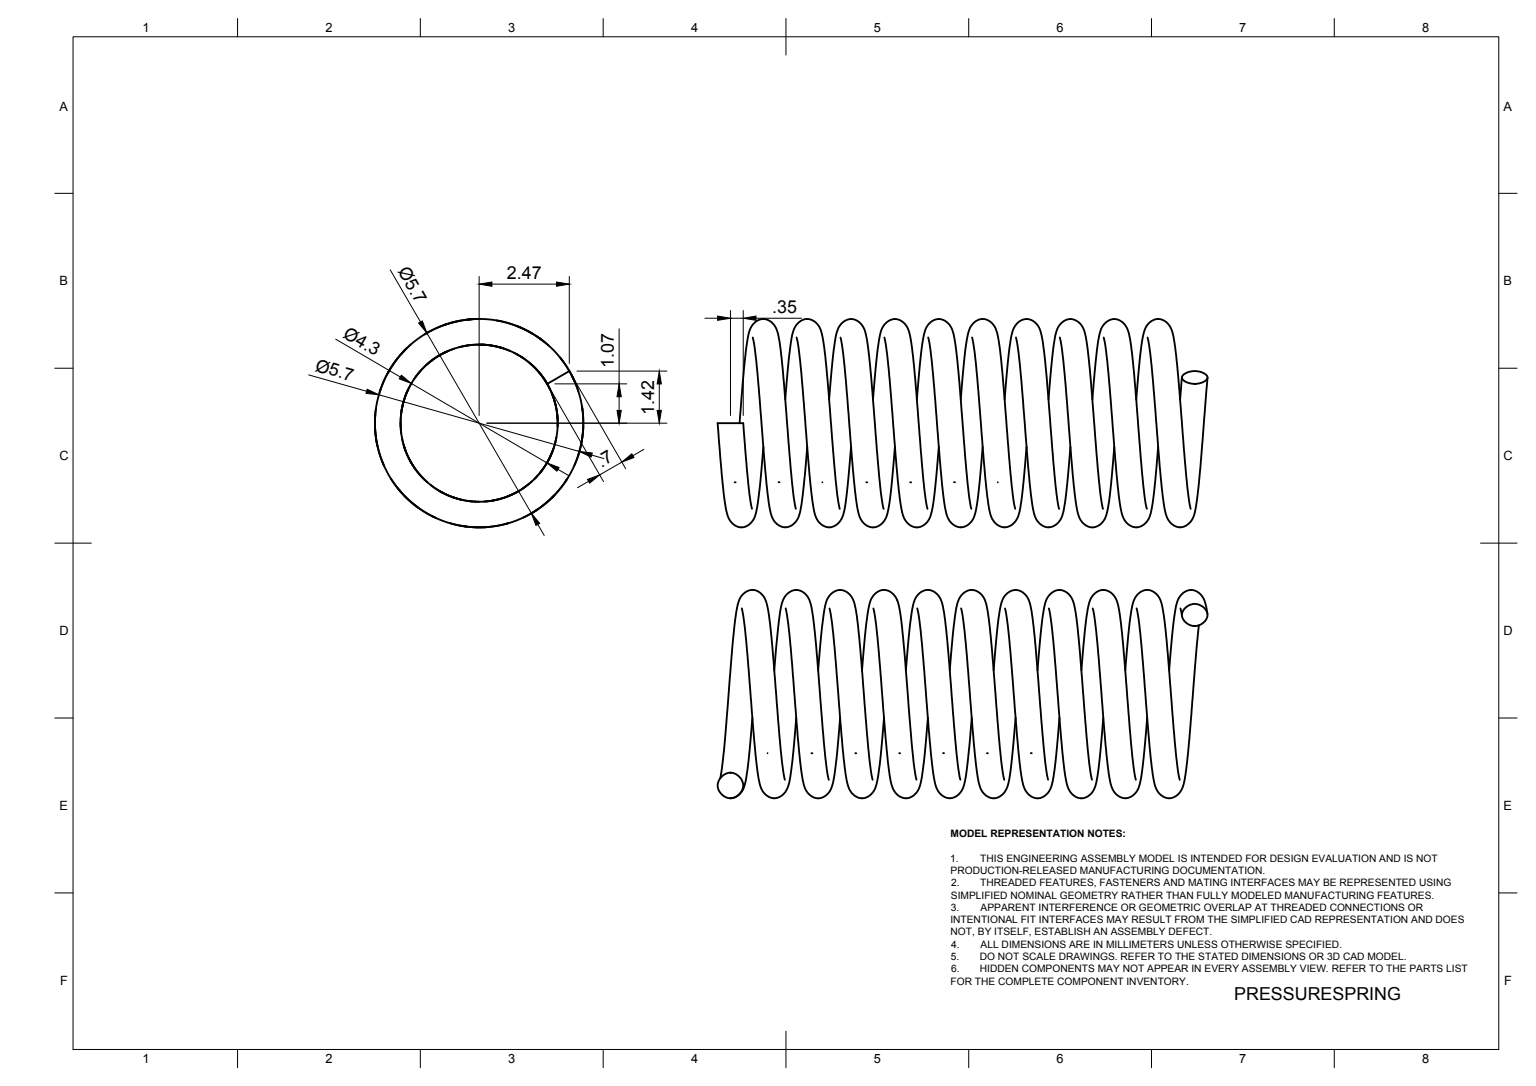
ISO-10303-21;
HEADER;
/* Generated by software containing ST-Developer
 * from STEP Tools, Inc. (www.steptools.com) 
 */

FILE_DESCRIPTION(
/* description */ (''),
/* implementation_level */ '2;1');

FILE_NAME(
/* name */ 'PRESSURESPRING.step',
/* time_stamp */ '2026-10-06T01:16:10-07:00',
/* author */ (''),
/* organization */ (''),
/* preprocessor_version */ 'ST-DEVELOPER v20.2',
/* originating_system */ 'Autodesk Translation Framework v15.15.0.0',
/* authorisation */ '');

FILE_SCHEMA (('AUTOMOTIVE_DESIGN { 1 0 10303 214 3 1 1 }'));
ENDSEC;

DATA;
#10=MECHANICAL_DESIGN_GEOMETRIC_PRESENTATION_REPRESENTATION('',(#319),#17113);
#11=B_SPLINE_SURFACE_WITH_KNOTS('',3,3,((#11570,#11571,#11572,#11573,#11574,
#11575,#11576,#11577,#11578,#11579,#11580,#11581,#11582,#11583,#11584,#11585,
#11586,#11587,#11588,#11589,#11590,#11591,#11592,#11593,#11594,#11595,#11596,
#11597,#11598,#11599,#11600,#11601,#11602,#11603,#11604),(#11605,#11606,
#11607,#11608,#11609,#11610,#11611,#11612,#11613,#11614,#11615,#11616,#11617,
#11618,#11619,#11620,#11621,#11622,#11623,#11624,#11625,#11626,#11627,#11628,
#11629,#11630,#11631,#11632,#11633,#11634,#11635,#11636,#11637,#11638,#11639),
(#11640,#11641,#11642,#11643,#11644,#11645,#11646,#11647,#11648,#11649,
#11650,#11651,#11652,#11653,#11654,#11655,#11656,#11657,#11658,#11659,#11660,
#11661,#11662,#11663,#11664,#11665,#11666,#11667,#11668,#11669,#11670,#11671,
#11672,#11673,#11674),(#11675,#11676,#11677,#11678,#11679,#11680,#11681,
#11682,#11683,#11684,#11685,#11686,#11687,#11688,#11689,#11690,#11691,#11692,
#11693,#11694,#11695,#11696,#11697,#11698,#11699,#11700,#11701,#11702,#11703,
#11704,#11705,#11706,#11707,#11708,#11709),(#11710,#11711,#11712,#11713,
#11714,#11715,#11716,#11717,#11718,#11719,#11720,#11721,#11722,#11723,#11724,
#11725,#11726,#11727,#11728,#11729,#11730,#11731,#11732,#11733,#11734,#11735,
#11736,#11737,#11738,#11739,#11740,#11741,#11742,#11743,#11744),(#11745,
#11746,#11747,#11748,#11749,#11750,#11751,#11752,#11753,#11754,#11755,#11756,
#11757,#11758,#11759,#11760,#11761,#11762,#11763,#11764,#11765,#11766,#11767,
#11768,#11769,#11770,#11771,#11772,#11773,#11774,#11775,#11776,#11777,#11778,
#11779),(#11780,#11781,#11782,#11783,#11784,#11785,#11786,#11787,#11788,
#11789,#11790,#11791,#11792,#11793,#11794,#11795,#11796,#11797,#11798,#11799,
#11800,#11801,#11802,#11803,#11804,#11805,#11806,#11807,#11808,#11809,#11810,
#11811,#11812,#11813,#11814),(#11815,#11816,#11817,#11818,#11819,#11820,
#11821,#11822,#11823,#11824,#11825,#11826,#11827,#11828,#11829,#11830,#11831,
#11832,#11833,#11834,#11835,#11836,#11837,#11838,#11839,#11840,#11841,#11842,
#11843,#11844,#11845,#11846,#11847,#11848,#11849),(#11850,#11851,#11852,
#11853,#11854,#11855,#11856,#11857,#11858,#11859,#11860,#11861,#11862,#11863,
#11864,#11865,#11866,#11867,#11868,#11869,#11870,#11871,#11872,#11873,#11874,
#11875,#11876,#11877,#11878,#11879,#11880,#11881,#11882,#11883,#11884),
(#11885,#11886,#11887,#11888,#11889,#11890,#11891,#11892,#11893,#11894,
#11895,#11896,#11897,#11898,#11899,#11900,#11901,#11902,#11903,#11904,#11905,
#11906,#11907,#11908,#11909,#11910,#11911,#11912,#11913,#11914,#11915,#11916,
#11917,#11918,#11919)),.UNSPECIFIED.,.F.,.F.,.F.,(4,1,1,1,1,1,1,4),(4,1,
1,1,1,1,1,1,1,1,1,1,1,1,1,1,1,1,1,1,1,1,1,1,1,1,1,1,1,1,1,1,4),(-0.05714514294858,
0.,0.125,0.25,0.3267862857371,0.4035725714743,0.4803588572114,0.5571451429486),
(-0.02,0.0125,0.045,0.0775,0.11,0.1425,0.175,0.2075,0.24,0.2725,0.305,0.3375,
0.37,0.4025,0.435,0.4675,0.5,0.5325,0.565,0.5975,0.63,0.6625,0.695,0.7275,
0.76,0.7925,0.825,0.8575,0.89,0.9225,0.955,0.9875,1.02),.UNSPECIFIED.);
#12=B_SPLINE_SURFACE_WITH_KNOTS('',3,3,((#13047,#13048,#13049,#13050,#13051,
#13052,#13053,#13054,#13055,#13056,#13057,#13058,#13059,#13060,#13061,#13062,
#13063,#13064,#13065,#13066,#13067,#13068,#13069,#13070,#13071,#13072,#13073,
#13074,#13075,#13076,#13077,#13078,#13079,#13080,#13081),(#13082,#13083,
#13084,#13085,#13086,#13087,#13088,#13089,#13090,#13091,#13092,#13093,#13094,
#13095,#13096,#13097,#13098,#13099,#13100,#13101,#13102,#13103,#13104,#13105,
#13106,#13107,#13108,#13109,#13110,#13111,#13112,#13113,#13114,#13115,#13116),
(#13117,#13118,#13119,#13120,#13121,#13122,#13123,#13124,#13125,#13126,
#13127,#13128,#13129,#13130,#13131,#13132,#13133,#13134,#13135,#13136,#13137,
#13138,#13139,#13140,#13141,#13142,#13143,#13144,#13145,#13146,#13147,#13148,
#13149,#13150,#13151),(#13152,#13153,#13154,#13155,#13156,#13157,#13158,
#13159,#13160,#13161,#13162,#13163,#13164,#13165,#13166,#13167,#13168,#13169,
#13170,#13171,#13172,#13173,#13174,#13175,#13176,#13177,#13178,#13179,#13180,
#13181,#13182,#13183,#13184,#13185,#13186),(#13187,#13188,#13189,#13190,
#13191,#13192,#13193,#13194,#13195,#13196,#13197,#13198,#13199,#13200,#13201,
#13202,#13203,#13204,#13205,#13206,#13207,#13208,#13209,#13210,#13211,#13212,
#13213,#13214,#13215,#13216,#13217,#13218,#13219,#13220,#13221),(#13222,
#13223,#13224,#13225,#13226,#13227,#13228,#13229,#13230,#13231,#13232,#13233,
#13234,#13235,#13236,#13237,#13238,#13239,#13240,#13241,#13242,#13243,#13244,
#13245,#13246,#13247,#13248,#13249,#13250,#13251,#13252,#13253,#13254,#13255,
#13256),(#13257,#13258,#13259,#13260,#13261,#13262,#13263,#13264,#13265,
#13266,#13267,#13268,#13269,#13270,#13271,#13272,#13273,#13274,#13275,#13276,
#13277,#13278,#13279,#13280,#13281,#13282,#13283,#13284,#13285,#13286,#13287,
#13288,#13289,#13290,#13291)),.UNSPECIFIED.,.F.,.F.,.F.,(4,1,1,1,4),(4,
1,1,1,1,1,1,1,1,1,1,1,1,1,1,1,1,1,1,1,1,1,1,1,1,1,1,1,1,1,1,1,4),(0.4428548570514,
0.5,0.75,1.,1.057145142949),(-0.02,0.0125,0.045,0.0775,0.11,0.1425,0.175,
0.2075,0.24,0.2725,0.305,0.3375,0.37,0.4025,0.435,0.4675,0.5,0.5325,0.565,
0.5975,0.63,0.6625,0.695,0.7275,0.76,0.7925,0.825,0.8575,0.89,0.9225,0.955,
0.9875,1.02),.UNSPECIFIED.);
#13=B_SPLINE_SURFACE_WITH_KNOTS('',3,3,((#13335,#13336,#13337,#13338,#13339,
#13340,#13341,#13342,#13343,#13344,#13345,#13346,#13347,#13348,#13349,#13350,
#13351,#13352,#13353,#13354,#13355,#13356,#13357,#13358,#13359,#13360,#13361,
#13362,#13363,#13364,#13365,#13366,#13367,#13368,#13369),(#13370,#13371,
#13372,#13373,#13374,#13375,#13376,#13377,#13378,#13379,#13380,#13381,#13382,
#13383,#13384,#13385,#13386,#13387,#13388,#13389,#13390,#13391,#13392,#13393,
#13394,#13395,#13396,#13397,#13398,#13399,#13400,#13401,#13402,#13403,#13404),
(#13405,#13406,#13407,#13408,#13409,#13410,#13411,#13412,#13413,#13414,
#13415,#13416,#13417,#13418,#13419,#13420,#13421,#13422,#13423,#13424,#13425,
#13426,#13427,#13428,#13429,#13430,#13431,#13432,#13433,#13434,#13435,#13436,
#13437,#13438,#13439),(#13440,#13441,#13442,#13443,#13444,#13445,#13446,
#13447,#13448,#13449,#13450,#13451,#13452,#13453,#13454,#13455,#13456,#13457,
#13458,#13459,#13460,#13461,#13462,#13463,#13464,#13465,#13466,#13467,#13468,
#13469,#13470,#13471,#13472,#13473,#13474),(#13475,#13476,#13477,#13478,
#13479,#13480,#13481,#13482,#13483,#13484,#13485,#13486,#13487,#13488,#13489,
#13490,#13491,#13492,#13493,#13494,#13495,#13496,#13497,#13498,#13499,#13500,
#13501,#13502,#13503,#13504,#13505,#13506,#13507,#13508,#13509),(#13510,
#13511,#13512,#13513,#13514,#13515,#13516,#13517,#13518,#13519,#13520,#13521,
#13522,#13523,#13524,#13525,#13526,#13527,#13528,#13529,#13530,#13531,#13532,
#13533,#13534,#13535,#13536,#13537,#13538,#13539,#13540,#13541,#13542,#13543,
#13544),(#13545,#13546,#13547,#13548,#13549,#13550,#13551,#13552,#13553,
#13554,#13555,#13556,#13557,#13558,#13559,#13560,#13561,#13562,#13563,#13564,
#13565,#13566,#13567,#13568,#13569,#13570,#13571,#13572,#13573,#13574,#13575,
#13576,#13577,#13578,#13579)),.UNSPECIFIED.,.F.,.F.,.F.,(4,1,1,1,4),(4,
1,1,1,1,1,1,1,1,1,1,1,1,1,1,1,1,1,1,1,1,1,1,1,1,1,1,1,1,1,1,1,4),(0.4428548570514,
0.5,0.75,1.,1.057145142949),(-0.02,0.0125,0.045,0.0775,0.11,0.1425,0.175,
0.2075,0.24,0.2725,0.305,0.3375,0.37,0.4025,0.435,0.4675,0.5,0.5325,0.565,
0.5975,0.63,0.6625,0.695,0.7275,0.76,0.7925,0.825,0.8575,0.89,0.9225,0.955,
0.9875,1.02),.UNSPECIFIED.);
#14=B_SPLINE_SURFACE_WITH_KNOTS('',3,3,((#14695,#14696,#14697,#14698,#14699,
#14700,#14701,#14702,#14703,#14704,#14705,#14706,#14707,#14708,#14709,#14710,
#14711,#14712,#14713,#14714,#14715,#14716,#14717,#14718,#14719,#14720,#14721,
#14722,#14723,#14724,#14725,#14726,#14727,#14728,#14729),(#14730,#14731,
#14732,#14733,#14734,#14735,#14736,#14737,#14738,#14739,#14740,#14741,#14742,
#14743,#14744,#14745,#14746,#14747,#14748,#14749,#14750,#14751,#14752,#14753,
#14754,#14755,#14756,#14757,#14758,#14759,#14760,#14761,#14762,#14763,#14764),
(#14765,#14766,#14767,#14768,#14769,#14770,#14771,#14772,#14773,#14774,
#14775,#14776,#14777,#14778,#14779,#14780,#14781,#14782,#14783,#14784,#14785,
#14786,#14787,#14788,#14789,#14790,#14791,#14792,#14793,#14794,#14795,#14796,
#14797,#14798,#14799),(#14800,#14801,#14802,#14803,#14804,#14805,#14806,
#14807,#14808,#14809,#14810,#14811,#14812,#14813,#14814,#14815,#14816,#14817,
#14818,#14819,#14820,#14821,#14822,#14823,#14824,#14825,#14826,#14827,#14828,
#14829,#14830,#14831,#14832,#14833,#14834),(#14835,#14836,#14837,#14838,
#14839,#14840,#14841,#14842,#14843,#14844,#14845,#14846,#14847,#14848,#14849,
#14850,#14851,#14852,#14853,#14854,#14855,#14856,#14857,#14858,#14859,#14860,
#14861,#14862,#14863,#14864,#14865,#14866,#14867,#14868,#14869),(#14870,
#14871,#14872,#14873,#14874,#14875,#14876,#14877,#14878,#14879,#14880,#14881,
#14882,#14883,#14884,#14885,#14886,#14887,#14888,#14889,#14890,#14891,#14892,
#14893,#14894,#14895,#14896,#14897,#14898,#14899,#14900,#14901,#14902,#14903,
#14904),(#14905,#14906,#14907,#14908,#14909,#14910,#14911,#14912,#14913,
#14914,#14915,#14916,#14917,#14918,#14919,#14920,#14921,#14922,#14923,#14924,
#14925,#14926,#14927,#14928,#14929,#14930,#14931,#14932,#14933,#14934,#14935,
#14936,#14937,#14938,#14939),(#14940,#14941,#14942,#14943,#14944,#14945,
#14946,#14947,#14948,#14949,#14950,#14951,#14952,#14953,#14954,#14955,#14956,
#14957,#14958,#14959,#14960,#14961,#14962,#14963,#14964,#14965,#14966,#14967,
#14968,#14969,#14970,#14971,#14972,#14973,#14974),(#14975,#14976,#14977,
#14978,#14979,#14980,#14981,#14982,#14983,#14984,#14985,#14986,#14987,#14988,
#14989,#14990,#14991,#14992,#14993,#14994,#14995,#14996,#14997,#14998,#14999,
#15000,#15001,#15002,#15003,#15004,#15005,#15006,#15007,#15008,#15009),
(#15010,#15011,#15012,#15013,#15014,#15015,#15016,#15017,#15018,#15019,
#15020,#15021,#15022,#15023,#15024,#15025,#15026,#15027,#15028,#15029,#15030,
#15031,#15032,#15033,#15034,#15035,#15036,#15037,#15038,#15039,#15040,#15041,
#15042,#15043,#15044)),.UNSPECIFIED.,.F.,.F.,.F.,(4,1,1,1,1,1,1,4),(4,1,
1,1,1,1,1,1,1,1,1,1,1,1,1,1,1,1,1,1,1,1,1,1,1,1,1,1,1,1,1,1,4),(-0.05714514294857,
0.,0.125,0.25,0.3267862857371,0.4035725714743,0.4803588572114,0.5571451429486),
(-0.02,0.0125,0.045,0.0775,0.11,0.1425,0.175,0.2075,0.24,0.2725,0.305,0.3375,
0.37,0.4025,0.435,0.4675,0.5,0.5325,0.565,0.5975,0.63,0.6625,0.695,0.7275,
0.76,0.7925,0.825,0.8575,0.89,0.9225,0.955,0.9875,1.02),.UNSPECIFIED.);
#15=B_SPLINE_SURFACE_WITH_KNOTS('',3,3,((#15100,#15101,#15102,#15103,#15104,
#15105,#15106,#15107,#15108,#15109,#15110,#15111,#15112,#15113,#15114,#15115,
#15116,#15117,#15118,#15119,#15120,#15121,#15122,#15123,#15124,#15125,#15126,
#15127,#15128,#15129,#15130,#15131,#15132,#15133,#15134),(#15135,#15136,
#15137,#15138,#15139,#15140,#15141,#15142,#15143,#15144,#15145,#15146,#15147,
#15148,#15149,#15150,#15151,#15152,#15153,#15154,#15155,#15156,#15157,#15158,
#15159,#15160,#15161,#15162,#15163,#15164,#15165,#15166,#15167,#15168,#15169),
(#15170,#15171,#15172,#15173,#15174,#15175,#15176,#15177,#15178,#15179,
#15180,#15181,#15182,#15183,#15184,#15185,#15186,#15187,#15188,#15189,#15190,
#15191,#15192,#15193,#15194,#15195,#15196,#15197,#15198,#15199,#15200,#15201,
#15202,#15203,#15204),(#15205,#15206,#15207,#15208,#15209,#15210,#15211,
#15212,#15213,#15214,#15215,#15216,#15217,#15218,#15219,#15220,#15221,#15222,
#15223,#15224,#15225,#15226,#15227,#15228,#15229,#15230,#15231,#15232,#15233,
#15234,#15235,#15236,#15237,#15238,#15239),(#15240,#15241,#15242,#15243,
#15244,#15245,#15246,#15247,#15248,#15249,#15250,#15251,#15252,#15253,#15254,
#15255,#15256,#15257,#15258,#15259,#15260,#15261,#15262,#15263,#15264,#15265,
#15266,#15267,#15268,#15269,#15270,#15271,#15272,#15273,#15274),(#15275,
#15276,#15277,#15278,#15279,#15280,#15281,#15282,#15283,#15284,#15285,#15286,
#15287,#15288,#15289,#15290,#15291,#15292,#15293,#15294,#15295,#15296,#15297,
#15298,#15299,#15300,#15301,#15302,#15303,#15304,#15305,#15306,#15307,#15308,
#15309),(#15310,#15311,#15312,#15313,#15314,#15315,#15316,#15317,#15318,
#15319,#15320,#15321,#15322,#15323,#15324,#15325,#15326,#15327,#15328,#15329,
#15330,#15331,#15332,#15333,#15334,#15335,#15336,#15337,#15338,#15339,#15340,
#15341,#15342,#15343,#15344)),.UNSPECIFIED.,.F.,.F.,.F.,(4,1,1,1,4),(4,
1,1,1,1,1,1,1,1,1,1,1,1,1,1,1,1,1,1,1,1,1,1,1,1,1,1,1,1,1,1,1,4),(-0.05714514294858,
0.,0.25,0.5,0.5571451429486),(-0.02,0.0125,0.045,0.0775,0.11,0.1425,0.175,
0.2075,0.24,0.2725,0.305,0.3375,0.37,0.4025,0.435,0.4675,0.5,0.5325,0.565,
0.5975,0.63,0.6625,0.695,0.7275,0.76,0.7925,0.825,0.8575,0.89,0.9225,0.955,
0.9875,1.02),.UNSPECIFIED.);
#16=B_SPLINE_SURFACE_WITH_KNOTS('',3,3,((#16439,#16440,#16441,#16442,#16443,
#16444,#16445,#16446,#16447,#16448,#16449,#16450,#16451,#16452,#16453,#16454,
#16455,#16456,#16457,#16458,#16459,#16460,#16461,#16462,#16463,#16464,#16465,
#16466,#16467,#16468,#16469,#16470,#16471,#16472,#16473),(#16474,#16475,
#16476,#16477,#16478,#16479,#16480,#16481,#16482,#16483,#16484,#16485,#16486,
#16487,#16488,#16489,#16490,#16491,#16492,#16493,#16494,#16495,#16496,#16497,
#16498,#16499,#16500,#16501,#16502,#16503,#16504,#16505,#16506,#16507,#16508),
(#16509,#16510,#16511,#16512,#16513,#16514,#16515,#16516,#16517,#16518,
#16519,#16520,#16521,#16522,#16523,#16524,#16525,#16526,#16527,#16528,#16529,
#16530,#16531,#16532,#16533,#16534,#16535,#16536,#16537,#16538,#16539,#16540,
#16541,#16542,#16543),(#16544,#16545,#16546,#16547,#16548,#16549,#16550,
#16551,#16552,#16553,#16554,#16555,#16556,#16557,#16558,#16559,#16560,#16561,
#16562,#16563,#16564,#16565,#16566,#16567,#16568,#16569,#16570,#16571,#16572,
#16573,#16574,#16575,#16576,#16577,#16578),(#16579,#16580,#16581,#16582,
#16583,#16584,#16585,#16586,#16587,#16588,#16589,#16590,#16591,#16592,#16593,
#16594,#16595,#16596,#16597,#16598,#16599,#16600,#16601,#16602,#16603,#16604,
#16605,#16606,#16607,#16608,#16609,#16610,#16611,#16612,#16613),(#16614,
#16615,#16616,#16617,#16618,#16619,#16620,#16621,#16622,#16623,#16624,#16625,
#16626,#16627,#16628,#16629,#16630,#16631,#16632,#16633,#16634,#16635,#16636,
#16637,#16638,#16639,#16640,#16641,#16642,#16643,#16644,#16645,#16646,#16647,
#16648),(#16649,#16650,#16651,#16652,#16653,#16654,#16655,#16656,#16657,
#16658,#16659,#16660,#16661,#16662,#16663,#16664,#16665,#16666,#16667,#16668,
#16669,#16670,#16671,#16672,#16673,#16674,#16675,#16676,#16677,#16678,#16679,
#16680,#16681,#16682,#16683)),.UNSPECIFIED.,.F.,.F.,.F.,(4,1,1,1,4),(4,
1,1,1,1,1,1,1,1,1,1,1,1,1,1,1,1,1,1,1,1,1,1,1,1,1,1,1,1,1,1,1,4),(0.4428548570514,
0.5,0.75,1.,1.057145142949),(-0.02,0.0125,0.045,0.0775,0.11,0.1425,0.175,
0.2075,0.24,0.2725,0.305,0.3375,0.37,0.4025,0.435,0.4675,0.5,0.5325,0.565,
0.5975,0.63,0.6625,0.695,0.7275,0.76,0.7925,0.825,0.8575,0.89,0.9225,0.955,
0.9875,1.02),.UNSPECIFIED.);
#203=B_SPLINE_CURVE_WITH_KNOTS('',3,(#11526,#11527,#11528,#11529,#11530,
#11531,#11532,#11533,#11534,#11535,#11536,#11537,#11538,#11539,#11540,#11541,
#11542,#11543,#11544,#11545,#11546,#11547),.UNSPECIFIED.,.F.,.F.,(4,2,2,
2,2,2,2,2,2,2,4),(-0.102916914552731,-0.0960165368188152,-0.0889835057043814,
-0.0739989051443188,-0.0615887125232106,-0.0518493032905911,-0.0421259736973909,
-0.0296860378067567,-0.0142968246061035,-0.00712380381615376,-1.60735926204118E-5),
 .UNSPECIFIED.);
#204=B_SPLINE_CURVE_WITH_KNOTS('',3,(#11548,#11549,#11550,#11551,#11552,
#11553,#11554,#11555,#11556,#11557,#11558,#11559,#11560,#11561,#11562,#11563,
#11564,#11565,#11566,#11567,#11568,#11569),.UNSPECIFIED.,.F.,.F.,(4,2,2,
2,2,2,2,2,2,2,4),(-0.10788302753294,-0.100819295498672,-0.0936081097542318,
-0.077747080264816,-0.0645335298256269,-0.0542154745376808,-0.0438805066497465,
-0.0307065427009455,-0.0148008794241195,-0.00733029393624065,-1.25860813603491E-6),
 .UNSPECIFIED.);
#205=B_SPLINE_CURVE_WITH_KNOTS('',3,(#11921,#11922,#11923,#11924,#11925,
#11926,#11927,#11928,#11929,#11930,#11931,#11932,#11933,#11934,#11935,#11936,
#11937,#11938,#11939,#11940,#11941,#11942,#11943,#11944,#11945,#11946,#11947,
#11948,#11949,#11950,#11951,#11952,#11953,#11954,#11955,#11956,#11957,#11958,
#11959,#11960,#11961,#11962,#11963,#11964,#11965,#11966,#11967,#11968,#11969,
#11970,#11971,#11972,#11973,#11974,#11975,#11976,#11977,#11978,#11979,#11980,
#11981,#11982,#11983,#11984,#11985,#11986,#11987,#11988,#11989,#11990,#11991,
#11992,#11993,#11994,#11995,#11996,#11997,#11998,#11999,#12000,#12001,#12002,
#12003,#12004,#12005,#12006,#12007,#12008,#12009,#12010,#12011,#12012,#12013,
#12014,#12015,#12016,#12017,#12018,#12019,#12020,#12021,#12022,#12023,#12024,
#12025,#12026,#12027,#12028,#12029,#12030,#12031,#12032,#12033,#12034,#12035,
#12036,#12037,#12038,#12039,#12040,#12041,#12042,#12043,#12044,#12045,#12046,
#12047,#12048,#12049,#12050,#12051,#12052,#12053,#12054,#12055,#12056,#12057,
#12058,#12059,#12060,#12061,#12062,#12063,#12064,#12065,#12066,#12067,#12068,
#12069,#12070,#12071,#12072,#12073,#12074,#12075,#12076,#12077,#12078,#12079,
#12080,#12081,#12082,#12083,#12084,#12085,#12086,#12087,#12088,#12089,#12090,
#12091,#12092,#12093,#12094,#12095,#12096,#12097,#12098,#12099,#12100,#12101,
#12102,#12103,#12104,#12105,#12106,#12107,#12108,#12109,#12110,#12111,#12112,
#12113,#12114,#12115,#12116,#12117,#12118,#12119,#12120,#12121,#12122,#12123,
#12124,#12125,#12126,#12127,#12128,#12129,#12130,#12131,#12132,#12133,#12134,
#12135,#12136,#12137,#12138,#12139,#12140,#12141,#12142,#12143,#12144,#12145,
#12146,#12147,#12148,#12149,#12150,#12151,#12152,#12153,#12154,#12155,#12156,
#12157,#12158,#12159,#12160,#12161,#12162,#12163,#12164,#12165,#12166,#12167,
#12168,#12169,#12170,#12171,#12172,#12173,#12174,#12175,#12176,#12177,#12178,
#12179,#12180,#12181,#12182,#12183,#12184,#12185,#12186,#12187,#12188,#12189,
#12190,#12191,#12192,#12193,#12194,#12195,#12196,#12197,#12198,#12199,#12200,
#12201,#12202,#12203,#12204,#12205,#12206,#12207,#12208,#12209,#12210,#12211,
#12212,#12213,#12214,#12215,#12216,#12217,#12218,#12219,#12220,#12221,#12222,
#12223,#12224,#12225,#12226,#12227,#12228,#12229,#12230,#12231,#12232,#12233,
#12234,#12235,#12236,#12237,#12238,#12239,#12240,#12241,#12242,#12243,#12244,
#12245,#12246,#12247,#12248,#12249,#12250,#12251,#12252,#12253,#12254,#12255,
#12256,#12257,#12258,#12259,#12260,#12261,#12262,#12263,#12264,#12265,#12266,
#12267,#12268,#12269,#12270,#12271,#12272,#12273,#12274,#12275,#12276,#12277,
#12278,#12279,#12280,#12281,#12282,#12283,#12284,#12285,#12286,#12287,#12288,
#12289,#12290,#12291,#12292,#12293,#12294,#12295,#12296,#12297,#12298,#12299,
#12300,#12301,#12302,#12303,#12304,#12305,#12306,#12307,#12308,#12309,#12310,
#12311,#12312,#12313,#12314,#12315,#12316,#12317,#12318,#12319,#12320,#12321,
#12322,#12323,#12324,#12325,#12326,#12327,#12328,#12329,#12330,#12331,#12332,
#12333,#12334,#12335,#12336,#12337,#12338,#12339,#12340,#12341,#12342,#12343,
#12344,#12345,#12346,#12347,#12348,#12349,#12350,#12351,#12352,#12353,#12354,
#12355,#12356,#12357,#12358,#12359,#12360,#12361,#12362,#12363,#12364,#12365,
#12366,#12367,#12368,#12369,#12370,#12371,#12372,#12373,#12374,#12375,#12376,
#12377,#12378,#12379,#12380,#12381,#12382,#12383,#12384,#12385,#12386,#12387,
#12388,#12389,#12390,#12391,#12392,#12393,#12394,#12395,#12396,#12397,#12398,
#12399,#12400,#12401,#12402,#12403,#12404,#12405,#12406,#12407,#12408,#12409,
#12410,#12411,#12412,#12413,#12414,#12415,#12416,#12417,#12418,#12419,#12420,
#12421,#12422,#12423,#12424,#12425,#12426,#12427,#12428,#12429,#12430,#12431,
#12432,#12433,#12434,#12435,#12436,#12437,#12438,#12439,#12440,#12441,#12442,
#12443,#12444,#12445,#12446,#12447,#12448,#12449,#12450,#12451,#12452,#12453,
#12454,#12455,#12456,#12457,#12458,#12459,#12460,#12461,#12462,#12463,#12464,
#12465,#12466,#12467,#12468,#12469,#12470,#12471,#12472,#12473),
 .UNSPECIFIED.,.F.,.F.,(4,3,3,3,3,3,3,3,3,3,3,3,3,3,3,3,3,3,3,3,3,3,3,3,
3,3,3,3,3,3,3,3,3,3,3,3,3,3,3,3,3,3,3,3,3,3,3,3,3,3,3,3,3,3,3,3,3,3,3,3,
3,3,3,3,3,3,3,3,3,3,3,3,3,3,3,3,3,3,3,3,3,3,3,3,3,3,3,3,3,3,3,3,3,3,3,3,
3,3,3,3,3,3,3,3,3,3,3,3,3,3,3,3,3,3,3,3,3,3,3,3,3,3,3,3,3,3,3,3,3,3,3,3,
3,3,3,3,3,3,3,3,3,3,3,3,3,3,3,3,3,3,3,3,3,3,3,3,3,3,3,3,3,3,3,3,3,3,3,3,
3,3,3,3,3,3,3,3,3,3,3,3,3,3,3,3,4),(0.,0.00625925877618659,0.012498777633829,
0.01694915254237,0.0234628389430874,0.0301365197565823,0.03389830508475,
0.0399395455000561,0.0449988746104484,0.05084745762712,0.0573237266639631,
0.0638987543535039,0.06779661016949,0.0736716349306864,0.0774993881424463,
0.0833663385077181,0.08474576271186,0.091167331299509,0.097628739000386,
0.1016949152542,0.107513390502625,0.110000096381761,0.115819871711873,0.1186440677966,
0.12510195465327,0.131545205429102,0.135593220339,0.141479707111754,0.142500758971052,
0.148398207638992,0.1525423728814,0.159137176794001,0.165656536879295,0.1694915254237,
0.175001153770124,0.181104985312333,0.1864406779661,0.193291692194109,0.199994170967044,
0.2033898305085,0.207501144893393,0.213996704784992,0.2203389830508,0.227648989561867,
0.234707372019173,0.2372881355932,0.240000783824304,0.247222805643196,0.2542372881356,
0.2627118644068,0.270472303966788,0.271186440678,0.272500297957407,0.281244760606251,
0.2881355932203,0.297798413321956,0.304999991245754,0.3050847457627,0.314508174872632,
0.3220338983051,0.330512021731323,0.337499649903537,0.3389830508475,0.346615949971345,
0.354646702577775,0.3559322033898,0.363033438865616,0.369999163432914,0.3728813559322,
0.37985332543126,0.387078943207013,0.3898305084746,0.396262716777247,0.402498837141279,
0.4067796610169,0.413421019419821,0.420230556868151,0.4237288135593,0.429797841794845,
0.434998879663644,0.4406779661017,0.447154148986824,0.453734297968348,0.4576271186441,
0.46350827908289,0.467499317471382,0.47337093009509,0.4745762711864,0.48099518354306,
0.487461530539164,0.4915254237288,0.497345526991414,0.500000003734255,0.505820187494862,
0.5084745762712,0.514924727843856,0.521366864166133,0.5254237288136,0.531295850595029,
0.532500689595544,0.538382527082556,0.5423728813559,0.54894525402918,0.555450031435636,
0.5593220338983,0.565001126342026,0.571071570720213,0.5762711864407,0.583082695457437,
0.589755631698227,0.5932203389831,0.597501167527674,0.603935922491351,0.6101694915254,
0.617407999264796,0.624410071113853,0.6271186440678,0.630000840110392,0.637106843597801,
0.6440677966102,0.65254237288135,0.660180609988071,0.6610169491525,0.662500353088126,
0.670988906543055,0.6779661016949,0.687400217121739,0.6949152542373,0.695000011705008,
0.704653651272696,0.7118644067797,0.720597517779026,0.727499705010129,0.728813559322,
0.736568079962082,0.744745446872398,0.7457627118644,0.752979538682311,0.759999219617496,
0.7627118644068,0.769740858446909,0.777036628437343,0.7796610169492,0.786153842810917,
0.792498859618453,0.7966101694915,0.803280942492757,0.810128713700182,0.8135593220339,
0.81966162847591,0.824998852078597,0.8305084745763,0.836998731347478,0.843600194647583,
0.8474576271186,0.853354320256163,0.85749924799678,0.863385148965961,0.864406779661,
0.870826069225487,0.877299244450954,0.8813559322034,0.887175557231592,0.889999911082328,
0.895818397253527,0.8983050847458,0.904749271770384,0.911193161122928,0.9152542372881,
0.921121621454876,0.922500619004354,0.928376243104498,0.9322033898305,0.938769848536967,
0.945274226985483,0.9491525423729,0.955001131578282,0.961043720040324,0.9661016949153,
0.972776378140019,0.979322863868025,0.9830508474576,0.987501227214033,0.993762571705349,
1.),.UNSPECIFIED.);
#206=B_SPLINE_CURVE_WITH_KNOTS('',3,(#12475,#12476,#12477,#12478,#12479,
#12480,#12481,#12482,#12483,#12484,#12485,#12486,#12487,#12488,#12489,#12490,
#12491,#12492,#12493,#12494,#12495,#12496,#12497,#12498,#12499,#12500,#12501,
#12502,#12503,#12504,#12505,#12506,#12507,#12508,#12509,#12510,#12511,#12512,
#12513,#12514,#12515,#12516,#12517,#12518,#12519,#12520,#12521,#12522,#12523,
#12524,#12525,#12526,#12527,#12528,#12529),.UNSPECIFIED.,.F.,.F.,(4,3,3,
3,3,3,3,3,3,3,3,3,3,3,3,3,3,3,4),(2.3090748468048E-7,4.45838606717901E-5,
0.103040149515435,0.193721878728962,0.25,0.251116964176227,0.330254232791472,
0.414362786406979,0.487704402387173,0.498471340022485,0.5,0.590018211493824,
0.65062380043533,0.733876213547321,0.75,0.804169141594039,0.887250644440787,
0.959806362373788,1.),.UNSPECIFIED.);
#207=B_SPLINE_CURVE_WITH_KNOTS('',3,(#12530,#12531,#12532,#12533,#12534,
#12535,#12536,#12537,#12538,#12539,#12540,#12541,#12542,#12543,#12544,#12545,
#12546,#12547,#12548,#12549,#12550,#12551,#12552,#12553,#12554,#12555,#12556,
#12557,#12558,#12559,#12560,#12561,#12562,#12563,#12564,#12565,#12566,#12567,
#12568,#12569,#12570,#12571,#12572,#12573,#12574,#12575,#12576,#12577,#12578,
#12579,#12580,#12581,#12582,#12583,#12584,#12585,#12586,#12587,#12588,#12589,
#12590,#12591,#12592,#12593,#12594,#12595,#12596,#12597,#12598,#12599,#12600,
#12601,#12602,#12603,#12604,#12605,#12606,#12607,#12608,#12609,#12610,#12611,
#12612,#12613,#12614,#12615,#12616,#12617,#12618,#12619,#12620,#12621,#12622,
#12623,#12624,#12625,#12626,#12627,#12628,#12629,#12630,#12631,#12632,#12633,
#12634,#12635,#12636,#12637,#12638,#12639,#12640,#12641,#12642,#12643,#12644,
#12645,#12646,#12647,#12648,#12649,#12650,#12651,#12652,#12653,#12654,#12655,
#12656,#12657,#12658,#12659,#12660,#12661,#12662,#12663,#12664,#12665,#12666,
#12667,#12668,#12669,#12670,#12671,#12672,#12673,#12674,#12675,#12676,#12677,
#12678,#12679,#12680,#12681,#12682,#12683,#12684,#12685,#12686,#12687,#12688,
#12689,#12690,#12691,#12692,#12693,#12694,#12695,#12696,#12697,#12698,#12699,
#12700,#12701,#12702,#12703,#12704,#12705,#12706,#12707,#12708,#12709,#12710,
#12711,#12712,#12713,#12714,#12715,#12716,#12717,#12718,#12719,#12720,#12721,
#12722,#12723,#12724,#12725,#12726,#12727,#12728,#12729,#12730,#12731,#12732,
#12733,#12734,#12735,#12736,#12737,#12738,#12739,#12740,#12741,#12742,#12743,
#12744,#12745,#12746,#12747,#12748,#12749,#12750,#12751,#12752,#12753,#12754,
#12755,#12756,#12757,#12758,#12759,#12760,#12761,#12762,#12763,#12764,#12765,
#12766,#12767,#12768,#12769,#12770,#12771,#12772,#12773,#12774,#12775,#12776,
#12777,#12778,#12779,#12780,#12781,#12782,#12783,#12784,#12785,#12786,#12787,
#12788,#12789,#12790,#12791,#12792,#12793,#12794,#12795,#12796,#12797,#12798,
#12799,#12800,#12801,#12802,#12803,#12804,#12805,#12806,#12807,#12808,#12809,
#12810,#12811,#12812,#12813,#12814,#12815,#12816,#12817,#12818,#12819,#12820,
#12821,#12822,#12823,#12824,#12825,#12826,#12827,#12828,#12829,#12830,#12831,
#12832,#12833,#12834,#12835,#12836,#12837,#12838,#12839,#12840,#12841,#12842,
#12843,#12844,#12845,#12846,#12847,#12848,#12849,#12850,#12851,#12852,#12853,
#12854,#12855,#12856,#12857,#12858,#12859,#12860,#12861,#12862,#12863,#12864,
#12865,#12866,#12867,#12868,#12869,#12870,#12871,#12872,#12873,#12874,#12875,
#12876,#12877,#12878,#12879,#12880,#12881,#12882,#12883,#12884,#12885,#12886,
#12887,#12888,#12889,#12890,#12891,#12892,#12893,#12894,#12895,#12896,#12897,
#12898,#12899,#12900,#12901,#12902,#12903,#12904,#12905,#12906,#12907,#12908,
#12909,#12910,#12911,#12912,#12913,#12914,#12915,#12916,#12917,#12918,#12919,
#12920,#12921,#12922,#12923,#12924,#12925,#12926,#12927,#12928,#12929,#12930,
#12931,#12932,#12933,#12934,#12935,#12936,#12937,#12938,#12939,#12940,#12941,
#12942,#12943,#12944,#12945,#12946,#12947,#12948,#12949,#12950,#12951,#12952,
#12953,#12954,#12955,#12956,#12957,#12958,#12959,#12960,#12961,#12962,#12963,
#12964,#12965,#12966,#12967,#12968,#12969,#12970,#12971,#12972,#12973,#12974,
#12975,#12976,#12977,#12978,#12979,#12980,#12981,#12982,#12983,#12984,#12985,
#12986,#12987,#12988,#12989,#12990,#12991,#12992,#12993,#12994,#12995,#12996,
#12997,#12998,#12999,#13000,#13001,#13002,#13003,#13004,#13005,#13006,#13007,
#13008,#13009,#13010,#13011,#13012,#13013,#13014,#13015,#13016,#13017,#13018,
#13019,#13020,#13021,#13022,#13023,#13024,#13025,#13026,#13027,#13028,#13029,
#13030,#13031,#13032,#13033,#13034,#13035,#13036,#13037,#13038,#13039,#13040,
#13041,#13042,#13043,#13044,#13045,#13046),.UNSPECIFIED.,.F.,.F.,(4,3,3,
3,3,3,3,3,3,3,3,3,3,3,3,3,3,3,3,3,3,3,3,3,3,3,3,3,3,3,3,3,3,3,3,3,3,3,3,
3,3,3,3,3,3,3,3,3,3,3,3,3,3,3,3,3,3,3,3,3,3,3,3,3,3,3,3,3,3,3,3,3,3,3,3,
3,3,3,3,3,3,3,3,3,3,3,3,3,3,3,3,3,3,3,3,3,3,3,3,3,3,3,3,3,3,3,3,3,3,3,3,
3,3,3,3,3,3,3,3,3,3,3,3,3,3,3,3,3,3,3,3,3,3,3,3,3,3,3,3,3,3,3,3,3,3,3,3,
3,3,3,3,3,3,3,3,3,3,3,3,3,3,3,3,3,3,3,3,3,3,3,3,3,4),(0.,0.00661684428018137,
0.0124983817048157,0.01818181818182,0.0250973632804601,0.0321069440395133,
0.03636363636364,0.0426727072895669,0.0450002377175405,0.0513095386321912,
0.05454545454545,0.0617456270204197,0.0688539157013956,0.07272727272727,
0.0775015374916661,0.0844748541646262,0.09090909090909,0.099999999999995,
0.108428998891845,0.1090909090909,0.110000217048989,0.12078325484281,0.1272727272727,
0.135245023027212,0.142498954904298,0.1454545454545,0.152858323610583,0.160506895105771,
0.1636363636364,0.170111029696646,0.174998755495631,0.181458997908831,0.1818181818182,
0.188790646856768,0.195802632099578,0.2,0.206382022349692,0.207500940523936,
0.213892441612431,0.2181818181818,0.225620518782517,0.232894897619836,0.2363636363636,
0.240001295617423,0.24749297412486,0.2545454545455,0.264726456123787,0.272499960749247,
0.2727272727273,0.282186815835694,0.2909090909091,0.298158858068406,0.30499857495095,
0.3090909090909,0.316250190246083,0.323581911184479,0.3272727272727,0.33362603963409,
0.337499304115395,0.343846043279279,0.3454545454545,0.352469372648584,0.359471200512104,
0.3636363636364,0.370001396088217,0.376550684913404,0.3818181818182,0.389651332870855,
0.397226018556947,0.4,0.402500854077189,0.410898586807204,0.4181818181818,
0.428299197899163,0.434999622589465,0.4363636363636,0.444446016034832,0.452935768204114,
0.4545454545455,0.461363105296409,0.467498436350891,0.4727272727273,0.479753855421816,
0.486893984305155,0.4909090909091,0.497221599841649,0.500000000005468,0.506312508953864,
0.5090909090909,0.51621847416553,0.523276761335571,0.5272727272727,0.532501563654628,
0.539319218740823,0.5454545454545,0.553958909635691,0.562058015370272,0.5636363636364,
0.565000377410551,0.575117784621314,0.5818181818182,0.590215898849764,0.597499145923507,
0.6,0.607544531271774,0.615369919544731,0.6181818181818,0.624731104355087,
0.629998603919711,0.6363636363636,0.643337807116345,0.65037226491035,0.6545454545455,
0.660892194670005,0.662500695894973,0.6688540092563,0.6727272727273,0.680054450651049,
0.687247439083709,0.6909090909091,0.695001425052158,0.702251199224186,0.7090909090909,
0.718550473994048,0.7272727272727,0.727500039250745,0.737681014960217,0.7454545454545,
0.75294621533796,0.759998704384844,0.7636363636364,0.770877063207263,0.778316868345802,
0.7818181818182,0.78820968148288,0.792499059485903,0.798881080459228,0.8,
0.806989821379187,0.813987898953542,0.8181818181818,0.8246420626511,0.825001244513147,
0.831475912696751,0.8363636363636,0.844016416669735,0.851452485846813,0.8545454545455,
0.857501045096921,0.865473353019941,0.8727272727273,0.883510301615267,0.889999782950977,
0.8909090909091,0.899338076324425,0.908253206519462,0.9090909090909,0.916064220506329,
0.922498462512828,0.9272727272727,0.934348434679549,0.941558334052561,0.9454545454545,
0.951763846001661,0.954999762293423,0.961308832885248,0.9636363636364,0.970630377326059,
0.977577339610233,0.9818181818182,0.987501618301725,0.994118465771046,1.),
 .UNSPECIFIED.);
#208=B_SPLINE_CURVE_WITH_KNOTS('',3,(#13292,#13293,#13294,#13295,#13296,
#13297,#13298,#13299,#13300,#13301,#13302,#13303,#13304,#13305,#13306,#13307,
#13308,#13309,#13310,#13311,#13312,#13313,#13314,#13315,#13316,#13317,#13318,
#13319,#13320,#13321,#13322,#13323,#13324,#13325,#13326,#13327,#13328,#13329,
#13330,#13331,#13332,#13333,#13334),.UNSPECIFIED.,.F.,.F.,(4,3,3,3,3,3,
3,3,3,3,3,3,3,3,4),(0.,0.0875545420214221,0.172845777591114,0.25,0.335847439737665,
0.429706536547853,0.5,0.501528659336918,0.577112096273498,0.657242820384804,
0.735419949981763,0.75,0.839853036636981,0.941009610342587,1.),
 .UNSPECIFIED.);
#209=B_SPLINE_CURVE_WITH_KNOTS('',3,(#13581,#13582,#13583,#13584,#13585,
#13586,#13587,#13588,#13589,#13590,#13591,#13592,#13593,#13594,#13595,#13596,
#13597,#13598,#13599,#13600,#13601,#13602,#13603,#13604,#13605,#13606,#13607,
#13608,#13609,#13610,#13611,#13612,#13613,#13614,#13615,#13616,#13617,#13618,
#13619,#13620,#13621,#13622,#13623,#13624,#13625,#13626,#13627,#13628,#13629,
#13630,#13631,#13632,#13633,#13634,#13635,#13636,#13637,#13638,#13639,#13640,
#13641,#13642,#13643,#13644,#13645,#13646,#13647,#13648,#13649,#13650,#13651,
#13652,#13653,#13654,#13655,#13656,#13657,#13658,#13659,#13660,#13661,#13662,
#13663,#13664,#13665,#13666,#13667,#13668,#13669,#13670,#13671,#13672,#13673,
#13674,#13675,#13676,#13677,#13678,#13679,#13680,#13681,#13682,#13683,#13684,
#13685,#13686,#13687,#13688,#13689,#13690,#13691,#13692,#13693,#13694,#13695,
#13696,#13697,#13698,#13699,#13700,#13701,#13702,#13703,#13704,#13705,#13706,
#13707,#13708,#13709,#13710,#13711,#13712,#13713,#13714,#13715,#13716,#13717,
#13718,#13719,#13720,#13721,#13722,#13723,#13724,#13725,#13726,#13727,#13728,
#13729,#13730,#13731,#13732,#13733,#13734,#13735,#13736,#13737,#13738,#13739,
#13740,#13741,#13742,#13743,#13744,#13745,#13746,#13747,#13748,#13749,#13750,
#13751,#13752,#13753,#13754,#13755,#13756,#13757,#13758,#13759,#13760,#13761,
#13762,#13763,#13764,#13765,#13766,#13767,#13768,#13769,#13770,#13771,#13772,
#13773,#13774,#13775,#13776,#13777,#13778,#13779,#13780,#13781,#13782,#13783,
#13784,#13785,#13786,#13787,#13788,#13789,#13790,#13791,#13792,#13793,#13794,
#13795,#13796,#13797,#13798,#13799,#13800,#13801,#13802,#13803,#13804,#13805,
#13806,#13807,#13808,#13809,#13810,#13811,#13812,#13813,#13814,#13815,#13816,
#13817,#13818,#13819,#13820,#13821,#13822,#13823,#13824,#13825,#13826,#13827,
#13828,#13829,#13830,#13831,#13832,#13833,#13834,#13835,#13836,#13837,#13838,
#13839,#13840,#13841,#13842,#13843,#13844,#13845,#13846,#13847,#13848,#13849,
#13850,#13851,#13852,#13853,#13854,#13855,#13856,#13857,#13858,#13859,#13860,
#13861,#13862,#13863,#13864,#13865,#13866,#13867,#13868,#13869,#13870,#13871,
#13872,#13873,#13874,#13875,#13876,#13877,#13878,#13879,#13880,#13881,#13882,
#13883,#13884,#13885,#13886,#13887,#13888,#13889,#13890,#13891,#13892,#13893,
#13894,#13895,#13896,#13897,#13898,#13899,#13900,#13901,#13902,#13903,#13904,
#13905,#13906,#13907,#13908,#13909,#13910,#13911,#13912,#13913,#13914,#13915,
#13916,#13917,#13918,#13919,#13920,#13921,#13922,#13923,#13924,#13925,#13926,
#13927,#13928,#13929,#13930,#13931,#13932,#13933,#13934,#13935,#13936,#13937,
#13938,#13939,#13940,#13941,#13942,#13943,#13944,#13945,#13946,#13947,#13948,
#13949,#13950,#13951,#13952,#13953,#13954,#13955,#13956,#13957,#13958,#13959,
#13960,#13961,#13962,#13963,#13964,#13965,#13966,#13967,#13968,#13969,#13970,
#13971,#13972,#13973,#13974,#13975,#13976,#13977,#13978,#13979,#13980,#13981,
#13982,#13983,#13984,#13985,#13986,#13987,#13988,#13989,#13990,#13991,#13992,
#13993,#13994,#13995,#13996,#13997,#13998,#13999,#14000,#14001,#14002,#14003,
#14004,#14005,#14006,#14007,#14008,#14009,#14010,#14011,#14012,#14013,#14014,
#14015,#14016,#14017,#14018,#14019,#14020,#14021,#14022,#14023,#14024,#14025,
#14026,#14027,#14028,#14029,#14030,#14031,#14032,#14033,#14034,#14035,#14036,
#14037,#14038,#14039,#14040,#14041,#14042,#14043,#14044,#14045,#14046,#14047,
#14048,#14049,#14050,#14051,#14052,#14053,#14054,#14055,#14056,#14057,#14058,
#14059,#14060,#14061,#14062,#14063,#14064,#14065,#14066,#14067,#14068,#14069,
#14070,#14071,#14072,#14073,#14074,#14075,#14076,#14077,#14078,#14079,#14080,
#14081,#14082,#14083,#14084,#14085,#14086,#14087,#14088,#14089,#14090,#14091,
#14092,#14093,#14094,#14095,#14096,#14097),.UNSPECIFIED.,.F.,.F.,(4,3,3,
3,3,3,3,3,3,3,3,3,3,3,3,3,3,3,3,3,3,3,3,3,3,3,3,3,3,3,3,3,3,3,3,3,3,3,3,
3,3,3,3,3,3,3,3,3,3,3,3,3,3,3,3,3,3,3,3,3,3,3,3,3,3,3,3,3,3,3,3,3,3,3,3,
3,3,3,3,3,3,3,3,3,3,3,3,3,3,3,3,3,3,3,3,3,3,3,3,3,3,3,3,3,3,3,3,3,3,3,3,
3,3,3,3,3,3,3,3,3,3,3,3,3,3,3,3,3,3,3,3,3,3,3,3,3,3,3,3,3,3,3,3,3,3,3,3,
3,3,3,3,3,3,3,3,3,3,3,3,3,3,3,3,3,3,3,3,3,3,3,3,3,4),(0.,0.00661684587302782,
0.0124983817015463,0.01818181818182,0.0250973637783485,0.0321069452291795,
0.03636363636364,0.0426727071234974,0.0450002377120509,0.0513095384439047,
0.05454545454545,0.0617456257734155,0.0688539134555847,0.07272727272727,
0.0775015374894108,0.084474851540618,0.09090909090909,0.099999999999995,
0.108428992128763,0.1090909090909,0.110000217049007,0.120783250406177,0.1272727272727,
0.135245029127456,0.14249895490368,0.1454545454545,0.152858325981983,0.160506900311987,
0.1636363636364,0.170111030760943,0.174998755491235,0.181458998931494,0.1818181818182,
0.188790646918572,0.195802632397153,0.2,0.20638202166108,0.207500940519021,
0.213892440897584,0.2181818181818,0.225620516663454,0.232894893756121,0.2363636363636,
0.240001295616291,0.247492969823263,0.2545454545455,0.264726443160001,0.272499960749249,
0.2727272727273,0.282186826709124,0.2909090909091,0.298158861584354,0.304998574949388,
0.3090909090909,0.316250191676838,0.323581914343074,0.3272727272727,0.333626040135667,
0.337499304110203,0.343846043754309,0.3454545454545,0.352469372214191,0.359471199824338,
0.3636363636364,0.37000139608426,0.376550683586942,0.3818181818182,0.389651329369765,
0.397226012189459,0.4,0.402500854076844,0.41089857897861,0.4181818181818,
0.428299211683496,0.434999622589454,0.4363636363636,0.444446021132103,0.452935779498683,
0.4545454545455,0.461363107469399,0.467498436348121,0.4727272727273,0.479753856203367,
0.486893986084007,0.4909090909091,0.497221599849583,0.50000000008049,0.506312509021862,
0.5090909090909,0.516218473166445,0.523276759559391,0.5272727272727,0.532501563651875,
0.539319216575929,0.5454545454545,0.553958903433111,0.562058004188518,0.5636363636364,
0.565000377410543,0.575117770912628,0.5818181818182,0.590215906719939,0.597499145923154,
0.6,0.607544534174367,0.615369925924941,0.6181818181818,0.624731105684524,
0.62999860391574,0.6363636363636,0.643337807374441,0.650372265605971,0.6545454545455,
0.66089219418957,0.662500695889797,0.668854008752732,0.6727272727273,0.680054448914732,
0.687247435925352,0.6909090909091,0.695001425050611,0.702251195725602,0.7090909090909,
0.7185504630727,0.7272727272727,0.72750003925074,0.737681027864929,0.7454545454545,
0.752946219661666,0.759998704383705,0.7636363636364,0.770877064964224,0.778316872209192,
0.7818181818182,0.788209682197035,0.792499059480986,0.798881081142189,0.8,
0.806989821147635,0.813987898664929,0.8181818181818,0.824642061622228,0.825001244508765,
0.831475911633545,0.8363636363636,0.844016413814636,0.85145248064292,0.8545454545455,
0.857501045096319,0.865473346951777,0.8727272727273,0.883510306083592,0.889999782950987,
0.8909090909091,0.899338083037124,0.908253221411253,0.9090909090909,0.916064223141442,
0.922498462510562,0.9272727272727,0.934348435683629,0.941558336299738,0.9454545454545,
0.951763846186177,0.954999762287945,0.961308833047529,0.9636363636364,0.970630376636409,
0.977577338426202,0.9818181818182,0.987501618298469,0.994118464170932,1.),
 .UNSPECIFIED.);
#210=B_SPLINE_CURVE_WITH_KNOTS('',3,(#14099,#14100,#14101,#14102,#14103,
#14104,#14105,#14106,#14107,#14108,#14109,#14110,#14111,#14112,#14113,#14114,
#14115,#14116,#14117,#14118,#14119,#14120,#14121,#14122,#14123,#14124,#14125,
#14126,#14127,#14128,#14129,#14130,#14131,#14132,#14133,#14134,#14135,#14136,
#14137,#14138,#14139,#14140,#14141),.UNSPECIFIED.,.F.,.F.,(4,3,3,3,3,3,
3,3,3,3,3,3,3,3,4),(0.,0.0875545420481924,0.172845777629218,0.25,0.335847439744804,
0.429706536572654,0.5,0.501528659337301,0.577112096262907,0.657242820363663,
0.735419949953638,0.75,0.839853036634623,0.941009610341032,1.),
 .UNSPECIFIED.);
#211=B_SPLINE_CURVE_WITH_KNOTS('',3,(#14142,#14143,#14144,#14145,#14146,
#14147,#14148,#14149,#14150,#14151,#14152,#14153,#14154,#14155,#14156,#14157,
#14158,#14159,#14160,#14161,#14162,#14163,#14164,#14165,#14166,#14167,#14168,
#14169,#14170,#14171,#14172,#14173,#14174,#14175,#14176,#14177,#14178,#14179,
#14180,#14181,#14182,#14183,#14184,#14185,#14186,#14187,#14188,#14189,#14190,
#14191,#14192,#14193,#14194,#14195,#14196,#14197,#14198,#14199,#14200,#14201,
#14202,#14203,#14204,#14205,#14206,#14207,#14208,#14209,#14210,#14211,#14212,
#14213,#14214,#14215,#14216,#14217,#14218,#14219,#14220,#14221,#14222,#14223,
#14224,#14225,#14226,#14227,#14228,#14229,#14230,#14231,#14232,#14233,#14234,
#14235,#14236,#14237,#14238,#14239,#14240,#14241,#14242,#14243,#14244,#14245,
#14246,#14247,#14248,#14249,#14250,#14251,#14252,#14253,#14254,#14255,#14256,
#14257,#14258,#14259,#14260,#14261,#14262,#14263,#14264,#14265,#14266,#14267,
#14268,#14269,#14270,#14271,#14272,#14273,#14274,#14275,#14276,#14277,#14278,
#14279,#14280,#14281,#14282,#14283,#14284,#14285,#14286,#14287,#14288,#14289,
#14290,#14291,#14292,#14293,#14294,#14295,#14296,#14297,#14298,#14299,#14300,
#14301,#14302,#14303,#14304,#14305,#14306,#14307,#14308,#14309,#14310,#14311,
#14312,#14313,#14314,#14315,#14316,#14317,#14318,#14319,#14320,#14321,#14322,
#14323,#14324,#14325,#14326,#14327,#14328,#14329,#14330,#14331,#14332,#14333,
#14334,#14335,#14336,#14337,#14338,#14339,#14340,#14341,#14342,#14343,#14344,
#14345,#14346,#14347,#14348,#14349,#14350,#14351,#14352,#14353,#14354,#14355,
#14356,#14357,#14358,#14359,#14360,#14361,#14362,#14363,#14364,#14365,#14366,
#14367,#14368,#14369,#14370,#14371,#14372,#14373,#14374,#14375,#14376,#14377,
#14378,#14379,#14380,#14381,#14382,#14383,#14384,#14385,#14386,#14387,#14388,
#14389,#14390,#14391,#14392,#14393,#14394,#14395,#14396,#14397,#14398,#14399,
#14400,#14401,#14402,#14403,#14404,#14405,#14406,#14407,#14408,#14409,#14410,
#14411,#14412,#14413,#14414,#14415,#14416,#14417,#14418,#14419,#14420,#14421,
#14422,#14423,#14424,#14425,#14426,#14427,#14428,#14429,#14430,#14431,#14432,
#14433,#14434,#14435,#14436,#14437,#14438,#14439,#14440,#14441,#14442,#14443,
#14444,#14445,#14446,#14447,#14448,#14449,#14450,#14451,#14452,#14453,#14454,
#14455,#14456,#14457,#14458,#14459,#14460,#14461,#14462,#14463,#14464,#14465,
#14466,#14467,#14468,#14469,#14470,#14471,#14472,#14473,#14474,#14475,#14476,
#14477,#14478,#14479,#14480,#14481,#14482,#14483,#14484,#14485,#14486,#14487,
#14488,#14489,#14490,#14491,#14492,#14493,#14494,#14495,#14496,#14497,#14498,
#14499,#14500,#14501,#14502,#14503,#14504,#14505,#14506,#14507,#14508,#14509,
#14510,#14511,#14512,#14513,#14514,#14515,#14516,#14517,#14518,#14519,#14520,
#14521,#14522,#14523,#14524,#14525,#14526,#14527,#14528,#14529,#14530,#14531,
#14532,#14533,#14534,#14535,#14536,#14537,#14538,#14539,#14540,#14541,#14542,
#14543,#14544,#14545,#14546,#14547,#14548,#14549,#14550,#14551,#14552,#14553,
#14554,#14555,#14556,#14557,#14558,#14559,#14560,#14561,#14562,#14563,#14564,
#14565,#14566,#14567,#14568,#14569,#14570,#14571,#14572,#14573,#14574,#14575,
#14576,#14577,#14578,#14579,#14580,#14581,#14582,#14583,#14584,#14585,#14586,
#14587,#14588,#14589,#14590,#14591,#14592,#14593,#14594,#14595,#14596,#14597,
#14598,#14599,#14600,#14601,#14602,#14603,#14604,#14605,#14606,#14607,#14608,
#14609,#14610,#14611,#14612,#14613,#14614,#14615,#14616,#14617,#14618,#14619,
#14620,#14621,#14622,#14623,#14624,#14625,#14626,#14627,#14628,#14629,#14630,
#14631,#14632,#14633,#14634,#14635,#14636,#14637,#14638,#14639,#14640,#14641,
#14642,#14643,#14644,#14645,#14646,#14647,#14648,#14649,#14650,#14651,#14652,
#14653,#14654,#14655,#14656,#14657,#14658,#14659,#14660,#14661,#14662,#14663,
#14664,#14665,#14666,#14667,#14668,#14669,#14670,#14671,#14672,#14673,#14674,
#14675,#14676,#14677,#14678,#14679,#14680,#14681,#14682,#14683,#14684,#14685,
#14686,#14687,#14688,#14689,#14690,#14691,#14692,#14693,#14694),
 .UNSPECIFIED.,.F.,.F.,(4,3,3,3,3,3,3,3,3,3,3,3,3,3,3,3,3,3,3,3,3,3,3,3,
3,3,3,3,3,3,3,3,3,3,3,3,3,3,3,3,3,3,3,3,3,3,3,3,3,3,3,3,3,3,3,3,3,3,3,3,
3,3,3,3,3,3,3,3,3,3,3,3,3,3,3,3,3,3,3,3,3,3,3,3,3,3,3,3,3,3,3,3,3,3,3,3,
3,3,3,3,3,3,3,3,3,3,3,3,3,3,3,3,3,3,3,3,3,3,3,3,3,3,3,3,3,3,3,3,3,3,3,3,
3,3,3,3,3,3,3,3,3,3,3,3,3,3,3,3,3,3,3,3,3,3,3,3,3,3,3,3,3,3,3,3,3,3,3,3,
3,3,3,3,3,3,3,3,3,3,3,3,3,3,3,3,4),(0.,0.00625925877606793,0.0124987776338276,
0.01694915254237,0.0234628389429566,0.0301365197563092,0.03389830508475,
0.039939545499986,0.0449988746104479,0.05084745762712,0.0573237266639023,
0.0638987543533824,0.06779661016949,0.0736716349306714,0.0774993881424457,
0.0833663385077112,0.08474576271186,0.0911673312994687,0.097628739000311,
0.1016949152542,0.107513390502593,0.110000096381758,0.115819871711832,0.1186440677966,
0.125101954653236,0.131545205429034,0.135593220339,0.141479707111713,0.142500758971051,
0.148398207639012,0.1525423728814,0.159137176793838,0.165656536878994,0.1694915254237,
0.175001153770122,0.181104985312047,0.1864406779661,0.193291692193679,0.199994170966203,
0.2033898305085,0.207501144893392,0.213996704784881,0.2203389830508,0.227648989561818,
0.2347073720192,0.2372881355932,0.240000783824308,0.247222805643388,0.2542372881356,
0.2627118644068,0.270472303966989,0.271186440678,0.272500297957408,0.28124476060672,
0.2881355932203,0.297798413322731,0.304999991245749,0.3050847457627,0.314508174872286,
0.3220338983051,0.330512021731217,0.337499649903534,0.3389830508475,0.346615949971126,
0.354646702577011,0.3559322033898,0.363033438864976,0.36999916343291,0.3728813559322,
0.379853325430446,0.387078943205471,0.3898305084746,0.396262716777213,0.402498837141285,
0.4067796610169,0.413421019420046,0.42023055686854,0.4237288135593,0.429797841794883,
0.434998879663639,0.4406779661017,0.447154148986795,0.453734297968399,0.4576271186441,
0.463508279082776,0.46749931747137,0.473370930095005,0.4745762711864,0.480995183542743,
0.487461530538509,0.4915254237288,0.497345526991346,0.500000003734252,0.505820187494761,
0.5084745762712,0.514924727844113,0.521366864166466,0.5254237288136,0.531295850594903,
0.532500689595533,0.538382527082556,0.5423728813559,0.548945254028873,0.555450031435156,
0.5593220338983,0.565001126342024,0.571071570720126,0.5762711864407,0.583082695457072,
0.589755631697393,0.5932203389831,0.597501167527672,0.60393592249075,0.6101694915254,
0.617407999264105,0.624410071112492,0.6271186440678,0.630000840110391,0.637106843597752,
0.6440677966102,0.65254237288135,0.66018060998796,0.6610169491525,0.662500353088121,
0.67098890654174,0.6779661016949,0.687400217120541,0.6949152542373,0.695000011705004,
0.704653651273056,0.7118644067797,0.720597517778143,0.727499705010129,0.728813559322,
0.736568079961608,0.744745446870372,0.7457627118644,0.752979538681499,0.759999219617496,
0.7627118644068,0.769740858446694,0.777036628436699,0.7796610169492,0.786153842811008,
0.79249885961846,0.7966101694915,0.803280942492585,0.810128713699996,0.8135593220339,
0.819661628475613,0.824998852078598,0.8305084745763,0.836998731347269,0.843600194647035,
0.8474576271186,0.853354320256033,0.857499247996783,0.863385148965559,0.864406779661,
0.870826069224946,0.877299244449807,0.8813559322034,0.887175557231284,0.88999991108234,
0.895818397253246,0.8983050847458,0.90474927177023,0.911193161122714,0.9152542372881,
0.921121621454917,0.922500619004355,0.928376243104466,0.9322033898305,0.938769848537038,
0.945274226985684,0.9491525423729,0.95500113157828,0.961043720040502,0.9661016949153,
0.972776378140131,0.97932286386849,0.9830508474576,0.987501227214035,0.993762571705703,
1.),.UNSPECIFIED.);
#212=B_SPLINE_CURVE_WITH_KNOTS('',3,(#15045,#15046,#15047,#15048,#15049,
#15050,#15051,#15052,#15053,#15054,#15055,#15056,#15057,#15058,#15059,#15060,
#15061,#15062,#15063,#15064,#15065,#15066,#15067,#15068,#15069,#15070,#15071,
#15072,#15073,#15074,#15075,#15076,#15077,#15078,#15079,#15080,#15081,#15082,
#15083,#15084,#15085,#15086,#15087,#15088,#15089,#15090,#15091,#15092,#15093,
#15094,#15095,#15096,#15097,#15098,#15099),.UNSPECIFIED.,.F.,.F.,(4,3,3,
3,3,3,3,3,3,3,3,3,3,3,3,3,3,3,4),(2.28557416296169E-7,4.45838597195228E-5,
0.103040149522257,0.1937218787354,0.25,0.251116964175455,0.330254232785831,
0.414362786403821,0.487704402379652,0.49847134002181,0.5,0.590018211501603,
0.650623800434858,0.733876213552138,0.75,0.804169141593649,0.887250644428625,
0.959806362374165,1.),.UNSPECIFIED.);
#213=B_SPLINE_CURVE_WITH_KNOTS('',3,(#15346,#15347,#15348,#15349,#15350,
#15351,#15352,#15353,#15354,#15355,#15356,#15357,#15358,#15359,#15360,#15361,
#15362,#15363,#15364,#15365,#15366,#15367,#15368,#15369,#15370,#15371,#15372,
#15373,#15374,#15375,#15376,#15377,#15378,#15379,#15380,#15381,#15382,#15383,
#15384,#15385,#15386,#15387,#15388,#15389,#15390,#15391,#15392,#15393,#15394,
#15395,#15396,#15397,#15398,#15399,#15400,#15401,#15402,#15403,#15404,#15405,
#15406,#15407,#15408,#15409,#15410,#15411,#15412,#15413,#15414,#15415,#15416,
#15417,#15418,#15419,#15420,#15421,#15422,#15423,#15424,#15425,#15426,#15427,
#15428,#15429,#15430,#15431,#15432,#15433,#15434,#15435,#15436,#15437,#15438,
#15439,#15440,#15441,#15442,#15443,#15444,#15445,#15446,#15447,#15448,#15449,
#15450,#15451,#15452,#15453,#15454,#15455,#15456,#15457,#15458,#15459,#15460,
#15461,#15462,#15463,#15464,#15465,#15466,#15467,#15468,#15469,#15470,#15471,
#15472,#15473,#15474,#15475,#15476,#15477,#15478,#15479,#15480,#15481,#15482,
#15483,#15484,#15485,#15486,#15487,#15488,#15489,#15490,#15491,#15492,#15493,
#15494,#15495,#15496,#15497,#15498,#15499,#15500,#15501,#15502,#15503,#15504,
#15505,#15506,#15507,#15508,#15509,#15510,#15511,#15512,#15513,#15514,#15515,
#15516,#15517,#15518,#15519,#15520,#15521,#15522,#15523,#15524,#15525,#15526,
#15527,#15528,#15529,#15530,#15531,#15532,#15533,#15534,#15535,#15536,#15537,
#15538,#15539,#15540,#15541,#15542,#15543,#15544,#15545,#15546,#15547,#15548,
#15549,#15550,#15551,#15552,#15553,#15554,#15555,#15556,#15557,#15558,#15559,
#15560,#15561,#15562,#15563,#15564,#15565,#15566,#15567,#15568,#15569,#15570,
#15571,#15572,#15573,#15574,#15575,#15576,#15577,#15578,#15579,#15580,#15581,
#15582,#15583,#15584,#15585,#15586,#15587,#15588,#15589,#15590,#15591,#15592,
#15593,#15594,#15595,#15596,#15597,#15598,#15599,#15600,#15601,#15602,#15603,
#15604,#15605,#15606,#15607,#15608,#15609,#15610,#15611,#15612,#15613,#15614,
#15615,#15616,#15617,#15618,#15619,#15620,#15621,#15622,#15623,#15624,#15625,
#15626,#15627,#15628,#15629,#15630,#15631,#15632,#15633,#15634,#15635,#15636,
#15637,#15638,#15639,#15640,#15641,#15642,#15643,#15644,#15645,#15646,#15647,
#15648,#15649,#15650,#15651,#15652,#15653,#15654,#15655,#15656,#15657,#15658,
#15659,#15660,#15661,#15662,#15663,#15664,#15665,#15666,#15667,#15668,#15669,
#15670,#15671,#15672,#15673,#15674,#15675,#15676,#15677,#15678,#15679,#15680,
#15681,#15682,#15683,#15684,#15685,#15686,#15687,#15688,#15689,#15690,#15691,
#15692,#15693,#15694,#15695,#15696,#15697,#15698,#15699,#15700,#15701,#15702,
#15703,#15704,#15705,#15706,#15707,#15708,#15709,#15710,#15711,#15712,#15713,
#15714,#15715,#15716,#15717,#15718,#15719,#15720,#15721,#15722,#15723,#15724,
#15725,#15726,#15727,#15728,#15729,#15730,#15731,#15732,#15733,#15734,#15735,
#15736,#15737,#15738,#15739,#15740,#15741,#15742,#15743,#15744,#15745,#15746,
#15747,#15748,#15749,#15750,#15751,#15752,#15753,#15754,#15755,#15756,#15757,
#15758,#15759,#15760,#15761,#15762,#15763,#15764,#15765,#15766,#15767,#15768,
#15769,#15770,#15771,#15772,#15773,#15774,#15775,#15776,#15777,#15778,#15779,
#15780,#15781,#15782,#15783,#15784,#15785,#15786,#15787,#15788,#15789,#15790,
#15791,#15792,#15793,#15794,#15795,#15796,#15797,#15798,#15799,#15800,#15801,
#15802,#15803,#15804,#15805,#15806,#15807,#15808,#15809,#15810,#15811,#15812,
#15813,#15814,#15815,#15816,#15817,#15818,#15819,#15820,#15821,#15822,#15823,
#15824,#15825,#15826,#15827,#15828,#15829,#15830,#15831,#15832,#15833,#15834,
#15835,#15836,#15837,#15838,#15839,#15840,#15841,#15842,#15843,#15844,#15845,
#15846,#15847,#15848,#15849,#15850,#15851,#15852,#15853,#15854,#15855,#15856,
#15857,#15858,#15859,#15860,#15861,#15862,#15863,#15864,#15865,#15866,#15867,
#15868,#15869,#15870,#15871,#15872,#15873,#15874,#15875,#15876,#15877,#15878,
#15879,#15880,#15881,#15882,#15883,#15884,#15885,#15886,#15887,#15888,#15889,
#15890,#15891,#15892,#15893,#15894,#15895,#15896,#15897,#15898),
 .UNSPECIFIED.,.F.,.F.,(4,3,3,3,3,3,3,3,3,3,3,3,3,3,3,3,3,3,3,3,3,3,3,3,
3,3,3,3,3,3,3,3,3,3,3,3,3,3,3,3,3,3,3,3,3,3,3,3,3,3,3,3,3,3,3,3,3,3,3,3,
3,3,3,3,3,3,3,3,3,3,3,3,3,3,3,3,3,3,3,3,3,3,3,3,3,3,3,3,3,3,3,3,3,3,3,3,
3,3,3,3,3,3,3,3,3,3,3,3,3,3,3,3,3,3,3,3,3,3,3,3,3,3,3,3,3,3,3,3,3,3,3,3,
3,3,3,3,3,3,3,3,3,3,3,3,3,3,3,3,3,3,3,3,3,3,3,3,3,3,3,3,3,3,3,3,3,3,3,3,
3,3,3,3,3,3,3,3,3,3,3,3,3,3,3,3,4),(0.,0.00625707247057022,0.0124987693041953,
0.01694915254237,0.0234597676321377,0.030130415664672,0.03389830508475,
0.0399367007525247,0.0449988678636083,0.05084745762712,0.0573205787421996,
0.0638925612737411,0.06779661016949,0.0736684880648363,0.0774993821578474,
0.0833631085591902,0.08474576271186,0.0911641141481979,0.097622449623175,
0.1016949152542,0.107509985014228,0.11000009299126,0.115816381204191,0.1186440677966,
0.125098471554685,0.131538419892334,0.135593220339,0.141475976279384,0.142500758333531,
0.148394384381762,0.1525423728814,0.159133140168786,0.165648703850875,0.1694915254237,
0.175001155269066,0.181100725849585,0.1864406779661,0.193286624103164,0.199984396474713,
0.2033898305085,0.207501147182458,0.213991841709094,0.2203389830508,0.227641776056833,
0.234693622399377,0.2372881355932,0.240000785292989,0.247217140945622,0.2542372881356,
0.2627118644068,0.27046083374304,0.271186440678,0.272500297585015,0.281238797730683,
0.2881355932203,0.297779235715604,0.304999989764099,0.3050847457627,0.314497758523359,
0.3220338983051,0.330516391338742,0.337499647052717,0.3389830508475,0.346610725412041,
0.354635740839695,0.3559322033898,0.363032643660964,0.369999158245744,0.3728813559322,
0.379849543493191,0.387071287109133,0.3898305084746,0.39626048216284,0.402498830192386,
0.4067796610169,0.41341773856689,0.420224034400144,0.4237288135593,0.429795057904492,
0.434998872355421,0.4406779661017,0.447151018279596,0.453728136179621,0.4576271186441,
0.463505178577456,0.467499311365647,0.473367745831533,0.4745762711864,0.480991993708343,
0.48745528955393,0.4915254237288,0.49734215213837,0.500000000044217,0.50581672845434,
0.5084745762712,0.514921286064733,0.521360156754795,0.5254237288136,0.531292163279376,
0.532500688634353,0.538378748567485,0.5423728813559,0.548941304568806,0.555442363344076,
0.5593220338983,0.565001127644577,0.571067371989645,0.5762711864407,0.583077792237934,
0.58974616604175,0.5932203389831,0.597501169807617,0.603931143495856,0.6101694915254,
0.617401150396015,0.624396992337254,0.6271186440678,0.630000841754257,0.637101282025258,
0.6440677966102,0.652108496201867,0.659748125429028,0.6610169491525,0.662500352947285,
0.670982845980953,0.6779661016949,0.687379114455814,0.6949152542373,0.695000010235901,
0.704643652731264,0.7118644067797,0.720602906926292,0.727499702414991,0.728813559322,
0.736562528658307,0.744733729676818,0.7457627118644,0.752979067516863,0.75999921470701,
0.7627118644068,0.769736974051562,0.777028740384925,0.7796610169492,0.786151711475952,
0.792498852817539,0.7966101694915,0.803277624820126,0.810122107164893,0.8135593220339,
0.819658892614575,0.824998844730939,0.8305084745763,0.836995593846511,0.843594013502594,
0.8474576271186,0.853351253166922,0.857499241666464,0.863381997606931,0.864406779661,
0.870822899633561,0.8772930400371,0.8813559322034,0.887172220416142,0.889999907008734,
0.895814976768646,0.8983050847458,0.904745868788263,0.911186525219332,0.9152542372881,
0.92111796368911,0.922500617842136,0.928372495737183,0.9322033898305,0.93876593182826,
0.945266618311092,0.9491525423729,0.955001132136413,0.961039527803894,0.9661016949153,
0.972771935762613,0.979314297120634,0.9830508474576,0.987501230695801,0.993758303164287,
1.),.UNSPECIFIED.);
#214=B_SPLINE_CURVE_WITH_KNOTS('',3,(#15900,#15901,#15902,#15903,#15904,
#15905,#15906,#15907,#15908,#15909,#15910,#15911,#15912,#15913,#15914,#15915,
#15916,#15917,#15918,#15919,#15920,#15921),.UNSPECIFIED.,.F.,.F.,(4,2,2,
2,2,2,2,2,2,2,4),(-0.108366379525748,-0.101004560326757,-0.0935005570164099,
-0.0775237436752796,-0.0642908492457915,-0.0539096504263199,-0.0435454398611879,
-0.0302727818609328,-0.0143408019654358,-0.00710487439831416,-1.34996523534921E-6),
 .UNSPECIFIED.);
#215=B_SPLINE_CURVE_WITH_KNOTS('',3,(#15922,#15923,#15924,#15925,#15926,
#15927,#15928,#15929,#15930,#15931,#15932,#15933,#15934,#15935,#15936,#15937,
#15938,#15939,#15940,#15941,#15942,#15943,#15944,#15945,#15946,#15947,#15948,
#15949,#15950,#15951,#15952,#15953,#15954,#15955,#15956,#15957,#15958,#15959,
#15960,#15961,#15962,#15963,#15964,#15965,#15966,#15967,#15968,#15969,#15970,
#15971,#15972,#15973,#15974,#15975,#15976,#15977,#15978,#15979,#15980,#15981,
#15982,#15983,#15984,#15985,#15986,#15987,#15988,#15989,#15990,#15991,#15992,
#15993,#15994,#15995,#15996,#15997,#15998,#15999,#16000,#16001,#16002,#16003,
#16004,#16005,#16006,#16007,#16008,#16009,#16010,#16011,#16012,#16013,#16014,
#16015,#16016,#16017,#16018,#16019,#16020,#16021,#16022,#16023,#16024,#16025,
#16026,#16027,#16028,#16029,#16030,#16031,#16032,#16033,#16034,#16035,#16036,
#16037,#16038,#16039,#16040,#16041,#16042,#16043,#16044,#16045,#16046,#16047,
#16048,#16049,#16050,#16051,#16052,#16053,#16054,#16055,#16056,#16057,#16058,
#16059,#16060,#16061,#16062,#16063,#16064,#16065,#16066,#16067,#16068,#16069,
#16070,#16071,#16072,#16073,#16074,#16075,#16076,#16077,#16078,#16079,#16080,
#16081,#16082,#16083,#16084,#16085,#16086,#16087,#16088,#16089,#16090,#16091,
#16092,#16093,#16094,#16095,#16096,#16097,#16098,#16099,#16100,#16101,#16102,
#16103,#16104,#16105,#16106,#16107,#16108,#16109,#16110,#16111,#16112,#16113,
#16114,#16115,#16116,#16117,#16118,#16119,#16120,#16121,#16122,#16123,#16124,
#16125,#16126,#16127,#16128,#16129,#16130,#16131,#16132,#16133,#16134,#16135,
#16136,#16137,#16138,#16139,#16140,#16141,#16142,#16143,#16144,#16145,#16146,
#16147,#16148,#16149,#16150,#16151,#16152,#16153,#16154,#16155,#16156,#16157,
#16158,#16159,#16160,#16161,#16162,#16163,#16164,#16165,#16166,#16167,#16168,
#16169,#16170,#16171,#16172,#16173,#16174,#16175,#16176,#16177,#16178,#16179,
#16180,#16181,#16182,#16183,#16184,#16185,#16186,#16187,#16188,#16189,#16190,
#16191,#16192,#16193,#16194,#16195,#16196,#16197,#16198,#16199,#16200,#16201,
#16202,#16203,#16204,#16205,#16206,#16207,#16208,#16209,#16210,#16211,#16212,
#16213,#16214,#16215,#16216,#16217,#16218,#16219,#16220,#16221,#16222,#16223,
#16224,#16225,#16226,#16227,#16228,#16229,#16230,#16231,#16232,#16233,#16234,
#16235,#16236,#16237,#16238,#16239,#16240,#16241,#16242,#16243,#16244,#16245,
#16246,#16247,#16248,#16249,#16250,#16251,#16252,#16253,#16254,#16255,#16256,
#16257,#16258,#16259,#16260,#16261,#16262,#16263,#16264,#16265,#16266,#16267,
#16268,#16269,#16270,#16271,#16272,#16273,#16274,#16275,#16276,#16277,#16278,
#16279,#16280,#16281,#16282,#16283,#16284,#16285,#16286,#16287,#16288,#16289,
#16290,#16291,#16292,#16293,#16294,#16295,#16296,#16297,#16298,#16299,#16300,
#16301,#16302,#16303,#16304,#16305,#16306,#16307,#16308,#16309,#16310,#16311,
#16312,#16313,#16314,#16315,#16316,#16317,#16318,#16319,#16320,#16321,#16322,
#16323,#16324,#16325,#16326,#16327,#16328,#16329,#16330,#16331,#16332,#16333,
#16334,#16335,#16336,#16337,#16338,#16339,#16340,#16341,#16342,#16343,#16344,
#16345,#16346,#16347,#16348,#16349,#16350,#16351,#16352,#16353,#16354,#16355,
#16356,#16357,#16358,#16359,#16360,#16361,#16362,#16363,#16364,#16365,#16366,
#16367,#16368,#16369,#16370,#16371,#16372,#16373,#16374,#16375,#16376,#16377,
#16378,#16379,#16380,#16381,#16382,#16383,#16384,#16385,#16386,#16387,#16388,
#16389,#16390,#16391,#16392,#16393,#16394,#16395,#16396,#16397,#16398,#16399,
#16400,#16401,#16402,#16403,#16404,#16405,#16406,#16407,#16408,#16409,#16410,
#16411,#16412,#16413,#16414,#16415,#16416,#16417,#16418,#16419,#16420,#16421,
#16422,#16423,#16424,#16425,#16426,#16427,#16428,#16429,#16430,#16431,#16432,
#16433,#16434,#16435,#16436,#16437,#16438),.UNSPECIFIED.,.F.,.F.,(4,3,3,
3,3,3,3,3,3,3,3,3,3,3,3,3,3,3,3,3,3,3,3,3,3,3,3,3,3,3,3,3,3,3,3,3,3,3,3,
3,3,3,3,3,3,3,3,3,3,3,3,3,3,3,3,3,3,3,3,3,3,3,3,3,3,3,3,3,3,3,3,3,3,3,3,
3,3,3,3,3,3,3,3,3,3,3,3,3,3,3,3,3,3,3,3,3,3,3,3,3,3,3,3,3,3,3,3,3,3,3,3,
3,3,3,3,3,3,3,3,3,3,3,3,3,3,3,3,3,3,3,3,3,3,3,3,3,3,3,3,3,3,3,3,3,3,3,3,
3,3,3,3,3,3,3,3,3,3,3,3,3,3,3,3,3,3,3,3,3,3,3,3,3,4),(0.,0.00661684587379473,
0.0124983817015441,0.01818181818182,0.0250973637786607,0.0321069452297743,
0.03636363636364,0.0426727071234223,0.045000237712052,0.0513095384438299,
0.05454545454545,0.0617456257730734,0.0688539134549294,0.07272727272727,
0.0775015374894184,0.0844748515404932,0.09090909090909,0.099999999999995,
0.108428992129646,0.1090909090909,0.110000217049001,0.120783250406619,0.1272727272727,
0.135245029127397,0.142498954903679,0.1454545454545,0.15285832598237,0.160506900312804,
0.1636363636364,0.170111030761004,0.174998755491224,0.181458998931522,0.1818181818182,
0.188790646918454,0.195802632396944,0.2,0.206382021661163,0.207500940519022,
0.213892440897663,0.2181818181818,0.225620516663835,0.232894893756836,0.2363636363636,
0.240001295616291,0.247492969823552,0.2545454545455,0.264726443160272,0.27249996074925,
0.2727272727273,0.282186826708758,0.2909090909091,0.298158861584068,0.304998574949384,
0.3090909090909,0.316250191676584,0.32358191434256,0.3272727272727,0.333626040135738,
0.337499304110204,0.343846043754328,0.3454545454545,0.352469372214463,0.35947119982488,
0.3636363636364,0.370001396084259,0.376550683587071,0.3818181818182,0.389651329370141,
0.397226012190253,0.4,0.402500854076842,0.410898578978884,0.4181818181818,
0.428299211683941,0.434999622589457,0.4363636363636,0.444446021132232,0.452935779498618,
0.4545454545455,0.461363107469256,0.467498436348121,0.4727272727273,0.479753856203258,
0.48689398608381,0.4909090909091,0.497221599850067,0.499999999973427,0.506312508914082,
0.5090909090909,0.516218473166076,0.523276759558518,0.5272727272727,0.532501563651881,
0.539319216575566,0.5454545454545,0.553958903432471,0.562058004187475,0.5636363636364,
0.565000377410548,0.575117770912058,0.5818181818182,0.590215906720766,0.597499145923165,
0.6,0.607544534174676,0.615369925925628,0.6181818181818,0.624731105684416,
0.629998603915741,0.6363636363636,0.643337807374075,0.650372265605402,0.6545454545455,
0.66089219418975,0.662500695889806,0.668854008752749,0.6727272727273,0.68005444891509,
0.687247435926077,0.6909090909091,0.695001425050612,0.702251195725806,0.7090909090909,
0.718550463073272,0.7272727272727,0.727500039250745,0.737681027863759,0.7454545454545,
0.752946219661041,0.759998704383708,0.7636363636364,0.770877064963762,0.778316872208324,
0.7818181818182,0.788209682196738,0.792499059480988,0.798881081142194,0.8,
0.806989821147026,0.81398789866388,0.8181818181818,0.824642061622016,0.825001244508772,
0.831475911633192,0.8363636363636,0.844016413814312,0.851452480642349,0.8545454545455,
0.857501045096315,0.865473346951193,0.8727272727273,0.883510306083999,0.889999782950997,
0.8909090909091,0.899338083038148,0.908253221413727,0.9090909090909,0.916064223141629,
0.922498462510559,0.9272727272727,0.934348435683951,0.941558336300596,0.9454545454545,
0.951763846186328,0.954999762287933,0.961308833047855,0.9636363636364,0.970630376636484,
0.977577338426374,0.9818181818182,0.987501618298468,0.994118464171033,1.),
 .UNSPECIFIED.);
#216=B_SPLINE_CURVE_WITH_KNOTS('',3,(#16684,#16685,#16686,#16687,#16688,
#16689,#16690,#16691,#16692,#16693,#16694,#16695,#16696,#16697,#16698,#16699,
#16700,#16701,#16702,#16703,#16704,#16705),.UNSPECIFIED.,.F.,.F.,(4,2,2,
2,2,2,2,2,2,2,4),(-0.107848148767986,-0.10078133624504,-0.0935834381175982,
-0.0777250902731328,-0.0645137902634984,-0.0541974885556667,-0.0438642827821331,
-0.0306925477519394,-0.0147895883407361,-0.00732502687635996,-1.25961705293921E-6),
 .UNSPECIFIED.);
#274=SHAPE_REPRESENTATION_RELATIONSHIP('SRR','None',#17199,#290);
#290=ADVANCED_BREP_SHAPE_REPRESENTATION('',(#340),#17106);
#319=STYLED_ITEM('',(#17298),#340);
#340=MANIFOLD_SOLID_BREP('Body1',#6026);
#1289=FACE_OUTER_BOUND('',#1761,.T.);
#1290=FACE_OUTER_BOUND('',#1762,.T.);
#1291=FACE_OUTER_BOUND('',#1763,.T.);
#1292=FACE_OUTER_BOUND('',#1764,.T.);
#1293=FACE_OUTER_BOUND('',#1765,.T.);
#1294=FACE_OUTER_BOUND('',#1766,.T.);
#1295=FACE_OUTER_BOUND('',#1767,.T.);
#1296=FACE_OUTER_BOUND('',#1768,.T.);
#1761=EDGE_LOOP('',(#5176,#5177));
#1762=EDGE_LOOP('',(#5178,#5179,#5180,#5181));
#1763=EDGE_LOOP('',(#5182,#5183,#5184,#5185));
#1764=EDGE_LOOP('',(#5186,#5187,#5188,#5189));
#1765=EDGE_LOOP('',(#5190,#5191,#5192,#5193));
#1766=EDGE_LOOP('',(#5194,#5195,#5196,#5197));
#1767=EDGE_LOOP('',(#5198,#5199,#5200,#5201));
#1768=EDGE_LOOP('',(#5202,#5203));
#2992=VERTEX_POINT('',#11524);
#2993=VERTEX_POINT('',#11525);
#2994=VERTEX_POINT('',#11920);
#2995=VERTEX_POINT('',#12474);
#2996=VERTEX_POINT('',#13580);
#2997=VERTEX_POINT('',#14098);
#2998=VERTEX_POINT('',#15345);
#2999=VERTEX_POINT('',#15899);
#3747=EDGE_CURVE('',#2992,#2993,#203,.T.);
#3748=EDGE_CURVE('',#2993,#2992,#204,.T.);
#3749=EDGE_CURVE('',#2993,#2994,#205,.T.);
#3750=EDGE_CURVE('',#2995,#2994,#206,.T.);
#3751=EDGE_CURVE('',#2992,#2995,#207,.T.);
#3752=EDGE_CURVE('',#2994,#2995,#208,.T.);
#3753=EDGE_CURVE('',#2995,#2996,#209,.T.);
#3754=EDGE_CURVE('',#2997,#2996,#210,.T.);
#3755=EDGE_CURVE('',#2994,#2997,#211,.T.);
#3756=EDGE_CURVE('',#2996,#2997,#212,.T.);
#3757=EDGE_CURVE('',#2997,#2998,#213,.T.);
#3758=EDGE_CURVE('',#2999,#2998,#214,.T.);
#3759=EDGE_CURVE('',#2996,#2999,#215,.T.);
#3760=EDGE_CURVE('',#2998,#2999,#216,.T.);
#5176=ORIENTED_EDGE('',*,*,#3747,.F.);
#5177=ORIENTED_EDGE('',*,*,#3748,.F.);
#5178=ORIENTED_EDGE('',*,*,#3747,.T.);
#5179=ORIENTED_EDGE('',*,*,#3749,.T.);
#5180=ORIENTED_EDGE('',*,*,#3750,.F.);
#5181=ORIENTED_EDGE('',*,*,#3751,.F.);
#5182=ORIENTED_EDGE('',*,*,#3748,.T.);
#5183=ORIENTED_EDGE('',*,*,#3751,.T.);
#5184=ORIENTED_EDGE('',*,*,#3752,.F.);
#5185=ORIENTED_EDGE('',*,*,#3749,.F.);
#5186=ORIENTED_EDGE('',*,*,#3752,.T.);
#5187=ORIENTED_EDGE('',*,*,#3753,.T.);
#5188=ORIENTED_EDGE('',*,*,#3754,.F.);
#5189=ORIENTED_EDGE('',*,*,#3755,.F.);
#5190=ORIENTED_EDGE('',*,*,#3750,.T.);
#5191=ORIENTED_EDGE('',*,*,#3755,.T.);
#5192=ORIENTED_EDGE('',*,*,#3756,.F.);
#5193=ORIENTED_EDGE('',*,*,#3753,.F.);
#5194=ORIENTED_EDGE('',*,*,#3756,.T.);
#5195=ORIENTED_EDGE('',*,*,#3757,.T.);
#5196=ORIENTED_EDGE('',*,*,#3758,.F.);
#5197=ORIENTED_EDGE('',*,*,#3759,.F.);
#5198=ORIENTED_EDGE('',*,*,#3754,.T.);
#5199=ORIENTED_EDGE('',*,*,#3759,.T.);
#5200=ORIENTED_EDGE('',*,*,#3760,.F.);
#5201=ORIENTED_EDGE('',*,*,#3757,.F.);
#5202=ORIENTED_EDGE('',*,*,#3758,.T.);
#5203=ORIENTED_EDGE('',*,*,#3760,.T.);
#5616=PLANE('',#6816);
#5617=PLANE('',#6817);
#5937=ADVANCED_FACE('',(#1289),#5616,.F.);
#5938=ADVANCED_FACE('',(#1290),#11,.T.);
#5939=ADVANCED_FACE('',(#1291),#12,.T.);
#5940=ADVANCED_FACE('',(#1292),#13,.T.);
#5941=ADVANCED_FACE('',(#1293),#14,.T.);
#5942=ADVANCED_FACE('',(#1294),#15,.T.);
#5943=ADVANCED_FACE('',(#1295),#16,.T.);
#5944=ADVANCED_FACE('',(#1296),#5617,.T.);
#6026=CLOSED_SHELL('',(#5937,#5938,#5939,#5940,#5941,#5942,#5943,#5944));
#6815=AXIS2_PLACEMENT_3D('',#11522,#8470,#8471);
#6816=AXIS2_PLACEMENT_3D('',#11523,#8472,#8473);
#6817=AXIS2_PLACEMENT_3D('',#16706,#8474,#8475);
#8470=DIRECTION('axis',(0.,0.,1.));
#8471=DIRECTION('refdir',(1.,0.,0.));
#8472=DIRECTION('center_axis',(0.,0.,1.));
#8473=DIRECTION('ref_axis',(-1.,0.,0.));
#8474=DIRECTION('center_axis',(0.500000000000017,0.,-0.866025403784429));
#8475=DIRECTION('ref_axis',(0.866025403784429,0.,0.500000000000017));
#11522=CARTESIAN_POINT('',(0.,0.,0.));
#11523=CARTESIAN_POINT('Origin',(2.5,6.35,0.));
#11524=CARTESIAN_POINT('',(2.14860532402759,6.34999974649317,8.70644660934498E-7));
#11525=CARTESIAN_POINT('',(2.8478479312681,6.34999003058963,5.15480744294665E-6));
#11526=CARTESIAN_POINT('Ctrl Pts',(2.1486053225045,6.34999974649289,3.65871305311616E-18));
#11527=CARTESIAN_POINT('Ctrl Pts',(2.14860981858709,6.32558894509038,3.65871305311616E-18));
#11528=CARTESIAN_POINT('Ctrl Pts',(2.1520163214667,6.30133488915141,-3.08118123936608E-14));
#11529=CARTESIAN_POINT('Ctrl Pts',(2.16455445600999,6.25365679968968,-3.08118123936608E-14));
#11530=CARTESIAN_POINT('Ctrl Pts',(2.17377138804027,6.23034157217996,-3.09576802169716E-14));
#11531=CARTESIAN_POINT('Ctrl Pts',(2.20956345199181,6.16111636506853,-3.09576802169716E-14));
#11532=CARTESIAN_POINT('Ctrl Pts',(2.24442612782612,6.11856284402862,-3.22770038253786E-14));
#11533=CARTESIAN_POINT('Ctrl Pts',(2.31888272951377,6.05624332235576,-3.22770038253786E-14));
#11534=CARTESIAN_POINT('Ctrl Pts',(2.35750239145032,6.03309219630646,-3.42413397489756E-14));
#11535=CARTESIAN_POINT('Ctrl Pts',(2.43122237823416,6.00648674167113,-3.42413397489756E-14));
#11536=CARTESIAN_POINT('Ctrl Pts',(2.46540202197458,5.99983772837923,-3.50466365285637E-14));
#11537=CARTESIAN_POINT('Ctrl Pts',(2.53454022793098,6.00026453242939,-3.50466365285637E-14));
#11538=CARTESIAN_POINT('Ctrl Pts',(2.56868396399153,6.00727311231843,-3.43411381866254E-14));
#11539=CARTESIAN_POINT('Ctrl Pts',(2.64251672073783,6.03475210628683,-3.43411381866254E-14));
#11540=CARTESIAN_POINT('Ctrl Pts',(2.68113652459894,6.05843083260967,-3.21032521178046E-14));
#11541=CARTESIAN_POINT('Ctrl Pts',(2.75646506084904,6.12284688425985,-3.21032521178045E-14));
#11542=CARTESIAN_POINT('Ctrl Pts',(2.79073198571329,6.16644333813941,-2.3349794938747E-14));
#11543=CARTESIAN_POINT('Ctrl Pts',(2.82474145767008,6.23412167292725,-2.3349794938747E-14));
#11544=CARTESIAN_POINT('Ctrl Pts',(2.83343278835146,6.2567646493699,-2.41677926809621E-14));
#11545=CARTESIAN_POINT('Ctrl Pts',(2.8451097183543,6.30324581117954,-2.41677926809621E-14));
#11546=CARTESIAN_POINT('Ctrl Pts',(2.84795198077779,6.32630237599366,6.695966560974E-17));
#11547=CARTESIAN_POINT('Ctrl Pts',(2.84784813424439,6.34999165496226,6.695966560974E-17));
#11548=CARTESIAN_POINT('Ctrl Pts',(2.84815123000917,6.34999228813821,-1.05605361430648E-16));
#11549=CARTESIAN_POINT('Ctrl Pts',(2.84815609492309,6.37365275855263,-1.05605361430648E-16));
#11550=CARTESIAN_POINT('Ctrl Pts',(2.84496435783334,6.39716343968712,-1.99114533756745E-14));
#11551=CARTESIAN_POINT('Ctrl Pts',(2.83316209106941,6.44347800850811,-1.99114533756745E-14));
#11552=CARTESIAN_POINT('Ctrl Pts',(2.82446061839549,6.46618019518869,-1.99676121479179E-14));
#11553=CARTESIAN_POINT('Ctrl Pts',(2.78983170226385,6.53526148665337,-1.99676121479179E-14));
#11554=CARTESIAN_POINT('Ctrl Pts',(2.75535086791679,6.5782452428205,-2.11426632102796E-14));
#11555=CARTESIAN_POINT('Ctrl Pts',(2.68122114567467,6.64162093032331,-2.11426632102796E-14));
#11556=CARTESIAN_POINT('Ctrl Pts',(2.64251574891792,6.66533843223839,-2.16999633566802E-14));
#11557=CARTESIAN_POINT('Ctrl Pts',(2.5686604418669,6.69282040482859,-2.16999633566802E-14));
#11558=CARTESIAN_POINT('Ctrl Pts',(2.53453195804941,6.69982796752832,-2.21446346512339E-14));
#11559=CARTESIAN_POINT('Ctrl Pts',(2.46541194722646,6.70025495629189,-2.21446346512339E-14));
#11560=CARTESIAN_POINT('Ctrl Pts',(2.43124007875004,6.69360737099457,-2.18419242653537E-14));
#11561=CARTESIAN_POINT('Ctrl Pts',(2.35752298816286,6.6670078332254,-2.18419242653537E-14));
#11562=CARTESIAN_POINT('Ctrl Pts',(2.31889621664184,6.6438557899457,-2.14275374584633E-14));
#11563=CARTESIAN_POINT('Ctrl Pts',(2.2444310357439,6.58153621615099,-2.14275374584633E-14));
#11564=CARTESIAN_POINT('Ctrl Pts',(2.20956813686693,6.53898582858603,-2.0492122078762E-14));
#11565=CARTESIAN_POINT('Ctrl Pts',(2.1737661560062,6.46974575644438,-2.0492122078762E-14));
#11566=CARTESIAN_POINT('Ctrl Pts',(2.16454384175254,6.44641342304313,-2.02715049049549E-14));
#11567=CARTESIAN_POINT('Ctrl Pts',(2.15200448436394,6.39870188647906,-2.02715049049549E-14));
#11568=CARTESIAN_POINT('Ctrl Pts',(2.14860099263747,6.37442980938693,2.47455274716954E-18));
#11569=CARTESIAN_POINT('Ctrl Pts',(2.14860532218071,6.34999974649284,2.47455274716954E-18));
#11570=CARTESIAN_POINT('Ctrl Pts',(1.965062045595,6.552581420145,-0.9330800615582));
#11571=CARTESIAN_POINT('Ctrl Pts',(2.189120896398,6.506720309034,-0.461213217722));
#11572=CARTESIAN_POINT('Ctrl Pts',(2.281137760944,6.414998086811,0.6484217724168));
#11573=CARTESIAN_POINT('Ctrl Pts',(1.286585694332,6.277414753478,1.992594001388));
#11574=CARTESIAN_POINT('Ctrl Pts',(-0.3475095635628,6.139831420145,2.346140516093));
#11575=CARTESIAN_POINT('Ctrl Pts',(-1.808863355149,6.002248086811,1.534037087326));
#11576=CARTESIAN_POINT('Ctrl Pts',(-2.371417852518,5.864664753478,-0.04036000087055));
#11577=CARTESIAN_POINT('Ctrl Pts',(-1.755619809682,5.727081420145,-1.594692483255));
#11578=CARTESIAN_POINT('Ctrl Pts',(-0.2674627113239,5.589498086811,-2.356631432544));
#11579=CARTESIAN_POINT('Ctrl Pts',(1.353595852992,5.451914753478,-1.947569137845));
#11580=CARTESIAN_POINT('Ctrl Pts',(2.302058075825,5.314331420145,-0.570767882745));
#11581=CARTESIAN_POINT('Ctrl Pts',(2.106637066738,5.176748086811,1.089645653198));
#11582=CARTESIAN_POINT('Ctrl Pts',(0.8644366963533,5.039164753478,2.208618700598));
#11583=CARTESIAN_POINT('Ctrl Pts',(-0.8072987362944,4.901581420145,2.230138139478));
#11584=CARTESIAN_POINT('Ctrl Pts',(-2.077890724405,4.763998086811,1.143511043905));
#11585=CARTESIAN_POINT('Ctrl Pts',(-2.31598729768,4.626414753478,-0.5113220189456));
#11586=CARTESIAN_POINT('Ctrl Pts',(-1.403279241419,4.488831420145,-1.912081258926));
#11587=CARTESIAN_POINT('Ctrl Pts',(0.206712538824,4.351248086811,-2.362735130395));
#11588=CARTESIAN_POINT('Ctrl Pts',(1.713989702755,4.213664753478,-1.639355565149));
#11589=CARTESIAN_POINT('Ctrl Pts',(2.369592383424,4.076081420145,-0.1013869148015));
#11590=CARTESIAN_POINT('Ctrl Pts',(1.847754286391,3.938498086811,1.486960479376));
#11591=CARTESIAN_POINT('Ctrl Pts',(0.4077746306339,3.800914753478,2.336443284436));
#11592=CARTESIAN_POINT('Ctrl Pts',(-1.234826573077,3.663331420145,2.024956962767));
#11593=CARTESIAN_POINT('Ctrl Pts',(-2.263847498087,3.525748086811,0.7072777996607));
#11594=CARTESIAN_POINT('Ctrl Pts',(-2.167971838247,3.388164753478,-0.961844825848));
#11595=CARTESIAN_POINT('Ctrl Pts',(-0.9948398588049,3.250581420145,-2.153030639647));
#11596=CARTESIAN_POINT('Ctrl Pts',(0.6726241054473,3.112998086811,-2.274384493346));
#11597=CARTESIAN_POINT('Ctrl Pts',(2.005863443573,2.975414753478,-1.265605340552));
#11598=CARTESIAN_POINT('Ctrl Pts',(2.342399127393,2.837831420145,0.3720455468077));
#11599=CARTESIAN_POINT('Ctrl Pts',(1.514999911603,2.700248086811,1.824837442277));
#11600=CARTESIAN_POINT('Ctrl Pts',(-0.06517291272752,2.562664753478,2.370841772339));
#11601=CARTESIAN_POINT('Ctrl Pts',(-1.613049883864,2.425081420145,1.738908759939));
#11602=CARTESIAN_POINT('Ctrl Pts',(-2.359079411806,2.287498086811,0.2424553735028));
#11603=CARTESIAN_POINT('Ctrl Pts',(-2.075774396281,2.195775864589,-0.8343432069565));
#11604=CARTESIAN_POINT('Ctrl Pts',(-1.773180685345,2.149914753478,-1.260133922024));
#11605=CARTESIAN_POINT('Ctrl Pts',(1.950430605956,6.514669866795,-0.9261325432193));
#11606=CARTESIAN_POINT('Ctrl Pts',(2.172821161573,6.468808755684,-0.4577791208848));
#11607=CARTESIAN_POINT('Ctrl Pts',(2.264152887855,6.377086533461,0.6435937599656));
#11608=CARTESIAN_POINT('Ctrl Pts',(1.277006047232,6.239503200128,1.977757564583));
#11609=CARTESIAN_POINT('Ctrl Pts',(-0.3449220802747,6.101919866795,2.328671646129));
#11610=CARTESIAN_POINT('Ctrl Pts',(-1.795394938182,5.964336533461,1.522614969079));
#11611=CARTESIAN_POINT('Ctrl Pts',(-2.353760772811,5.826753200128,-0.04005948877329));
#11612=CARTESIAN_POINT('Ctrl Pts',(-1.742547832982,5.689169866795,-1.582818737658));
#11613=CARTESIAN_POINT('Ctrl Pts',(-0.2654712401003,5.551586533461,-2.339084449417));
#11614=CARTESIAN_POINT('Ctrl Pts',(1.343517262312,5.414003200128,-1.933067946727));
#11615=CARTESIAN_POINT('Ctrl Pts',(2.284917434461,5.276419866795,-0.5665180648611));
#11616=CARTESIAN_POINT('Ctrl Pts',(2.0909514892,5.138836533461,1.081532380318));
#11617=CARTESIAN_POINT('Ctrl Pts',(0.8580002821075,5.001253200128,2.192173789215));
#11618=CARTESIAN_POINT('Ctrl Pts',(-0.8012877593092,4.863669866795,2.213532998868));
#11619=CARTESIAN_POINT('Ctrl Pts',(-2.0624191861,4.726086533461,1.134996700628));
#11620=CARTESIAN_POINT('Ctrl Pts',(-2.298742942253,4.588503200128,-0.5075148224894));
#11621=CARTESIAN_POINT('Ctrl Pts',(-1.392830718655,4.450919866795,-1.897844303107));
#11622=CARTESIAN_POINT('Ctrl Pts',(0.2051734006369,4.313336533461,-2.345142700415));
#11623=CARTESIAN_POINT('Ctrl Pts',(1.701227695095,4.175753200128,-1.627149267617));
#11624=CARTESIAN_POINT('Ctrl Pts',(2.351948895778,4.038169866795,-0.1006320091092));
#11625=CARTESIAN_POINT('Ctrl Pts',(1.833996295711,3.900586533461,1.475888883674));
#11626=CARTESIAN_POINT('Ctrl Pts',(0.4047384263025,3.763003200128,2.319046618024));
#11627=CARTESIAN_POINT('Ctrl Pts',(-1.225632313532,3.625419866795,2.009879558143));
#11628=CARTESIAN_POINT('Ctrl Pts',(-2.246991364667,3.487836533461,0.7020115575811));
#11629=CARTESIAN_POINT('Ctrl Pts',(-2.151829574871,3.350253200128,-0.9546831311102));
#11630=CARTESIAN_POINT('Ctrl Pts',(-0.9874324899755,3.212669866795,-2.1369996253));
#11631=CARTESIAN_POINT('Ctrl Pts',(0.6676158875029,3.075086533461,-2.25744990367));
#11632=CARTESIAN_POINT('Ctrl Pts',(1.990928205287,2.937503200128,-1.256181908764));
#11633=CARTESIAN_POINT('Ctrl Pts',(2.324958115024,2.799919866795,0.3692753737369));
#11634=CARTESIAN_POINT('Ctrl Pts',(1.503719540172,2.662336533461,1.811250085609));
#11635=CARTESIAN_POINT('Ctrl Pts',(-0.06468764889537,2.524753200128,2.353188982004));
#11636=CARTESIAN_POINT('Ctrl Pts',(-1.601039452915,2.387169866795,1.725961210209));
#11637=CARTESIAN_POINT('Ctrl Pts',(-2.34151420154,2.249586533461,0.2406501016691));
#11638=CARTESIAN_POINT('Ctrl Pts',(-2.060318615711,2.157864311239,-0.8281308625178));
#11639=CARTESIAN_POINT('Ctrl Pts',(-1.759977954049,2.112003200128,-1.250751229269));
#11640=CARTESIAN_POINT('Ctrl Pts',(1.924102649941,6.387168266731,-0.9136311105677));
#11641=CARTESIAN_POINT('Ctrl Pts',(2.143491258835,6.34130715562,-0.4515997733487));
#11642=CARTESIAN_POINT('Ctrl Pts',(2.233590140603,6.249584933397,0.6349061869998));
#11643=CARTESIAN_POINT('Ctrl Pts',(1.259768336267,6.112001600064,1.951060734658));
#11644=CARTESIAN_POINT('Ctrl Pts',(-0.3402661374637,5.974418266731,2.297237990153));
#11645=CARTESIAN_POINT('Ctrl Pts',(-1.771159736572,5.836834933397,1.502061897459));
#11646=CARTESIAN_POINT('Ctrl Pts',(-2.321988450378,5.699251600064,-0.03951874435758));
#11647=CARTESIAN_POINT('Ctrl Pts',(-1.719025989877,5.561668266731,-1.561453003354));
#11648=CARTESIAN_POINT('Ctrl Pts',(-0.261887767245,5.424084933397,-2.307510235851));
#11649=CARTESIAN_POINT('Ctrl Pts',(1.325381747376,5.286501600064,-1.906974361177));
#11650=CARTESIAN_POINT('Ctrl Pts',(2.254074396247,5.148918266731,-0.5588709008719));
#11651=CARTESIAN_POINT('Ctrl Pts',(2.062726707109,5.011334933397,1.066933277509));
#11652=CARTESIAN_POINT('Ctrl Pts',(0.8464185351747,4.873751600064,2.162582654353));
#11653=CARTESIAN_POINT('Ctrl Pts',(-0.7904715483566,4.736168266731,2.183653545964));
#11654=CARTESIAN_POINT('Ctrl Pts',(-2.034579548304,4.598584933397,1.119675907815));
#11655=CARTESIAN_POINT('Ctrl Pts',(-2.267713279938,4.461001600064,-0.500664115839));
#11656=CARTESIAN_POINT('Ctrl Pts',(-1.374029544296,4.323418266731,-1.872226185147));
#11657=CARTESIAN_POINT('Ctrl Pts',(0.2024038602847,4.185834933397,-2.313486709334));
#11658=CARTESIAN_POINT('Ctrl Pts',(1.678263613322,4.048251600064,-1.605185136098));
#11659=CARTESIAN_POINT('Ctrl Pts',(2.32020103103,3.910668266731,-0.09927362440098));
#11660=CARTESIAN_POINT('Ctrl Pts',(1.809240032321,3.773084933397,1.455966545758));
#11661=CARTESIAN_POINT('Ctrl Pts',(0.3992750504445,3.635501600064,2.287742885828));
#11662=CARTESIAN_POINT('Ctrl Pts',(-1.209088072716,3.497918266731,1.98274912836));
#11663=CARTESIAN_POINT('Ctrl Pts',(-2.216660272838,3.360334933397,0.6925354299232));
#11664=CARTESIAN_POINT('Ctrl Pts',(-2.122783027803,3.222751600064,-0.9417963073456));
#11665=CARTESIAN_POINT('Ctrl Pts',(-0.9741035978403,3.085168266731,-2.108153260827));
#11666=CARTESIAN_POINT('Ctrl Pts',(0.6586040510052,2.947584933397,-2.226977636885));
#11667=CARTESIAN_POINT('Ctrl Pts',(1.964053591005,2.810001600064,-1.239225293163));
#11668=CARTESIAN_POINT('Ctrl Pts',(2.293574586278,2.672418266731,0.3642906971391));
#11669=CARTESIAN_POINT('Ctrl Pts',(1.483421529162,2.534834933397,1.786800862735));
#11670=CARTESIAN_POINT('Ctrl Pts',(-0.06381446039555,2.397251600064,2.321424377909));
#11671=CARTESIAN_POINT('Ctrl Pts',(-1.579427765646,2.259668266731,1.702663262213));
#11672=CARTESIAN_POINT('Ctrl Pts',(-2.309907189879,2.122084933397,0.2374016778224));
#11673=CARTESIAN_POINT('Ctrl Pts',(-2.032507332538,2.030362711175,-0.8169523089941));
#11674=CARTESIAN_POINT('Ctrl Pts',(-1.736220829843,1.984501600064,-1.233867919887));
#11675=CARTESIAN_POINT('Ctrl Pts',(2.02121917785,6.172166666667,-0.9597454284554));
#11676=CARTESIAN_POINT('Ctrl Pts',(2.251681135642,6.126305555556,-0.4743936726209));
#11677=CARTESIAN_POINT('Ctrl Pts',(2.346327638903,6.034583333333,0.6669522342475));
#11678=CARTESIAN_POINT('Ctrl Pts',(1.323353471287,5.897,2.049537936119));
#11679=CARTESIAN_POINT('Ctrl Pts',(-0.357440619208,5.759416666667,2.413188029197));
#11680=CARTESIAN_POINT('Ctrl Pts',(-1.860556673889,5.621833333333,1.577876478448));
#11681=CARTESIAN_POINT('Ctrl Pts',(-2.439187736057,5.48425,-0.04151340053637));
#11682=CARTESIAN_POINT('Ctrl Pts',(-1.805791545513,5.346666666667,-1.6402652716));
#11683=CARTESIAN_POINT('Ctrl Pts',(-0.2751062047631,5.209083333333,-2.423978752864));
#11684=CARTESIAN_POINT('Ctrl Pts',(1.39227863225,5.0715,-2.00322636144));
#11685=CARTESIAN_POINT('Ctrl Pts',(2.367845810168,4.933916666667,-0.5870791679536));
#11686=CARTESIAN_POINT('Ctrl Pts',(2.166840100345,4.796333333333,1.120785318836));
#11687=CARTESIAN_POINT('Ctrl Pts',(0.8891403875127,4.65875,2.271736144014));
#11688=CARTESIAN_POINT('Ctrl Pts',(-0.8303695507784,4.521166666667,2.293870560918));
#11689=CARTESIAN_POINT('Ctrl Pts',(-2.137272251052,4.383583333333,1.176190063415));
#11690=CARTESIAN_POINT('Ctrl Pts',(-2.382173098413,4.246,-0.5259344726884));
#11691=CARTESIAN_POINT('Ctrl Pts',(-1.443381862163,4.108416666667,-1.966724317338));
#11692=CARTESIAN_POINT('Ctrl Pts',(0.212619926536,3.970833333333,-2.430256880916));
#11693=CARTESIAN_POINT('Ctrl Pts',(1.762971742094,3.83325,-1.68620472571));
#11694=CARTESIAN_POINT('Ctrl Pts',(2.437310099089,3.695666666667,-0.1042843288533));
#11695=CARTESIAN_POINT('Ctrl Pts',(1.900559022032,3.558083333333,1.529454525041));
#11696=CARTESIAN_POINT('Ctrl Pts',(0.4194279287647,3.4205,2.403213672081));
#11697=CARTESIAN_POINT('Ctrl Pts',(-1.270115188687,3.282916666667,2.082825759441));
#11698=CARTESIAN_POINT('Ctrl Pts',(-2.328543258529,3.145333333333,0.7274902367315));
#11699=CARTESIAN_POINT('Ctrl Pts',(-2.229927684129,3.00775,-0.9893322261645));
#11700=CARTESIAN_POINT('Ctrl Pts',(-1.023270184274,2.870166666667,-2.21455949908));
#11701=CARTESIAN_POINT('Ctrl Pts',(0.6918462164907,2.732583333333,-2.339381377835));
#11702=CARTESIAN_POINT('Ctrl Pts',(2.063186589648,2.595,-1.301773545343));
#11703=CARTESIAN_POINT('Ctrl Pts',(2.409339719873,2.457416666667,0.3826777866516));
#11704=CARTESIAN_POINT('Ctrl Pts',(1.558295262298,2.319833333333,1.876987265138));
#11705=CARTESIAN_POINT('Ctrl Pts',(-0.06703541060015,2.18225,2.438595192779));
#11706=CARTESIAN_POINT('Ctrl Pts',(-1.659147286165,2.044666666667,1.788602930884));
#11707=CARTESIAN_POINT('Ctrl Pts',(-2.426496689966,1.907083333333,0.2493842124707));
#11708=CARTESIAN_POINT('Ctrl Pts',(-2.135095442945,1.815361111111,-0.8581868926683));
#11709=CARTESIAN_POINT('Ctrl Pts',(-1.823854272208,1.7695,-1.29614576576));
#11710=CARTESIAN_POINT('Ctrl Pts',(2.22783143602,6.057791466659,-1.057852141678));
#11711=CARTESIAN_POINT('Ctrl Pts',(2.481851583861,6.011930355548,-0.5228869528331));
#11712=CARTESIAN_POINT('Ctrl Pts',(2.586173004113,5.920208133325,0.7351291587096));
#11713=CARTESIAN_POINT('Ctrl Pts',(1.458628780396,5.782624799992,2.259044983067));
#11714=CARTESIAN_POINT('Ctrl Pts',(-0.3939787711836,5.645041466659,2.659867970475));
#11715=CARTESIAN_POINT('Ctrl Pts',(-2.050745753855,5.507458133325,1.739169536568));
#11716=CARTESIAN_POINT('Ctrl Pts',(-2.688525408967,5.369874799992,-0.04575696675776));
#11717=CARTESIAN_POINT('Ctrl Pts',(-1.990382446436,5.232291466659,-1.807935811973));
#11718=CARTESIAN_POINT('Ctrl Pts',(-0.3032280011649,5.094708133325,-2.67176173918));
#11719=CARTESIAN_POINT('Ctrl Pts',(1.534599581587,4.957124799992,-2.20799936513));
#11720=CARTESIAN_POINT('Ctrl Pts',(2.609890797272,4.819541466659,-0.6470913397877));
#11721=CARTESIAN_POINT('Ctrl Pts',(2.388337962196,4.681958133325,1.235353787306));
#11722=CARTESIAN_POINT('Ctrl Pts',(0.9800297404872,4.544374799992,2.503956647275));
#11723=CARTESIAN_POINT('Ctrl Pts',(-0.9152512547927,4.406791466659,2.528353679688));
#11724=CARTESIAN_POINT('Ctrl Pts',(-2.355747640042,4.269208133325,1.29642209352));
#11725=CARTESIAN_POINT('Ctrl Pts',(-2.625682643845,4.131624799992,-0.5796963359453));
#11726=CARTESIAN_POINT('Ctrl Pts',(-1.590926665424,3.994041466659,-2.167766023679));
#11727=CARTESIAN_POINT('Ctrl Pts',(0.2343542756037,3.856458133325,-2.678681627526));
#11728=CARTESIAN_POINT('Ctrl Pts',(1.943185534203,3.718874799992,-1.858571270583));
#11729=CARTESIAN_POINT('Ctrl Pts',(2.686455836945,3.581291466659,-0.1149444397964));
#11730=CARTESIAN_POINT('Ctrl Pts',(2.094837206026,3.443708133325,1.685797813611));
#11731=CARTESIAN_POINT('Ctrl Pts',(0.4623025226986,3.306124799992,2.648874018616));
#11732=CARTESIAN_POINT('Ctrl Pts',(-1.399948395371,3.168541466659,2.295735540948));
#11733=CARTESIAN_POINT('Ctrl Pts',(-2.566570675924,3.030958133325,0.8018554526641));
#11734=CARTESIAN_POINT('Ctrl Pts',(-2.457874459731,2.893374799992,-1.090463349186));
#11735=CARTESIAN_POINT('Ctrl Pts',(-1.127870499672,2.755791466659,-2.440935314217));
#11736=CARTESIAN_POINT('Ctrl Pts',(0.7625678436463,2.618208133325,-2.578516685126));
#11737=CARTESIAN_POINT('Ctrl Pts',(2.274088823798,2.480624799992,-1.434842919896));
#11738=CARTESIAN_POINT('Ctrl Pts',(2.655626280814,2.343041466659,0.4217957222611));
#11739=CARTESIAN_POINT('Ctrl Pts',(1.717586697175,2.205458133325,2.06885590643));
#11740=CARTESIAN_POINT('Ctrl Pts',(-0.07388787752371,2.067874799992,2.687872294968));
#11741=CARTESIAN_POINT('Ctrl Pts',(-1.828747976278,1.930291466659,1.97143678412));
#11742=CARTESIAN_POINT('Ctrl Pts',(-2.674537063841,1.792708133325,0.2748766656669));
#11743=CARTESIAN_POINT('Ctrl Pts',(-2.353348315127,1.700985911103,-0.9459121298763));
#11744=CARTESIAN_POINT('Ctrl Pts',(-2.010291573953,1.655124799992,-1.428639859679));
#11745=CARTESIAN_POINT('Ctrl Pts',(2.404044642027,6.11768501526,-1.141524323672));
#11746=CARTESIAN_POINT('Ctrl Pts',(2.678156841681,6.071823904148,-0.5642453719883));
#11747=CARTESIAN_POINT('Ctrl Pts',(2.790729699461,5.980101681926,0.7932751493761));
#11748=CARTESIAN_POINT('Ctrl Pts',(1.574000908471,5.842518348593,2.437727064909));
#11749=CARTESIAN_POINT('Ctrl Pts',(-0.4251410311493,5.70493501526,2.870253664408));
#11750=CARTESIAN_POINT('Ctrl Pts',(-2.21295213902,5.567351681926,1.87673139824));
#11751=CARTESIAN_POINT('Ctrl Pts',(-2.901177800026,5.429768348593,-0.04937617316592));
#11752=CARTESIAN_POINT('Ctrl Pts',(-2.147814317805,5.29218501526,-1.95093683105));
#11753=CARTESIAN_POINT('Ctrl Pts',(-0.3272122117171,5.154601681926,-2.883088186116));
#11754=CARTESIAN_POINT('Ctrl Pts',(1.655980718345,5.017018348593,-2.382643927865));
#11755=CARTESIAN_POINT('Ctrl Pts',(2.816323482115,4.87943501526,-0.6982738654132));
#11756=CARTESIAN_POINT('Ctrl Pts',(2.577246639281,4.741851681926,1.333065691311));
#11757=CARTESIAN_POINT('Ctrl Pts',(1.057546459105,4.604268348593,2.702010333647));
#11758=CARTESIAN_POINT('Ctrl Pts',(-0.9876442353842,4.46668501526,2.728337080863));
#11759=CARTESIAN_POINT('Ctrl Pts',(-2.542078543486,4.329101681926,1.398964274111));
#11760=CARTESIAN_POINT('Ctrl Pts',(-2.833364405197,4.191518348593,-0.625548166661));
#11761=CARTESIAN_POINT('Ctrl Pts',(-1.716763065658,4.05393501526,-2.339228278286));
#11762=CARTESIAN_POINT('Ctrl Pts',(0.2528908298411,3.916351681926,-2.890555411972));
#11763=CARTESIAN_POINT('Ctrl Pts',(2.096884304816,3.778768348593,-2.005577366684));
#11764=CARTESIAN_POINT('Ctrl Pts',(2.898944532531,3.64118501526,-0.1240361187815));
#11765=CARTESIAN_POINT('Ctrl Pts',(2.260531061571,3.503601681926,1.819138169894));
#11766=CARTESIAN_POINT('Ctrl Pts',(0.4988689380713,3.366018348593,2.858390131722));
#11767=CARTESIAN_POINT('Ctrl Pts',(-1.510679122572,3.22843501526,2.477319709873));
#11768=CARTESIAN_POINT('Ctrl Pts',(-2.769576899795,3.090851681926,0.8652792457679));
#11769=CARTESIAN_POINT('Ctrl Pts',(-2.652283215936,2.953268348593,-1.176714956775));
#11770=CARTESIAN_POINT('Ctrl Pts',(-1.217080874162,2.81568501526,-2.634004246821));
#11771=CARTESIAN_POINT('Ctrl Pts',(0.8228841325514,2.678101681926,-2.78246779403));
#11772=CARTESIAN_POINT('Ctrl Pts',(2.45396081766,2.540518348593,-1.548333674601));
#11773=CARTESIAN_POINT('Ctrl Pts',(2.865676472823,2.40293501526,0.4551581999144));
#11774=CARTESIAN_POINT('Ctrl Pts',(1.853441436277,2.265351681926,2.232494737513));
#11775=CARTESIAN_POINT('Ctrl Pts',(-0.07973213466677,2.127768348593,2.900473027131));
#11776=CARTESIAN_POINT('Ctrl Pts',(-1.973395160382,1.99018501526,2.127370123848));
#11777=CARTESIAN_POINT('Ctrl Pts',(-2.886083028668,1.852601681926,0.2966183907052));
#11778=CARTESIAN_POINT('Ctrl Pts',(-2.539489440867,1.760879459704,-1.020730271999));
#11779=CARTESIAN_POINT('Ctrl Pts',(-2.169298183488,1.715018348593,-1.541639975322));
#11780=CARTESIAN_POINT('Ctrl Pts',(2.522021513594,6.235843307732,-1.197543860985));
#11781=CARTESIAN_POINT('Ctrl Pts',(2.809585584818,6.189982196621,-0.5919353335721));
#11782=CARTESIAN_POINT('Ctrl Pts',(2.92768287977,6.098259974399,0.8322045930226));
#11783=CARTESIAN_POINT('Ctrl Pts',(1.651243942889,5.960676641066,2.557356878692));
#11784=CARTESIAN_POINT('Ctrl Pts',(-0.4460045408999,5.823093307732,3.011109429734));
#11785=CARTESIAN_POINT('Ctrl Pts',(-2.321551274712,5.685509974399,1.968830727539));
#11786=CARTESIAN_POINT('Ctrl Pts',(-3.043551146479,5.547926641066,-0.0517992756068));
#11787=CARTESIAN_POINT('Ctrl Pts',(-2.253216858794,5.410343307732,-2.046677741984));
#11788=CARTESIAN_POINT('Ctrl Pts',(-0.3432699306139,5.272759974399,-3.024573796951));
#11789=CARTESIAN_POINT('Ctrl Pts',(1.737246856715,5.135176641066,-2.499570573799));
#11790=CARTESIAN_POINT('Ctrl Pts',(2.95453266007,4.997593307732,-0.7325411850372));
#11791=CARTESIAN_POINT('Ctrl Pts',(2.703723282204,4.860009974399,1.398484992228));
#11792=CARTESIAN_POINT('Ctrl Pts',(1.109444839277,4.722426641066,2.834609670836));
#11793=CARTESIAN_POINT('Ctrl Pts',(-1.03611221101,4.584843307732,2.862228385439));
#11794=CARTESIAN_POINT('Ctrl Pts',(-2.666829335795,4.447259974399,1.467617503593));
#11795=CARTESIAN_POINT('Ctrl Pts',(-2.972409854974,4.309676641066,-0.6562465216029));
#11796=CARTESIAN_POINT('Ctrl Pts',(-1.801012056782,4.172093307732,-2.45402433046));
#11797=CARTESIAN_POINT('Ctrl Pts',(0.2653012769813,4.034509974399,-3.032407471886));
#11798=CARTESIAN_POINT('Ctrl Pts',(2.199787489722,3.896926641066,-2.103999725101));
#11799=CARTESIAN_POINT('Ctrl Pts',(3.041208282885,3.759343307732,-0.1301231077663));
#11800=CARTESIAN_POINT('Ctrl Pts',(2.37146510084,3.621759974399,1.908411150304));
#11801=CARTESIAN_POINT('Ctrl Pts',(0.5233505951948,3.484176641066,2.998663702172));
#11802=CARTESIAN_POINT('Ctrl Pts',(-1.584814682997,3.346593307732,2.59889250604));
#11803=CARTESIAN_POINT('Ctrl Pts',(-2.905492020709,3.209009974399,0.9077422419465));
#11804=CARTESIAN_POINT('Ctrl Pts',(-2.782442228317,3.071426641066,-1.234461450704));
#11805=CARTESIAN_POINT('Ctrl Pts',(-1.276808298299,2.933843307732,-2.763266231105));
#11806=CARTESIAN_POINT('Ctrl Pts',(0.8632666171041,2.796259974399,-2.919015526896));
#11807=CARTESIAN_POINT('Ctrl Pts',(2.574387291926,2.658676641066,-1.624317106805));
#11808=CARTESIAN_POINT('Ctrl Pts',(3.006307615555,2.521093307732,0.4774947820042));
#11809=CARTESIAN_POINT('Ctrl Pts',(1.94439782638,2.383509974399,2.342052913063));
#11810=CARTESIAN_POINT('Ctrl Pts',(-0.0836449354721,2.245926641066,3.042811787328));
#11811=CARTESIAN_POINT('Ctrl Pts',(-2.0702381987,2.108343307732,2.231769379789));
#11812=CARTESIAN_POINT('Ctrl Pts',(-3.027715609383,1.970759974399,0.3111747384423));
#11813=CARTESIAN_POINT('Ctrl Pts',(-2.664113174709,1.879037752177,-1.070821922587));
#11814=CARTESIAN_POINT('Ctrl Pts',(-2.275755030715,1.833176641066,-1.617294918742));
#11815=CARTESIAN_POINT('Ctrl Pts',(2.585998917206,6.392208093593,-1.227922565736));
#11816=CARTESIAN_POINT('Ctrl Pts',(2.880857772614,6.346346982481,-0.6069512585133));
#11817=CARTESIAN_POINT('Ctrl Pts',(3.001950901767,6.254624760259,0.8533155505813));
#11818=CARTESIAN_POINT('Ctrl Pts',(1.693131888581,6.117041426926,2.622230652499));
#11819=CARTESIAN_POINT('Ctrl Pts',(-0.4573185651349,5.979458093593,3.087493775493));
#11820=CARTESIAN_POINT('Ctrl Pts',(-2.380443247722,5.841874760259,2.01877505887));
#11821=CARTESIAN_POINT('Ctrl Pts',(-3.120758457782,5.704291426926,-0.05311329420039));
#11822=CARTESIAN_POINT('Ctrl Pts',(-2.310375357889,5.566708093593,-2.09859685816));
#11823=CARTESIAN_POINT('Ctrl Pts',(-0.351977833691,5.429124760259,-3.101299700167));
#11824=CARTESIAN_POINT('Ctrl Pts',(1.781316482103,5.291541426926,-2.562978452993));
#11825=CARTESIAN_POINT('Ctrl Pts',(3.029481794112,5.153958093593,-0.7511239301902));
#11826=CARTESIAN_POINT('Ctrl Pts',(2.772310007078,5.016374760259,1.433961072947));
#11827=CARTESIAN_POINT('Ctrl Pts',(1.137588691296,4.878791426926,2.906516657361));
#11828=CARTESIAN_POINT('Ctrl Pts',(-1.062395796916,4.741208093593,2.934835989957));
#11829=CARTESIAN_POINT('Ctrl Pts',(-2.734480153149,4.603624760259,1.504847303921));
#11830=CARTESIAN_POINT('Ctrl Pts',(-3.04781248892,4.466041426926,-0.6728938611896));
#11831=CARTESIAN_POINT('Ctrl Pts',(-1.846699246461,4.328458093593,-2.516276814912));
#11832=CARTESIAN_POINT('Ctrl Pts',(0.2720313095305,4.190874760259,-3.109332095922));
#11833=CARTESIAN_POINT('Ctrl Pts',(2.255590618812,4.053291426926,-2.157372957203));
#11834=CARTESIAN_POINT('Ctrl Pts',(3.118356161574,3.915708093593,-0.1334240068824));
#11835=CARTESIAN_POINT('Ctrl Pts',(2.431623263287,3.778124760259,1.956822787462));
#11836=CARTESIAN_POINT('Ctrl Pts',(0.5366266961634,3.640541426926,3.074732330824));
#11837=CARTESIAN_POINT('Ctrl Pts',(-1.625017483837,3.502958093593,2.66481993525));
#11838=CARTESIAN_POINT('Ctrl Pts',(-2.979197115887,3.365374760259,0.9307694014992));
#11839=CARTESIAN_POINT('Ctrl Pts',(-2.853025856771,3.227791426926,-1.265776662747));
#11840=CARTESIAN_POINT('Ctrl Pts',(-1.309197744382,3.090208093593,-2.833363412276));
#11841=CARTESIAN_POINT('Ctrl Pts',(0.8851655408403,2.952624760259,-2.99306367974));
#11842=CARTESIAN_POINT('Ctrl Pts',(2.639693084894,2.815041426926,-1.665521985739));
#11843=CARTESIAN_POINT('Ctrl Pts',(3.08257015125,2.677458093593,0.4896076352159));
#11844=CARTESIAN_POINT('Ctrl Pts',(1.99372235587,2.539874760259,2.401464961569));
#11845=CARTESIAN_POINT('Ctrl Pts',(-0.08576679913106,2.402291426926,3.120000342931));
#11846=CARTESIAN_POINT('Ctrl Pts',(-2.122754984976,2.264708093593,2.288383809765));
#11847=CARTESIAN_POINT('Ctrl Pts',(-3.104521212555,2.127124760259,0.319068466441));
#11848=CARTESIAN_POINT('Ctrl Pts',(-2.731695089822,2.035402538037,-1.097986007416));
#11849=CARTESIAN_POINT('Ctrl Pts',(-2.33348526709,1.989541426926,-1.658321662257));
#11850=CARTESIAN_POINT('Ctrl Pts',(2.571274775611,6.501639428961,-1.220931029272));
#11851=CARTESIAN_POINT('Ctrl Pts',(2.864454765839,6.45577831785,-0.6034954039063));
#11852=CARTESIAN_POINT('Ctrl Pts',(2.984858415824,6.364056095628,0.848456948782));
#11853=CARTESIAN_POINT('Ctrl Pts',(1.6834915467,6.226472762294,2.607300214916));
#11854=CARTESIAN_POINT('Ctrl Pts',(-0.4547146880558,6.088889428961,3.069914226166));
#11855=CARTESIAN_POINT('Ctrl Pts',(-2.366889497484,5.951306095628,2.007280572303));
#11856=CARTESIAN_POINT('Ctrl Pts',(-3.102989506252,5.813722762294,-0.05281087811692));
#11857=CARTESIAN_POINT('Ctrl Pts',(-2.297220559686,5.676139428961,-2.08664788282));
#11858=CARTESIAN_POINT('Ctrl Pts',(-0.349973744893,5.538556095628,-3.083641542768));
#11859=CARTESIAN_POINT('Ctrl Pts',(1.771174035433,5.400972762294,-2.548385385147));
#11860=CARTESIAN_POINT('Ctrl Pts',(3.012232552977,5.263389428961,-0.7468471862867));
#11861=CARTESIAN_POINT('Ctrl Pts',(2.756525048771,5.125806095628,1.425796395948));
#11862=CARTESIAN_POINT('Ctrl Pts',(1.131111497181,4.988222762294,2.889967554217));
#11863=CARTESIAN_POINT('Ctrl Pts',(-1.05634673555,4.850639428961,2.918125642405));
#11864=CARTESIAN_POINT('Ctrl Pts',(-2.718910590186,4.713056095628,1.496279015422));
#11865=CARTESIAN_POINT('Ctrl Pts',(-3.03045887661,4.575472762294,-0.6690625430769));
#11866=CARTESIAN_POINT('Ctrl Pts',(-1.836184523888,4.437889428961,-2.50194965651));
#11867=CARTESIAN_POINT('Ctrl Pts',(0.2704824196632,4.300306095628,-3.091628203727));
#11868=CARTESIAN_POINT('Ctrl Pts',(2.242747753553,4.162722762294,-2.145089322943));
#11869=CARTESIAN_POINT('Ctrl Pts',(3.100600888221,4.025139428961,-0.1326643182543));
#11870=CARTESIAN_POINT('Ctrl Pts',(2.417778104653,3.887556095628,1.945681044282));
#11871=CARTESIAN_POINT('Ctrl Pts',(0.5335712550317,3.749972762294,3.057225442517));
#11872=CARTESIAN_POINT('Ctrl Pts',(-1.615764971251,3.612389428961,2.649647003123));
#11873=CARTESIAN_POINT('Ctrl Pts',(-2.962234185283,3.474806095628,0.9254697935337));
#11874=CARTESIAN_POINT('Ctrl Pts',(-2.836781319153,3.337222762294,-1.258569592904));
#11875=CARTESIAN_POINT('Ctrl Pts',(-1.301743443904,3.199639428961,-2.81723082854));
#11876=CARTESIAN_POINT('Ctrl Pts',(0.880125591801,3.062056095628,-2.976021795796));
#11877=CARTESIAN_POINT('Ctrl Pts',(2.624663219842,2.924472762294,-1.656038848919));
#11878=CARTESIAN_POINT('Ctrl Pts',(3.065018636018,2.786889428961,0.4868199108673));
#11879=CARTESIAN_POINT('Ctrl Pts',(1.982370514199,2.649306095628,2.387791518052));
#11880=CARTESIAN_POINT('Ctrl Pts',(-0.08527846076163,2.511722762294,3.10223570795));
#11881=CARTESIAN_POINT('Ctrl Pts',(-2.110668458271,2.374139428961,2.275354226878));
#11882=CARTESIAN_POINT('Ctrl Pts',(-3.086844712532,2.236556095628,0.3172517567559));
#11883=CARTESIAN_POINT('Ctrl Pts',(-2.716141384432,2.144833873405,-1.091734302771));
#11884=CARTESIAN_POINT('Ctrl Pts',(-2.320198885857,2.098972762294,-1.648879522586));
#11885=CARTESIAN_POINT('Ctrl Pts',(2.551614418722,6.552581420145,-1.211595605458));
#11886=CARTESIAN_POINT('Ctrl Pts',(2.842552710281,6.506720309034,-0.598880986523));
#11887=CARTESIAN_POINT('Ctrl Pts',(2.962035735699,6.414998086811,0.8419695182762));
#11888=CARTESIAN_POINT('Ctrl Pts',(1.670619315018,6.277414753478,2.587364402054));
#11889=CARTESIAN_POINT('Ctrl Pts',(-0.4512378705897,6.139831420145,3.046441196415));
#11890=CARTESIAN_POINT('Ctrl Pts',(-2.348791901428,6.002248086811,1.991932600627));
#11891=CARTESIAN_POINT('Ctrl Pts',(-3.079263577893,5.864664753478,-0.05240707813364));
#11892=CARTESIAN_POINT('Ctrl Pts',(-2.279655662895,5.727081420145,-2.07069305665));
#11893=CARTESIAN_POINT('Ctrl Pts',(-0.3472977925631,5.589498086811,-3.060063551872));
#11894=CARTESIAN_POINT('Ctrl Pts',(1.757631370145,5.451914753478,-2.528900044009));
#11895=CARTESIAN_POINT('Ctrl Pts',(2.989200566047,5.314331420145,-0.7411366794348));
#11896=CARTESIAN_POINT('Ctrl Pts',(2.735448240199,5.176748086811,1.414894540471));
#11897=CARTESIAN_POINT('Ctrl Pts',(1.122462847131,5.039164753478,2.86787042401));
#11898=CARTESIAN_POINT('Ctrl Pts',(-1.048269748206,4.901581420145,2.895813211186));
#11899=CARTESIAN_POINT('Ctrl Pts',(-2.698121387469,4.763998086811,1.484838239147));
#11900=CARTESIAN_POINT('Ctrl Pts',(-3.007287528446,4.626414753478,-0.6639467894038));
#11901=CARTESIAN_POINT('Ctrl Pts',(-1.822144778546,4.488831420145,-2.482819369995));
#11902=CARTESIAN_POINT('Ctrl Pts',(0.2684142700615,4.351248086811,-3.067989145611));
#11903=CARTESIAN_POINT('Ctrl Pts',(2.225599364098,4.213664753478,-2.12868764466));
#11904=CARTESIAN_POINT('Ctrl Pts',(3.076893223598,4.076081420145,-0.1316499467573));
#11905=CARTESIAN_POINT('Ctrl Pts',(2.399291406589,3.938498086811,1.930804071939));
#11906=CARTESIAN_POINT('Ctrl Pts',(0.5294914882953,3.800914753478,3.03384943313));
#11907=CARTESIAN_POINT('Ctrl Pts',(-1.603410587237,3.663331420145,2.629387400296));
#11908=CARTESIAN_POINT('Ctrl Pts',(-2.939584493455,3.525748086811,0.9183935111373));
#11909=CARTESIAN_POINT('Ctrl Pts',(-2.815090858966,3.388164753478,-1.248946378924));
#11910=CARTESIAN_POINT('Ctrl Pts',(-1.291790116112,3.250581420145,-2.795689854368));
#11911=CARTESIAN_POINT('Ctrl Pts',(0.8733960180478,3.112998086811,-2.953266681808));
#11912=CARTESIAN_POINT('Ctrl Pts',(2.604594646812,2.975414753478,-1.643376524728));
#11913=CARTESIAN_POINT('Ctrl Pts',(3.041583038692,2.837831420145,0.4830976119985));
#11914=CARTESIAN_POINT('Ctrl Pts',(1.967213008604,2.700248086811,2.369534101977));
#11915=CARTESIAN_POINT('Ctrl Pts',(-0.08462640871746,2.562664753478,3.078515543247));
#11916=CARTESIAN_POINT('Ctrl Pts',(-2.094529967139,2.425081420145,2.257956523383));
#11917=CARTESIAN_POINT('Ctrl Pts',(-3.063242229715,2.287498086811,0.3148260017099));
#11918=CARTESIAN_POINT('Ctrl Pts',(-2.695373355482,2.195775864589,-1.083386736722));
#11919=CARTESIAN_POINT('Ctrl Pts',(-2.302458293298,2.149914753478,-1.63627193969));
#11920=CARTESIAN_POINT('',(-2.80462878822583,2.1166580354494,-0.49452709968698));
#11921=CARTESIAN_POINT('Ctrl Pts',(2.8478481444634,6.34999057338997,3.43324101593387E-6));
#11922=CARTESIAN_POINT('Ctrl Pts',(2.84809696575054,6.34115918425508,0.13170913080596));
#11923=CARTESIAN_POINT('Ctrl Pts',(2.83938055714691,6.33232843183148,0.263538298043461));
#11924=CARTESIAN_POINT('Ctrl Pts',(2.82155635415381,6.32349742268422,0.394114480287347));
#11925=CARTESIAN_POINT('Ctrl Pts',(2.80378836361778,6.31469426402333,0.524278862461372));
#11926=CARTESIAN_POINT('Ctrl Pts',(2.77696985655664,6.30589085025552,0.653196924687804));
#11927=CARTESIAN_POINT('Ctrl Pts',(2.7410111732741,6.29708629637187,0.77950469363509));
#11928=CARTESIAN_POINT('Ctrl Pts',(2.71536342294656,6.29080639457517,0.869594480764798));
#11929=CARTESIAN_POINT('Ctrl Pts',(2.68506694171866,6.28452591276246,0.958356302134713));
#11930=CARTESIAN_POINT('Ctrl Pts',(2.65041891146736,6.27824452980137,1.04538327500442));
#11931=CARTESIAN_POINT('Ctrl Pts',(2.5997071381679,6.26905093159623,1.17275825381554));
#11932=CARTESIAN_POINT('Ctrl Pts',(2.53970189234722,6.25985740260528,1.29636375830609));
#11933=CARTESIAN_POINT('Ctrl Pts',(2.4712791398385,6.25066444347172,1.41511872849825));
#11934=CARTESIAN_POINT('Ctrl Pts',(2.40117573256152,6.24124567947012,1.53679065393686));
#11935=CARTESIAN_POINT('Ctrl Pts',(2.32223565051641,6.2318275136643,1.65337194442108));
#11936=CARTESIAN_POINT('Ctrl Pts',(2.23534963126661,6.22241048450276,1.7636827323246));
#11937=CARTESIAN_POINT('Ctrl Pts',(2.18637417655564,6.21710234299513,1.82586213752406));
#11938=CARTESIAN_POINT('Ctrl Pts',(2.1348731925072,6.21179456263259,1.88604881870501));
#11939=CARTESIAN_POINT('Ctrl Pts',(2.08100037887293,6.20648723984907,1.94402707460256));
#11940=CARTESIAN_POINT('Ctrl Pts',(1.9944833156645,6.19796394303658,2.03713727419703));
#11941=CARTESIAN_POINT('Ctrl Pts',(1.90176153167035,6.18944086409824,2.1246380745346));
#11942=CARTESIAN_POINT('Ctrl Pts',(1.80356554015024,6.18091740126049,2.20548528729524));
#11943=CARTESIAN_POINT('Ctrl Pts',(1.72132980638225,6.17377929704813,2.27319202116031));
#11944=CARTESIAN_POINT('Ctrl Pts',(1.6352558172579,6.16664092358867,2.33623234091894));
#11945=CARTESIAN_POINT('Ctrl Pts',(1.54579372034786,6.15950192742754,2.39401161664401));
#11946=CARTESIAN_POINT('Ctrl Pts',(1.44237556169335,6.15124924989005,2.46080444299466));
#11947=CARTESIAN_POINT('Ctrl Pts',(1.33442994880244,6.14299574021431,2.52056554350765));
#11948=CARTESIAN_POINT('Ctrl Pts',(1.22308284077281,6.13474085238257,2.57304695358816));
#11949=CARTESIAN_POINT('Ctrl Pts',(1.09978565476745,6.1256000272776,2.63116081298718));
#11950=CARTESIAN_POINT('Ctrl Pts',(0.972339627953733,6.11645960925327,2.68034830888395));
#11951=CARTESIAN_POINT('Ctrl Pts',(0.842080652999161,6.1073198587453,2.72037778091316));
#11952=CARTESIAN_POINT('Ctrl Pts',(0.709835318182901,6.09804073332239,2.76101767488489));
#11953=CARTESIAN_POINT('Ctrl Pts',(0.574689381761339,6.0887622959294,2.79221849312912));
#11954=CARTESIAN_POINT('Ctrl Pts',(0.438018273662977,6.07948481909915,2.8136898385709));
#11955=CARTESIAN_POINT('Ctrl Pts',(0.356995911669598,6.0739848776954,2.82641863800097));
#11956=CARTESIAN_POINT('Ctrl Pts',(0.275437198421243,6.06848527387585,2.83572713385917));
#11957=CARTESIAN_POINT('Ctrl Pts',(0.19362774091322,6.0629860644215,2.84154620372221));
#11958=CARTESIAN_POINT('Ctrl Pts',(0.0703208226356168,6.05469740695531,
2.85031696927805));
#11959=CARTESIAN_POINT('Ctrl Pts',(-0.0536460153404707,6.046408497496,2.85116138367029));
#11960=CARTESIAN_POINT('Ctrl Pts',(-0.177122198901636,6.03811907683254,
2.8438099188984));
#11961=CARTESIAN_POINT('Ctrl Pts',(-0.257570601659661,6.03271827294525,
2.83902022114639));
#11962=CARTESIAN_POINT('Ctrl Pts',(-0.337810365944785,6.02731725205642,
2.8307524461649));
#11963=CARTESIAN_POINT('Ctrl Pts',(-0.417522325443764,6.0219159424764,2.81894395536511));
#11964=CARTESIAN_POINT('Ctrl Pts',(-0.539700032319504,6.01363713936129,
2.80084460946207));
#11965=CARTESIAN_POINT('Ctrl Pts',(-0.66063668500771,6.00535765802631,2.77442476750783));
#11966=CARTESIAN_POINT('Ctrl Pts',(-0.779302709057901,5.99707724032767,
2.74024834526268));
#11967=CARTESIAN_POINT('Ctrl Pts',(-0.80720319833987,5.99513036710005,2.73221286155807));
#11968=CARTESIAN_POINT('Ctrl Pts',(-0.834978242685584,5.99318344210992,
2.72374880563183));
#11969=CARTESIAN_POINT('Ctrl Pts',(-0.862614625334214,5.99123646200206,
2.71486388828898));
#11970=CARTESIAN_POINT('Ctrl Pts',(-0.991268977026622,5.98217277712265,
2.67350235066958));
#11971=CARTESIAN_POINT('Ctrl Pts',(-1.11695009844818,5.97310986356814,2.62301486270993));
#11972=CARTESIAN_POINT('Ctrl Pts',(-1.23853382309703,5.96404772924091,2.56407752716352));
#11973=CARTESIAN_POINT('Ctrl Pts',(-1.36087184752588,5.95492937385326,2.50477454712509));
#11974=CARTESIAN_POINT('Ctrl Pts',(-1.47906260614583,5.9458118073915,2.43691597684037));
#11975=CARTESIAN_POINT('Ctrl Pts',(-1.59194254846901,5.93669503790605,2.361142032262));
#11976=CARTESIAN_POINT('Ctrl Pts',(-1.66297811258364,5.93095783739041,2.31345734366688));
#11977=CARTESIAN_POINT('Ctrl Pts',(-1.73191005931691,5.92522095249404,2.26263706352174));
#11978=CARTESIAN_POINT('Ctrl Pts',(-1.79844164777402,5.91948438522322,2.20883254135779));
#11979=CARTESIAN_POINT('Ctrl Pts',(-1.89364470256363,5.91127567202618,2.13184122053871));
#11980=CARTESIAN_POINT('Ctrl Pts',(-1.98397218151525,5.90306626998173,2.04870013519556));
#11981=CARTESIAN_POINT('Ctrl Pts',(-2.068411895023,5.89485622416037,1.95995768846063));
#11982=CARTESIAN_POINT('Ctrl Pts',(-2.10449982580334,5.8913474064134,1.92203085117033));
#11983=CARTESIAN_POINT('Ctrl Pts',(-2.13951267118782,5.88783847107766,1.88308144487671));
#11984=CARTESIAN_POINT('Ctrl Pts',(-2.17337325061447,5.88432942167148,1.84315455464047));
#11985=CARTESIAN_POINT('Ctrl Pts',(-2.25261903776763,5.87611699923038,1.74971144471963));
#11986=CARTESIAN_POINT('Ctrl Pts',(-2.32555045296493,5.86790395199546,1.65091252666336));
#11987=CARTESIAN_POINT('Ctrl Pts',(-2.39177095388154,5.85969032506734,1.54783633976085));
#11988=CARTESIAN_POINT('Ctrl Pts',(-2.4239061599349,5.85570445075158,1.4978159614874));
#11989=CARTESIAN_POINT('Ctrl Pts',(-2.45446166492524,5.85171843992237,1.44678875290166));
#11990=CARTESIAN_POINT('Ctrl Pts',(-2.48339614733578,5.84773229773376,1.39487982678156));
#11991=CARTESIAN_POINT('Ctrl Pts',(-2.54955855534775,5.83861747196516,1.27618340426768));
#11992=CARTESIAN_POINT('Ctrl Pts',(-2.60728825313002,5.82950370458883,1.15281098055722));
#11993=CARTESIAN_POINT('Ctrl Pts',(-2.65617001320165,5.8203907802979,1.026027535649));
#11994=CARTESIAN_POINT('Ctrl Pts',(-2.70494098821188,5.81129850943425,0.899531431288816));
#11995=CARTESIAN_POINT('Ctrl Pts',(-2.74490449140401,5.80220707783884,0.769638550200807));
#11996=CARTESIAN_POINT('Ctrl Pts',(-2.77560145945706,5.79311627166539,0.637585044842814));
#11997=CARTESIAN_POINT('Ctrl Pts',(-2.79488703263908,5.78740491256833,0.554621556816175));
#11998=CARTESIAN_POINT('Ctrl Pts',(-2.81051409637919,5.7816938003293,0.47080491634668));
#11999=CARTESIAN_POINT('Ctrl Pts',(-2.82235825676456,5.77598288191934,0.386440773001788));
#12000=CARTESIAN_POINT('Ctrl Pts',(-2.83958163538217,5.76767825695407,0.263761280720222));
#12001=CARTESIAN_POINT('Ctrl Pts',(-2.84880240909353,5.75937251212854,0.139905880303724));
#12002=CARTESIAN_POINT('Ctrl Pts',(-2.84961906389546,5.7510660046385,0.0159905663491347));
#12003=CARTESIAN_POINT('Ctrl Pts',(-2.84976071832129,5.74962518344168,-0.00550340222553886));
#12004=CARTESIAN_POINT('Ctrl Pts',(-2.84964964004326,5.74818433929835,-0.026999149914304));
#12005=CARTESIAN_POINT('Ctrl Pts',(-2.84928389354478,5.74674347407265,-0.0484908313339417));
#12006=CARTESIAN_POINT('Ctrl Pts',(-2.84717139437973,5.73842124378764,-0.1726236917816));
#12007=CARTESIAN_POINT('Ctrl Pts',(-2.83655873600505,5.730098310184,-0.296620339600148));
#12008=CARTESIAN_POINT('Ctrl Pts',(-2.81787179531194,5.72177503245665,-0.419370041283346));
#12009=CARTESIAN_POINT('Ctrl Pts',(-2.8047403931637,5.71592622559071,-0.505626840769667));
#12010=CARTESIAN_POINT('Ctrl Pts',(-2.78762313245978,5.71007724879857,-0.591267886240161));
#12011=CARTESIAN_POINT('Ctrl Pts',(-2.76668249612696,5.70422822671777,-0.675912222910682));
#12012=CARTESIAN_POINT('Ctrl Pts',(-2.73335868244143,5.69492040440685,-0.810610713439508));
#12013=CARTESIAN_POINT('Ctrl Pts',(-2.69033017548373,5.68561390947412,-0.942904815438035));
#12014=CARTESIAN_POINT('Ctrl Pts',(-2.63814095147965,5.67630828772023,-1.07148137412761));
#12015=CARTESIAN_POINT('Ctrl Pts',(-2.58654876642552,5.6671091212499,-1.19858703120764));
#12016=CARTESIAN_POINT('Ctrl Pts',(-2.52600370630068,5.65791080809458,-1.32206085512863));
#12017=CARTESIAN_POINT('Ctrl Pts',(-2.45698549554103,5.64871290946517,-1.44061470392629));
#12018=CARTESIAN_POINT('Ctrl Pts',(-2.41638579800083,5.64330228090425,-1.51035355039066));
#12019=CARTESIAN_POINT('Ctrl Pts',(-2.37285328242831,5.6378917957832,-1.57838946707628));
#12020=CARTESIAN_POINT('Ctrl Pts',(-2.32647920766074,5.63248136478523,-1.64445463159885));
#12021=CARTESIAN_POINT('Ctrl Pts',(-2.25985477999425,5.62470833922137,-1.73936873602186));
#12022=CARTESIAN_POINT('Ctrl Pts',(-2.18737469347683,5.61693403277976,-1.83019474974451));
#12023=CARTESIAN_POINT('Ctrl Pts',(-2.10939700128704,5.60915897176398,-1.91604133255032));
#12024=CARTESIAN_POINT('Ctrl Pts',(-2.02300955965761,5.60054538484182,-2.01114631005047));
#12025=CARTESIAN_POINT('Ctrl Pts',(-1.92987476389789,5.59193087181,-2.1001385814422));
#12026=CARTESIAN_POINT('Ctrl Pts',(-1.8311472911516,5.58331614827954,-2.18241178621735));
#12027=CARTESIAN_POINT('Ctrl Pts',(-1.74484421292693,5.57578554774807,-2.25433128977591));
#12028=CARTESIAN_POINT('Ctrl Pts',(-1.654268601442,5.56825478636485,-2.32111677068052));
#12029=CARTESIAN_POINT('Ctrl Pts',(-1.56020840510456,5.5607243421452,-2.38239123466756));
#12030=CARTESIAN_POINT('Ctrl Pts',(-1.43943537989252,5.55105527313395,-2.46106747256751));
#12031=CARTESIAN_POINT('Ctrl Pts',(-1.31278466650881,5.54138780920491,-2.5307545227796));
#12032=CARTESIAN_POINT('Ctrl Pts',(-1.18168851433157,5.5317212023782,-2.59072682747743));
#12033=CARTESIAN_POINT('Ctrl Pts',(-1.05343463133871,5.52226417530075,-2.64939888475589));
#12034=CARTESIAN_POINT('Ctrl Pts',(-0.920924786554568,5.51280796856319,
-2.6987732923217));
#12035=CARTESIAN_POINT('Ctrl Pts',(-0.785483990431386,5.50335188178882,
-2.73812465054624));
#12036=CARTESIAN_POINT('Ctrl Pts',(-0.716865969063655,5.49856116892452,
-2.75806112771405));
#12037=CARTESIAN_POINT('Ctrl Pts',(-0.647495507787036,5.49377048685132,
-2.77542419804366));
#12038=CARTESIAN_POINT('Ctrl Pts',(-0.577544734694411,5.48897974449455,
-2.79011435409674));
#12039=CARTESIAN_POINT('Ctrl Pts',(-0.492851432512891,5.48317932554051,
-2.80790054530938));
#12040=CARTESIAN_POINT('Ctrl Pts',(-0.407339492713478,5.47737808128343,
-2.82176053702046));
#12041=CARTESIAN_POINT('Ctrl Pts',(-0.321359348342017,5.47157630891338,
-2.83151871774004));
#12042=CARTESIAN_POINT('Ctrl Pts',(-0.185517346254951,5.46240995567958,
-2.84693589126732));
#12043=CARTESIAN_POINT('Ctrl Pts',(-0.0485070604358834,5.45324228419315,
-2.85211158994836));
#12044=CARTESIAN_POINT('Ctrl Pts',(0.0881700098645867,5.44407446649292,
-2.84741519824236));
#12045=CARTESIAN_POINT('Ctrl Pts',(0.22162178721207,5.43512299011284,-2.84282963155654));
#12046=CARTESIAN_POINT('Ctrl Pts',(0.354754767946376,5.42617137433824,-2.82883289177504));
#12047=CARTESIAN_POINT('Ctrl Pts',(0.486182151957727,5.41722071017753,-2.80581552730152));
#12048=CARTESIAN_POINT('Ctrl Pts',(0.637663211695356,5.40690432061671,-2.77928608833381));
#12049=CARTESIAN_POINT('Ctrl Pts',(0.787088749257628,5.39658988396729,-2.74074587821702));
#12050=CARTESIAN_POINT('Ctrl Pts',(0.932540277416806,5.38627621170946,-2.69066540502931));
#12051=CARTESIAN_POINT('Ctrl Pts',(1.07298509277952,5.37631755528078,-2.64230879510475));
#12052=CARTESIAN_POINT('Ctrl Pts',(1.2097258874806,5.36635961152581,-2.58319216877987));
#12053=CARTESIAN_POINT('Ctrl Pts',(1.34101116849616,5.35640131048165,-2.51369800567432));
#12054=CARTESIAN_POINT('Ctrl Pts',(1.38901313964186,5.35276024671819,-2.48828878396734));
#12055=CARTESIAN_POINT('Ctrl Pts',(1.43628546270362,5.34911913519016,-2.46149186313972));
#12056=CARTESIAN_POINT('Ctrl Pts',(1.48274123461023,5.34547792359802,-2.43332471124822));
#12057=CARTESIAN_POINT('Ctrl Pts',(1.53157103395927,5.34165063531641,-2.40371813452701));
#12058=CARTESIAN_POINT('Ctrl Pts',(1.57947953162742,5.33782297139469,-2.37260912009654));
#12059=CARTESIAN_POINT('Ctrl Pts',(1.62636044473214,5.33399503167055,-2.34002601055496));
#12060=CARTESIAN_POINT('Ctrl Pts',(1.75117389214106,5.32380371239363,-2.25327833522488));
#12061=CARTESIAN_POINT('Ctrl Pts',(1.86870088347843,5.31361043819798,-2.15607963389188));
#12062=CARTESIAN_POINT('Ctrl Pts',(1.97776383319767,5.30341709312524,-2.05014842743312));
#12063=CARTESIAN_POINT('Ctrl Pts',(2.08369263963999,5.29351667433051,-1.94726136730815));
#12064=CARTESIAN_POINT('Ctrl Pts',(2.18163634605226,5.28361618867375,-1.83613768070385));
#12065=CARTESIAN_POINT('Ctrl Pts',(2.27055708134304,5.27371736239433,-1.71837496386946));
#12066=CARTESIAN_POINT('Ctrl Pts',(2.37798703845376,5.2617580541501,-1.57609944649558));
#12067=CARTESIAN_POINT('Ctrl Pts',(2.47243782432304,5.24980145815805,-1.42389682933471));
#12068=CARTESIAN_POINT('Ctrl Pts',(2.55208901765524,5.23784528967073,-1.26431845019061));
#12069=CARTESIAN_POINT('Ctrl Pts',(2.62502815371991,5.2268966451668,-1.11818744295228));
#12070=CARTESIAN_POINT('Ctrl Pts',(2.68555690314024,5.21594835915329,-0.965870248777373));
#12071=CARTESIAN_POINT('Ctrl Pts',(2.73222929239438,5.20499867717148,-0.809323905587983));
#12072=CARTESIAN_POINT('Ctrl Pts',(2.73652421232884,5.20399105771656,-0.794918086199347));
#12073=CARTESIAN_POINT('Ctrl Pts',(2.74070175754344,5.20298342644034,-0.780476458486443));
#12074=CARTESIAN_POINT('Ctrl Pts',(2.74476077843502,5.20197578197562,-0.76600055127141));
#12075=CARTESIAN_POINT('Ctrl Pts',(2.75222850003782,5.20012193383388,-0.739368009109834));
#12076=CARTESIAN_POINT('Ctrl Pts',(2.75929326713199,5.1982680033424,-0.712625755318726));
#12077=CARTESIAN_POINT('Ctrl Pts',(2.76594836371704,5.19641400225846,-0.685783942329835));
#12078=CARTESIAN_POINT('Ctrl Pts',(2.81024179225335,5.18407457735774,-0.50713650871018));
#12079=CARTESIAN_POINT('Ctrl Pts',(2.83638460267271,5.17173202545407,-0.324080379512753));
#12080=CARTESIAN_POINT('Ctrl Pts',(2.84485026731554,5.15938981280454,-0.140202555747719));
#12081=CARTESIAN_POINT('Ctrl Pts',(2.85152140085033,5.14966387253007,0.00469729183389342));
#12082=CARTESIAN_POINT('Ctrl Pts',(2.84721632851365,5.1399381429254,0.150107288936105));
#12083=CARTESIAN_POINT('Ctrl Pts',(2.83218569049158,5.1302143201883,0.294285196709865));
#12084=CARTESIAN_POINT('Ctrl Pts',(2.81110865098778,5.11657887798971,0.49646180779319));
#12085=CARTESIAN_POINT('Ctrl Pts',(2.76890298599158,5.1029469832523,0.696619041135436));
#12086=CARTESIAN_POINT('Ctrl Pts',(2.70601952727829,5.08931459937678,0.890024566844041));
#12087=CARTESIAN_POINT('Ctrl Pts',(2.65915327878379,5.07915455564898,1.03416726531414));
#12088=CARTESIAN_POINT('Ctrl Pts',(2.60080132238486,5.06899424022782,1.17455881312527));
#12089=CARTESIAN_POINT('Ctrl Pts',(2.53114783776104,5.05883198207297,1.30922135465441));
#12090=CARTESIAN_POINT('Ctrl Pts',(2.53032809415689,5.05871238366133,1.31080618214344));
#12091=CARTESIAN_POINT('Ctrl Pts',(2.52950678519412,5.05859278498061,1.31239021592857));
#12092=CARTESIAN_POINT('Ctrl Pts',(2.52868391319439,5.05847318602808,1.31397345381782));
#12093=CARTESIAN_POINT('Ctrl Pts',(2.43719290793056,5.04517557911134,1.49000572385092));
#12094=CARTESIAN_POINT('Ctrl Pts',(2.32655093361843,5.0318746244084,1.65587647992433));
#12095=CARTESIAN_POINT('Ctrl Pts',(2.20012636487033,5.01857424917523,1.80870322130724));
#12096=CARTESIAN_POINT('Ctrl Pts',(2.09916138403714,5.00795232541635,1.93075346175748));
#12097=CARTESIAN_POINT('Ctrl Pts',(1.98812917464779,4.99733077123822,2.04448488234765));
#12098=CARTESIAN_POINT('Ctrl Pts',(1.86872280618781,4.98671158699582,2.14843627152901));
#12099=CARTESIAN_POINT('Ctrl Pts',(1.73420524933564,4.97474851719918,2.26554298103214));
#12100=CARTESIAN_POINT('Ctrl Pts',(1.58882199632064,4.96278798301116,2.37043814307767));
#12101=CARTESIAN_POINT('Ctrl Pts',(1.4349635770105,4.95082703617151,2.4608589775063));
#12102=CARTESIAN_POINT('Ctrl Pts',(1.30815421469591,4.94096888184876,2.53538339030905));
#12103=CARTESIAN_POINT('Ctrl Pts',(1.17558913257157,4.93111044721276,2.60007530364507));
#12104=CARTESIAN_POINT('Ctrl Pts',(1.03863029203751,4.92125008160984,2.65367989990671));
#12105=CARTESIAN_POINT('Ctrl Pts',(1.00955535153907,4.91915682832236,2.66505959938922));
#12106=CARTESIAN_POINT('Ctrl Pts',(0.980282458753524,4.91706348801221,2.67593968041636));
#12107=CARTESIAN_POINT('Ctrl Pts',(0.95082918475627,4.91497004488722,2.68631959875166));
#12108=CARTESIAN_POINT('Ctrl Pts',(0.799276180692962,4.90419814922434,2.73972988535656));
#12109=CARTESIAN_POINT('Ctrl Pts',(0.643155172613163,4.89342481534808,2.77982888277722));
#12110=CARTESIAN_POINT('Ctrl Pts',(0.484778766588518,4.88265174521157,2.80666919304322));
#12111=CARTESIAN_POINT('Ctrl Pts',(0.318147226613579,4.87131714486192,2.8349085144503));
#12112=CARTESIAN_POINT('Ctrl Pts',(0.149017878869776,4.8599828364626,2.84847134663192));
#12113=CARTESIAN_POINT('Ctrl Pts',(-0.019946453562988,4.848650802215,2.84737147468315));
#12114=CARTESIAN_POINT('Ctrl Pts',(-0.0469929580676308,4.84683685775162,
2.84719541568189));
#12115=CARTESIAN_POINT('Ctrl Pts',(-0.074035272357364,4.84502297155914,
2.84664355083377));
#12116=CARTESIAN_POINT('Ctrl Pts',(-0.101062509484977,4.84320915176765,
2.84571582061425));
#12117=CARTESIAN_POINT('Ctrl Pts',(-0.250363679354825,4.83318942923648,
2.840590945791));
#12118=CARTESIAN_POINT('Ctrl Pts',(-0.399415580182845,4.82317115084706,
2.82398464559706));
#12119=CARTESIAN_POINT('Ctrl Pts',(-0.546236844382753,4.81315266285064,
2.79581809727281));
#12120=CARTESIAN_POINT('Ctrl Pts',(-0.690256359088589,4.8033253548841,2.76818904338405));
#12121=CARTESIAN_POINT('Ctrl Pts',(-0.832128210659078,4.79349784523402,
2.72943686342525));
#12122=CARTESIAN_POINT('Ctrl Pts',(-0.969978395291538,4.78366857303063,
2.67953573585256));
#12123=CARTESIAN_POINT('Ctrl Pts',(-1.02701636231628,4.77960153673822,2.65888825629657));
#12124=CARTESIAN_POINT('Ctrl Pts',(-1.08336587223442,4.77553419869001,2.6363326080126));
#12125=CARTESIAN_POINT('Ctrl Pts',(-1.13892524763199,4.77146644831613,2.61195352742645));
#12126=CARTESIAN_POINT('Ctrl Pts',(-1.27332233275196,4.76162663659521,2.55298098957416));
#12127=CARTESIAN_POINT('Ctrl Pts',(-1.40296756560452,4.75178622629293,2.4834005734629));
#12128=CARTESIAN_POINT('Ctrl Pts',(-1.52659117388361,4.74194620226236,2.40439336973659));
#12129=CARTESIAN_POINT('Ctrl Pts',(-1.65471235135068,4.73174818682945,2.32251179298352));
#12130=CARTESIAN_POINT('Ctrl Pts',(-1.77636691693109,4.72155058628551,2.23050444652182));
#12131=CARTESIAN_POINT('Ctrl Pts',(-1.89012498891916,4.71135449693192,2.12963331895248));
#12132=CARTESIAN_POINT('Ctrl Pts',(-1.93344485021052,4.70747175552471,2.09122089530429));
#12133=CARTESIAN_POINT('Ctrl Pts',(-1.97561935365505,4.70358923326113,2.05152261794535));
#12134=CARTESIAN_POINT('Ctrl Pts',(-2.01656839967359,4.69970699068146,2.01060656280138));
#12135=CARTESIAN_POINT('Ctrl Pts',(-2.11229311203592,4.6906316497299,1.91495897169792));
#12136=CARTESIAN_POINT('Ctrl Pts',(-2.2014321872198,4.68155709368734,1.81253895656524));
#12137=CARTESIAN_POINT('Ctrl Pts',(-2.2828146653471,4.67248228155625,1.70429494526024));
#12138=CARTESIAN_POINT('Ctrl Pts',(-2.36171617245722,4.66368411799132,1.59935078744963));
#12139=CARTESIAN_POINT('Ctrl Pts',(-2.43332607264819,4.65488571371377,1.48893324423344));
#12140=CARTESIAN_POINT('Ctrl Pts',(-2.49660877287086,4.64608612005862,1.37394121389828));
#12141=CARTESIAN_POINT('Ctrl Pts',(-2.54004957872659,4.64004558388936,1.2950042145735));
#12142=CARTESIAN_POINT('Ctrl Pts',(-2.57956713284195,4.63400448725897,1.21391235616628));
#12143=CARTESIAN_POINT('Ctrl Pts',(-2.6150947154906,4.62796252329951,1.13110423363072));
#12144=CARTESIAN_POINT('Ctrl Pts',(-2.67021293955555,4.61858889586747,1.00263400537312));
#12145=CARTESIAN_POINT('Ctrl Pts',(-2.7157020102016,4.60921522696859,0.870109166010463));
#12146=CARTESIAN_POINT('Ctrl Pts',(-2.75141516065125,4.59984209210928,0.735000743640519));
#12147=CARTESIAN_POINT('Ctrl Pts',(-2.78803267481489,4.59023160145956,0.596470972184675));
#12148=CARTESIAN_POINT('Ctrl Pts',(-2.81437326800116,4.58062167223881,0.455223899761565));
#12149=CARTESIAN_POINT('Ctrl Pts',(-2.83023010740115,4.57101292479062,0.312821329313767));
#12150=CARTESIAN_POINT('Ctrl Pts',(-2.83837622524724,4.56607663281642,0.239665002810554));
#12151=CARTESIAN_POINT('Ctrl Pts',(-2.84375468353297,4.56114065273264,0.166203453674323));
#12152=CARTESIAN_POINT('Ctrl Pts',(-2.84633213932709,4.5562050686467,0.0926477277248243));
#12153=CARTESIAN_POINT('Ctrl Pts',(-2.85080369569687,4.54764246109071,-0.0349620554002695));
#12154=CARTESIAN_POINT('Ctrl Pts',(-2.84684405950869,4.53908011868222,-0.162981422032098));
#12155=CARTESIAN_POINT('Ctrl Pts',(-2.834239387605,4.53051741032784,-0.290140302708813));
#12156=CARTESIAN_POINT('Ctrl Pts',(-2.82343743161624,4.52317933762787,-0.399112963254424));
#12157=CARTESIAN_POINT('Ctrl Pts',(-2.80628716758326,4.51584099617165,-0.507452912356721));
#12158=CARTESIAN_POINT('Ctrl Pts',(-2.78268445247893,4.5085019887619,-0.614359082965291));
#12159=CARTESIAN_POINT('Ctrl Pts',(-2.75691231571862,4.50048842329653,-0.731091435038663));
#12160=CARTESIAN_POINT('Ctrl Pts',(-2.72344676688929,4.4924740638305,-0.846113502585519));
#12161=CARTESIAN_POINT('Ctrl Pts',(-2.68285940366929,4.48445839326727,-0.958539835166529));
#12162=CARTESIAN_POINT('Ctrl Pts',(-2.63657534198002,4.47531767158949,-1.08674592937551));
#12163=CARTESIAN_POINT('Ctrl Pts',(-2.58104650664304,4.46617733297043,-1.21155651494625));
#12164=CARTESIAN_POINT('Ctrl Pts',(-2.51705937033925,4.45703765854587,-1.33186684914844));
#12165=CARTESIAN_POINT('Ctrl Pts',(-2.45204500968134,4.44775125937788,-1.45410859820187));
#12166=CARTESIAN_POINT('Ctrl Pts',(-2.37829801534487,4.438465545901,-1.57170557119922));
#12167=CARTESIAN_POINT('Ctrl Pts',(-2.29659335178013,4.42918081300935,-1.68348107768699));
#12168=CARTESIAN_POINT('Ctrl Pts',(-2.24825681646411,4.42368795862703,-1.74960754441592));
#12169=CARTESIAN_POINT('Ctrl Pts',(-2.19713426300355,4.41819544744109,-1.81369612736419));
#12170=CARTESIAN_POINT('Ctrl Pts',(-2.14337940984177,4.41270334051083,-1.87549783130719));
#12171=CARTESIAN_POINT('Ctrl Pts',(-2.06216813859641,4.40440602483816,-1.96886605105165));
#12172=CARTESIAN_POINT('Ctrl Pts',(-1.97488330498467,4.39610851128944,-2.05708156164466));
#12173=CARTESIAN_POINT('Ctrl Pts',(-1.88215307563072,4.38781050185156,-2.13913975278296));
#12174=CARTESIAN_POINT('Ctrl Pts',(-1.81922503464678,4.38217935565867,-2.19482559817551));
#12175=CARTESIAN_POINT('Ctrl Pts',(-1.75379029273467,4.37654798110035,-2.24767632393704));
#12176=CARTESIAN_POINT('Ctrl Pts',(-1.68605559554002,4.37091628504346,-2.297386871109));
#12177=CARTESIAN_POINT('Ctrl Pts',(-1.58640436084932,4.36263093811323,-2.37052099007613));
#12178=CARTESIAN_POINT('Ctrl Pts',(-1.48177429550487,4.35434489532274,-2.436856127471));
#12179=CARTESIAN_POINT('Ctrl Pts',(-1.37329667206734,4.34605786010788,-2.49606869218833));
#12180=CARTESIAN_POINT('Ctrl Pts',(-1.35102808158013,4.34435667429918,-2.50822401338364));
#12181=CARTESIAN_POINT('Ctrl Pts',(-1.32859742487597,4.3426554466687,-2.52007934135439));
#12182=CARTESIAN_POINT('Ctrl Pts',(-1.30601458666857,4.34095417465092,-2.53163212802679));
#12183=CARTESIAN_POINT('Ctrl Pts',(-1.1857521478759,4.33189423630173,-2.59315523186848));
#12184=CARTESIAN_POINT('Ctrl Pts',(-1.06115273222554,4.32283502699286,-2.64611431941297));
#12185=CARTESIAN_POINT('Ctrl Pts',(-0.933490708804636,4.31377658423978,
-2.69020099239149));
#12186=CARTESIAN_POINT('Ctrl Pts',(-0.804885285362792,4.30465120117936,
-2.73461345817117));
#12187=CARTESIAN_POINT('Ctrl Pts',(-0.673170621020409,4.29552659604602,
-2.77002228964768));
#12188=CARTESIAN_POINT('Ctrl Pts',(-0.539627852568289,4.28640280719315,
-2.79606489591989));
#12189=CARTESIAN_POINT('Ctrl Pts',(-0.455700474782248,4.28066879641315,
-2.81243184472943));
#12190=CARTESIAN_POINT('Ctrl Pts',(-0.371050677151256,4.27493510804125,
-2.82509843252094));
#12191=CARTESIAN_POINT('Ctrl Pts',(-0.285995403583839,4.26920175159779,
-2.83396412656041));
#12192=CARTESIAN_POINT('Ctrl Pts',(-0.164183522195132,4.26099072709857,
-2.84666112729261));
#12193=CARTESIAN_POINT('Ctrl Pts',(-0.041479910489348,4.25277906620465,
-2.8515628186172));
#12194=CARTESIAN_POINT('Ctrl Pts',(0.0810094029847688,4.24456677723678,
-2.84834577334894));
#12195=CARTESIAN_POINT('Ctrl Pts',(0.13687525607919,4.2408212543333,-2.84687851899624));
#12196=CARTESIAN_POINT('Ctrl Pts',(0.192696365280209,4.23707560078048,-2.84372312835945));
#12197=CARTESIAN_POINT('Ctrl Pts',(0.248367412713555,4.2333298173677,-2.83885251761691));
#12198=CARTESIAN_POINT('Ctrl Pts',(0.370431291058467,4.22511684362492,-2.82817325677034));
#12199=CARTESIAN_POINT('Ctrl Pts',(0.491772856086867,4.21690324558581,-2.80924474939128));
#12200=CARTESIAN_POINT('Ctrl Pts',(0.611351618208173,4.20868903157138,-2.78255509152167));
#12201=CARTESIAN_POINT('Ctrl Pts',(0.665887443384615,4.20494280664393,-2.77038284212073));
#12202=CARTESIAN_POINT('Ctrl Pts',(0.720056775219937,4.20119645359587,-2.75659701156376));
#12203=CARTESIAN_POINT('Ctrl Pts',(0.773762155636671,4.19744997321655,-2.74124726262043));
#12204=CARTESIAN_POINT('Ctrl Pts',(0.904265963911871,4.1883460444605,-2.70394744875398));
#12205=CARTESIAN_POINT('Ctrl Pts',(1.03210179914571,4.17924314089706,-2.65739809823362));
#12206=CARTESIAN_POINT('Ctrl Pts',(1.15608961781954,4.17014107439263,-2.60220541100469));
#12207=CARTESIAN_POINT('Ctrl Pts',(1.27992336361626,4.16105031852814,-2.5470813087078));
#12208=CARTESIAN_POINT('Ctrl Pts',(1.39991978605433,4.15196039764364,-2.48333477778042));
#12209=CARTESIAN_POINT('Ctrl Pts',(1.51488473647243,4.14287112430601,-2.41152225575072));
#12210=CARTESIAN_POINT('Ctrl Pts',(1.58728265227502,4.13714725417506,-2.36629910813426));
#12211=CARTESIAN_POINT('Ctrl Pts',(1.65768480452553,4.13142364084257,-2.31787630256474));
#12212=CARTESIAN_POINT('Ctrl Pts',(1.72578611389249,4.12570023749965,-2.2663846186789));
#12213=CARTESIAN_POINT('Ctrl Pts',(1.82435957315917,4.11741587892366,-2.19185281523377));
#12214=CARTESIAN_POINT('Ctrl Pts',(1.91812685833765,4.10913045284344,-2.11087324313886));
#12215=CARTESIAN_POINT('Ctrl Pts',(2.00602383790393,4.10084427739672,-2.02395239693411));
#12216=CARTESIAN_POINT('Ctrl Pts',(2.02405849606512,4.09914412407652,-2.00611802132622));
#12217=CARTESIAN_POINT('Ctrl Pts',(2.04184612028,4.09744393920902,-1.98803367128797));
#12218=CARTESIAN_POINT('Ctrl Pts',(2.05937768551325,4.09574372554221,-1.96970393933037));
#12219=CARTESIAN_POINT('Ctrl Pts',(2.14496407303129,4.0874435456202,-1.88022102542318));
#12220=CARTESIAN_POINT('Ctrl Pts',(2.22444454601499,4.07914267934137,-1.78488749043672));
#12221=CARTESIAN_POINT('Ctrl Pts',(2.29734399251735,4.07084144642509,-1.68478489258555));
#12222=CARTESIAN_POINT('Ctrl Pts',(2.34680041128402,4.06520972669216,-1.61687332073572));
#12223=CARTESIAN_POINT('Ctrl Pts',(2.39322871986781,4.05957783821317,-1.54676757298662));
#12224=CARTESIAN_POINT('Ctrl Pts',(2.43649261093021,4.05394588081884,-1.47481174068824));
#12225=CARTESIAN_POINT('Ctrl Pts',(2.50775104962519,4.04466968117841,-1.3562958111528));
#12226=CARTESIAN_POINT('Ctrl Pts',(2.57049079385341,4.03539477674111,-1.23266463282099));
#12227=CARTESIAN_POINT('Ctrl Pts',(2.62418232290552,4.02612074408822,-1.10522080479152));
#12228=CARTESIAN_POINT('Ctrl Pts',(2.67732164753879,4.01694209262305,-0.979087705777112));
#12229=CARTESIAN_POINT('Ctrl Pts',(2.72159833392014,4.00776429510233,-0.849218780956081));
#12230=CARTESIAN_POINT('Ctrl Pts',(2.75645283976302,3.99858694103764,-0.71685792494221));
#12231=CARTESIAN_POINT('Ctrl Pts',(2.77720016500195,3.99312407346834,-0.63806943943041));
#12232=CARTESIAN_POINT('Ctrl Pts',(2.79460803017755,3.98766136302824,-0.558397714916988));
#12233=CARTESIAN_POINT('Ctrl Pts',(2.80854958934038,3.98219872313878,-0.478104491334957));
#12234=CARTESIAN_POINT('Ctrl Pts',(2.8289977693348,3.97418663192289,-0.360337872195623));
#12235=CARTESIAN_POINT('Ctrl Pts',(2.84198145600201,3.96617321355946,-0.24125180620398));
#12236=CARTESIAN_POINT('Ctrl Pts',(2.84709160218678,3.95815901551443,-0.121817505725509));
#12237=CARTESIAN_POINT('Ctrl Pts',(2.85255389365086,3.94959255107487,0.00584713172955927));
#12238=CARTESIAN_POINT('Ctrl Pts',(2.84901944856095,3.94102519579393,0.13390865241372));
#12239=CARTESIAN_POINT('Ctrl Pts',(2.83687638457245,3.93245761829523,0.261142010808346));
#12240=CARTESIAN_POINT('Ctrl Pts',(2.82647528994478,3.92511909283096,0.37012325324529));
#12241=CARTESIAN_POINT('Ctrl Pts',(2.80975935061011,3.91778040433192,0.478496429154096));
#12242=CARTESIAN_POINT('Ctrl Pts',(2.7870018996455,3.91044197297679,0.585499256888617));
#12243=CARTESIAN_POINT('Ctrl Pts',(2.75718958450986,3.90082861036861,0.725673216871521));
#12244=CARTESIAN_POINT('Ctrl Pts',(2.71698441767795,3.8912168171005,0.863652500268121));
#12245=CARTESIAN_POINT('Ctrl Pts',(2.6668868192048,3.88160588597332,0.997942599994107));
#12246=CARTESIAN_POINT('Ctrl Pts',(2.6178084021306,3.87219047883392,1.12950071304055));
#12247=CARTESIAN_POINT('Ctrl Pts',(2.55923541270253,3.86277589911363,1.25751936135917));
#12248=CARTESIAN_POINT('Ctrl Pts',(2.49159411524659,3.8533614819027,1.3805726182506));
#12249=CARTESIAN_POINT('Ctrl Pts',(2.45647354948705,3.8484733488955,1.4444640597682));
#12250=CARTESIAN_POINT('Ctrl Pts',(2.41890760236793,3.84358525969874,1.50701644777642));
#12251=CARTESIAN_POINT('Ctrl Pts',(2.37895180791164,3.83869712124206,1.56802637965971));
#12252=CARTESIAN_POINT('Ctrl Pts',(2.32958431699072,3.83265756842715,1.64340736755695));
#12253=CARTESIAN_POINT('Ctrl Pts',(2.27658552809973,3.82661713171428,1.71640518801221));
#12254=CARTESIAN_POINT('Ctrl Pts',(2.22009732330164,3.82057613731894,1.78659955199873));
#12255=CARTESIAN_POINT('Ctrl Pts',(2.13518671489279,3.81149557773424,1.89211266175804));
#12256=CARTESIAN_POINT('Ctrl Pts',(2.04239038531967,3.80241375807755,1.99128929097583));
#12257=CARTESIAN_POINT('Ctrl Pts',(1.94300077141682,3.79333178629112,2.08335525699706));
#12258=CARTESIAN_POINT('Ctrl Pts',(1.84671862500594,3.78453376703233,2.17254273315104));
#12259=CARTESIAN_POINT('Ctrl Pts',(1.74425017248423,3.77573560500794,2.25505686398576));
#12260=CARTESIAN_POINT('Ctrl Pts',(1.63679510037212,3.76693830745429,2.33023339542586));
#12261=CARTESIAN_POINT('Ctrl Pts',(1.51201676441845,3.7567227622217,2.41752943749707));
#12262=CARTESIAN_POINT('Ctrl Pts',(1.38035145290207,3.74650912030626,2.49505664498431));
#12263=CARTESIAN_POINT('Ctrl Pts',(1.24344279684043,3.73629626040805,2.56183339412736));
#12264=CARTESIAN_POINT('Ctrl Pts',(1.11100607355229,3.72641698951877,2.62642897268857));
#12265=CARTESIAN_POINT('Ctrl Pts',(0.973661763850657,3.716538450394,2.68096532304448));
#12266=CARTESIAN_POINT('Ctrl Pts',(0.832885022088923,3.70665962806103,2.72450770689853));
#12267=CARTESIAN_POINT('Ctrl Pts',(0.778429129104624,3.7028382575346,2.74135096783613));
#12268=CARTESIAN_POINT('Ctrl Pts',(0.723459584799259,3.69901684463083,2.75654863331248));
#12269=CARTESIAN_POINT('Ctrl Pts',(0.66806180137864,3.69519533060128,2.77004446035488));
#12270=CARTESIAN_POINT('Ctrl Pts',(0.609112947181974,3.6911288524964,2.78440538766031));
#12271=CARTESIAN_POINT('Ctrl Pts',(0.54970265226331,3.68706195029126,2.79683335328153));
#12272=CARTESIAN_POINT('Ctrl Pts',(0.489945752046593,3.68299474226145,2.8072625801369));
#12273=CARTESIAN_POINT('Ctrl Pts',(0.342616168957259,3.67296711262878,2.83297565492781));
#12274=CARTESIAN_POINT('Ctrl Pts',(0.193179931634859,3.66293762400927,2.84653552760749));
#12275=CARTESIAN_POINT('Ctrl Pts',(0.0435912834424511,3.65290804896259,
2.84831532521404));
#12276=CARTESIAN_POINT('Ctrl Pts',(-0.102943903755338,3.64308320145753,
2.85005879290761));
#12277=CARTESIAN_POINT('Ctrl Pts',(-0.249624082421185,3.63325827101767,
2.84049861746464));
#12278=CARTESIAN_POINT('Ctrl Pts',(-0.394624710814754,3.62343492385677,
2.82003242443467));
#12279=CARTESIAN_POINT('Ctrl Pts',(-0.571154976497794,3.61147554062221,
2.7951159634984));
#12280=CARTESIAN_POINT('Ctrl Pts',(-0.745496729775374,3.59951886296536,
2.75400322734476));
#12281=CARTESIAN_POINT('Ctrl Pts',(-0.914569285802567,3.58756265879809,
2.69722852032646));
#12282=CARTESIAN_POINT('Ctrl Pts',(-1.06695640580188,3.57678638876359,2.64605679680953));
#12283=CARTESIAN_POINT('Ctrl Pts',(-1.21506381218767,3.56601050337461,2.58216093989508));
#12284=CARTESIAN_POINT('Ctrl Pts',(-1.35660426622524,3.55523336831249,2.5058952187549));
#12285=CARTESIAN_POINT('Ctrl Pts',(-1.37210206020685,3.55405333946462,2.49754459954765));
#12286=CARTESIAN_POINT('Ctrl Pts',(-1.38752108339747,3.55287329563457,2.48904564691914));
#12287=CARTESIAN_POINT('Ctrl Pts',(-1.40285830175433,3.55169323467695,2.48039880218197));
#12288=CARTESIAN_POINT('Ctrl Pts',(-1.4300617271585,3.54960017585195,2.46506200574888));
#12289=CARTESIAN_POINT('Ctrl Pts',(-1.45700064554427,3.54750701042459,2.44926397377593));
#12290=CARTESIAN_POINT('Ctrl Pts',(-1.48365784997017,3.5454137553533,2.43300829364778));
#12291=CARTESIAN_POINT('Ctrl Pts',(-1.63619964879767,3.53343542150859,2.33998763595633));
#12292=CARTESIAN_POINT('Ctrl Pts',(-1.779513195613,3.52145415224934,2.23197927270628));
#12293=CARTESIAN_POINT('Ctrl Pts',(-1.91158903059991,3.50947312524184,2.11162428747825));
#12294=CARTESIAN_POINT('Ctrl Pts',(-2.02014920877862,3.49962527967019,2.01269810130387));
#12295=CARTESIAN_POINT('Ctrl Pts',(-2.12111753814876,3.48977759776559,1.90543133827463));
#12296=CARTESIAN_POINT('Ctrl Pts',(-2.21340374161109,3.4799318441425,1.7912975705709));
#12297=CARTESIAN_POINT('Ctrl Pts',(-2.33818722219613,3.46661904808004,1.63697321598664));
#12298=CARTESIAN_POINT('Ctrl Pts',(-2.44734366893353,3.45330963601978,1.4697973896561));
#12299=CARTESIAN_POINT('Ctrl Pts',(-2.53808343374277,3.43999992429471,1.29318656076566));
#12300=CARTESIAN_POINT('Ctrl Pts',(-2.61036500647599,3.42939766079826,1.15250172980146));
#12301=CARTESIAN_POINT('Ctrl Pts',(-2.67095976199367,3.41879520715212,1.00583019415891));
#12302=CARTESIAN_POINT('Ctrl Pts',(-2.71843656738083,3.40819070139704,0.854910070656629));
#12303=CARTESIAN_POINT('Ctrl Pts',(-2.71897202898103,3.40807109971839,0.853207935684107));
#12304=CARTESIAN_POINT('Ctrl Pts',(-2.71950581296388,3.4079514977575,0.851505288330626));
#12305=CARTESIAN_POINT('Ctrl Pts',(-2.72003791742379,3.40783189551727,0.849802131157961));
#12306=CARTESIAN_POINT('Ctrl Pts',(-2.78064313378115,3.39420953338379,0.655817271573425));
#12307=CARTESIAN_POINT('Ctrl Pts',(-2.81946197667226,3.38058354759009,0.455223171462301));
#12308=CARTESIAN_POINT('Ctrl Pts',(-2.83688305988526,3.36695824880052,0.252781415767838));
#12309=CARTESIAN_POINT('Ctrl Pts',(-2.84989568282765,3.35678087501392,0.101568187380142));
#12310=CARTESIAN_POINT('Ctrl Pts',(-2.85096951908672,3.34660388452721,-0.0506770999019837));
#12311=CARTESIAN_POINT('Ctrl Pts',(-2.84026065611321,3.33642907378275,-0.201987989379743));
#12312=CARTESIAN_POINT('Ctrl Pts',(-2.82729090711349,3.32410612765842,-0.385244070095902));
#12313=CARTESIAN_POINT('Ctrl Pts',(-2.79701034081176,3.31178591434536,-0.567458903452159));
#12314=CARTESIAN_POINT('Ctrl Pts',(-2.74953742834339,3.2994652189085,-0.745047684255998));
#12315=CARTESIAN_POINT('Ctrl Pts',(-2.71201735900181,3.28972759542826,-0.885404427156217));
#12316=CARTESIAN_POINT('Ctrl Pts',(-2.66375909072285,3.27998967079027,-1.02287042766145));
#12317=CARTESIAN_POINT('Ctrl Pts',(-2.60484225061453,3.27024985781717,-1.15566723149896));
#12318=CARTESIAN_POINT('Ctrl Pts',(-2.59362723400801,3.26839585200089,-1.18094554509474));
#12319=CARTESIAN_POINT('Ctrl Pts',(-2.58202606365812,3.26654177776194,-1.2060546646842));
#12320=CARTESIAN_POINT('Ctrl Pts',(-2.57004711808163,3.26468762415302,-1.23098575734892));
#12321=CARTESIAN_POINT('Ctrl Pts',(-2.49934599096278,3.25374419435236,-1.37813195986286));
#12322=CARTESIAN_POINT('Ctrl Pts',(-2.41558860934539,3.24279918690502,-1.51887089551128));
#12323=CARTESIAN_POINT('Ctrl Pts',(-2.32053943933346,3.2318544370577,-1.65153069994788));
#12324=CARTESIAN_POINT('Ctrl Pts',(-2.22030733295526,3.22031288092584,-1.79142431110442));
#12325=CARTESIAN_POINT('Ctrl Pts',(-2.10751788126752,3.20877161125327,-1.92233476579457));
#12326=CARTESIAN_POINT('Ctrl Pts',(-1.98418459168677,3.19723278017763,-2.04229092572904));
#12327=CARTESIAN_POINT('Ctrl Pts',(-1.96884192219244,3.19579734881805,-2.05721348006891));
#12328=CARTESIAN_POINT('Ctrl Pts',(-1.95333602220956,3.19436195519667,-2.07196648687955));
#12329=CARTESIAN_POINT('Ctrl Pts',(-1.93767071885483,3.19292660345666,-2.0865461270179));
#12330=CARTESIAN_POINT('Ctrl Pts',(-1.82653568299889,3.18274372582708,-2.18997909558875));
#12331=CARTESIAN_POINT('Ctrl Pts',(-1.70721454429739,3.17256239098252,-2.28483266857398));
#12332=CARTESIAN_POINT('Ctrl Pts',(-1.58112343764028,3.16238084259267,-2.36958986849931));
#12333=CARTESIAN_POINT('Ctrl Pts',(-1.45847682856542,3.15247742895588,-2.45203171107739));
#12334=CARTESIAN_POINT('Ctrl Pts',(-1.32942616321843,3.14257381328154,-2.5249204589247));
#12335=CARTESIAN_POINT('Ctrl Pts',(-1.19531110992135,3.13266837927901,-2.58689025716349));
#12336=CARTESIAN_POINT('Ctrl Pts',(-1.1434844665379,3.12884058081056,-2.61083750659531));
#12337=CARTESIAN_POINT('Ctrl Pts',(-1.09090186043034,3.12501251080862,-2.63315460308598));
#12338=CARTESIAN_POINT('Ctrl Pts',(-1.0376728971373,3.12118407600231,-2.65383209561131));
#12339=CARTESIAN_POINT('Ctrl Pts',(-0.899746226006865,3.1112638514515,-2.70741152934259));
#12340=CARTESIAN_POINT('Ctrl Pts',(-0.757621948601878,3.10134294670043,
-2.74993223899868));
#12341=CARTESIAN_POINT('Ctrl Pts',(-0.613079557174189,3.0914224103428,-2.78133826411903));
#12342=CARTESIAN_POINT('Ctrl Pts',(-0.463051255015121,3.08112535346184,
-2.81393626239366));
#12343=CARTESIAN_POINT('Ctrl Pts',(-0.310416588733038,3.0708286934687,-2.83456026641949));
#12344=CARTESIAN_POINT('Ctrl Pts',(-0.157139282858265,3.06053360293976,
-2.84309887830231));
#12345=CARTESIAN_POINT('Ctrl Pts',(-0.10200333405594,3.05683031770076,-2.84617033408585));
#12346=CARTESIAN_POINT('Ctrl Pts',(-0.0467840851091486,3.05312723554094,
-2.84767753954083));
#12347=CARTESIAN_POINT('Ctrl Pts',(0.0084273585641129,3.04942441103761,
-2.84761369930359));
#12348=CARTESIAN_POINT('Ctrl Pts',(0.145022335917836,3.04026349809047,-2.84745575639935));
#12349=CARTESIAN_POINT('Ctrl Pts',(0.281736206132755,3.03110343981126,-2.83767675257286));
#12350=CARTESIAN_POINT('Ctrl Pts',(0.417030580383158,3.02194313588785,-2.81812304454695));
#12351=CARTESIAN_POINT('Ctrl Pts',(0.549244980840984,3.0129913661047,-2.7990144763031));
#12352=CARTESIAN_POINT('Ctrl Pts',(0.680102565697361,3.00403936173425,-2.77057126889529));
#12353=CARTESIAN_POINT('Ctrl Pts',(0.808165230425777,2.99508609591237,-2.73269807790536));
#12354=CARTESIAN_POINT('Ctrl Pts',(0.891144568989746,2.98928474797492,-2.70815780815293));
#12355=CARTESIAN_POINT('Ctrl Pts',(0.972950471700694,2.98348287041621,-2.67965937474857));
#12356=CARTESIAN_POINT('Ctrl Pts',(1.05326830465212,2.977680183882,-2.64743662252163));
#12357=CARTESIAN_POINT('Ctrl Pts',(1.18358736308271,2.96826508118665,-2.59515385322933));
#12358=CARTESIAN_POINT('Ctrl Pts',(1.30991012635984,2.95884987814422,-2.53310462897821));
#12359=CARTESIAN_POINT('Ctrl Pts',(1.43108061450185,2.94943519183428,-2.46224537776815));
#12360=CARTESIAN_POINT('Ctrl Pts',(1.55546616618113,2.93977070200258,-2.38950599057501));
#12361=CARTESIAN_POINT('Ctrl Pts',(1.67442352860711,2.93010675668848,-2.30748226668282));
#12362=CARTESIAN_POINT('Ctrl Pts',(1.78668491565101,2.92044402340607,-2.21715735664828));
#12363=CARTESIAN_POINT('Ctrl Pts',(1.84292582065231,2.91560317047436,-2.17190622606571));
#12364=CARTESIAN_POINT('Ctrl Pts',(1.89748577612663,2.91076262174164,-2.12457090221474));
#12365=CARTESIAN_POINT('Ctrl Pts',(1.95020241061681,2.90592246113963,-2.07527108311025));
#12366=CARTESIAN_POINT('Ctrl Pts',(2.04397384324838,2.89731286763642,-1.98757742226459));
#12367=CARTESIAN_POINT('Ctrl Pts',(2.13200436224271,2.88870359842508,-1.89357535354423));
#12368=CARTESIAN_POINT('Ctrl Pts',(2.21323285300151,2.88009397817898,-1.79402779742342));
#12369=CARTESIAN_POINT('Ctrl Pts',(2.2842772396131,2.87256379777517,-1.70696111678932));
#12370=CARTESIAN_POINT('Ctrl Pts',(2.35011819774215,2.86503334884133,-1.61565336536314));
#12371=CARTESIAN_POINT('Ctrl Pts',(2.41006756861768,2.85750217954432,-1.52063939005921));
#12372=CARTESIAN_POINT('Ctrl Pts',(2.47195337799855,2.84972774420458,-1.42255634634576));
#12373=CARTESIAN_POINT('Ctrl Pts',(2.52756038400556,2.84195254121281,-1.32052427569478));
#12374=CARTESIAN_POINT('Ctrl Pts',(2.57669081111168,2.83417607352209,-1.21548324525062));
#12375=CARTESIAN_POINT('Ctrl Pts',(2.63456575396471,2.82501550542389,-1.09174640858425));
#12376=CARTESIAN_POINT('Ctrl Pts',(2.68344801398981,2.81585527377479,-0.963865763740706));
#12377=CARTESIAN_POINT('Ctrl Pts',(2.72311848058956,2.80669569192513,-0.833190120338741));
#12378=CARTESIAN_POINT('Ctrl Pts',(2.76346867605783,2.79737916631502,-0.700275430743322));
#12379=CARTESIAN_POINT('Ctrl Pts',(2.79428908464733,2.78806331296295,-0.564467934780335));
#12380=CARTESIAN_POINT('Ctrl Pts',(2.81530111786789,2.77874846160411,-0.427164010794746));
#12381=CARTESIAN_POINT('Ctrl Pts',(2.82757907739632,2.77330551532677,-0.346933220937656));
#12382=CARTESIAN_POINT('Ctrl Pts',(2.83650712469226,2.76786291117145,-0.266191152347382));
#12383=CARTESIAN_POINT('Ctrl Pts',(2.84202147888127,2.76242071492505,-0.185215426013762));
#12384=CARTESIAN_POINT('Ctrl Pts',(2.85045103785572,2.75410146073187,-0.0614312733763999));
#12385=CARTESIAN_POINT('Ctrl Pts',(2.85090464794611,2.74578206280165,0.0629964521132601));
#12386=CARTESIAN_POINT('Ctrl Pts',(2.84311949965228,2.73746218504955,0.186903956485225));
#12387=CARTESIAN_POINT('Ctrl Pts',(2.83764713126289,2.7316139424348,0.274001527981754));
#12388=CARTESIAN_POINT('Ctrl Pts',(2.82810498296568,2.72576546273895,0.360841618066086));
#12389=CARTESIAN_POINT('Ctrl Pts',(2.81441718411854,2.71991662923419,0.447018804472821));
#12390=CARTESIAN_POINT('Ctrl Pts',(2.79498016771151,2.71161113950106,0.569392562650119));
#12391=CARTESIAN_POINT('Ctrl Pts',(2.76718158097466,2.7033049363225,0.690428490885676));
#12392=CARTESIAN_POINT('Ctrl Pts',(2.73160210686119,2.69499768545555,0.809094381998766));
#12393=CARTESIAN_POINT('Ctrl Pts',(2.72542648768954,2.69355577494406,0.829691520389315));
#12394=CARTESIAN_POINT('Ctrl Pts',(2.71901656920653,2.69211383286841,0.850217300525002));
#12395=CARTESIAN_POINT('Ctrl Pts',(2.7123755330958,2.69067185748077,0.870666388989825));
#12396=CARTESIAN_POINT('Ctrl Pts',(2.67064740764895,2.68161138425584,0.999155696156249));
#12397=CARTESIAN_POINT('Ctrl Pts',(2.61979265389133,2.67255160135519,1.12463777940907));
#12398=CARTESIAN_POINT('Ctrl Pts',(2.56050167822933,2.66349257395265,1.24599674437055));
#12399=CARTESIAN_POINT('Ctrl Pts',(2.50071299431134,2.65435750204791,1.36837443702413));
#12400=CARTESIAN_POINT('Ctrl Pts',(2.43234529298495,2.64522319837834,1.48656062936928));
#12401=CARTESIAN_POINT('Ctrl Pts',(2.35605753556705,2.63608972977292,1.5993931294019));
#12402=CARTESIAN_POINT('Ctrl Pts',(2.30824860094078,2.63036585718514,1.67010436538998));
#12403=CARTESIAN_POINT('Ctrl Pts',(2.25732817701152,2.62464231256294,1.73871255946905));
#12404=CARTESIAN_POINT('Ctrl Pts',(2.20345030717718,2.61891911235483,1.80492507141801));
#12405=CARTESIAN_POINT('Ctrl Pts',(2.12615843289759,2.61070874931855,1.89991192158544));
#12406=CARTESIAN_POINT('Ctrl Pts',(2.04273521956806,2.60249780250347,1.99001459206904));
#12407=CARTESIAN_POINT('Ctrl Pts',(1.95373829132842,2.59428624309621,2.07422470903276));
#12408=CARTESIAN_POINT('Ctrl Pts',(1.91054670840689,2.59030104657237,2.11509317855876));
#12409=CARTESIAN_POINT('Ctrl Pts',(1.86604300917947,2.58631570576403,2.15457416437758));
#12410=CARTESIAN_POINT('Ctrl Pts',(1.8202943955014,2.58233021737761,2.19255519697283));
#12411=CARTESIAN_POINT('Ctrl Pts',(1.72604711272271,2.57411966364129,2.27080039024623));
#12412=CARTESIAN_POINT('Ctrl Pts',(1.62651467735229,2.56590848357433,2.34267673037767));
#12413=CARTESIAN_POINT('Ctrl Pts',(1.52277917244175,2.55769664838017,2.40780009086491));
#12414=CARTESIAN_POINT('Ctrl Pts',(1.47844499771388,2.55418709842765,2.43563232096971));
#12415=CARTESIAN_POINT('Ctrl Pts',(1.4333434682952,2.55067742881538,2.46223167461521));
#12416=CARTESIAN_POINT('Ctrl Pts',(1.38756025028133,2.54716763729551,2.4875707972306));
#12417=CARTESIAN_POINT('Ctrl Pts',(1.26891421197317,2.53807210235528,2.55323648529147));
#12418=CARTESIAN_POINT('Ctrl Pts',(1.14563385239945,2.52897755889248,2.61047602220136));
#12419=CARTESIAN_POINT('Ctrl Pts',(1.0189814365323,2.51988384752141,2.65889309143623));
#12420=CARTESIAN_POINT('Ctrl Pts',(0.892334871035826,2.5107905562101,2.70730792417368));
#12421=CARTESIAN_POINT('Ctrl Pts',(0.762315362595673,2.50169809691366,2.7469015143793));
#12422=CARTESIAN_POINT('Ctrl Pts',(0.630164154549595,2.49260631026847,2.77723091893705));
#12423=CARTESIAN_POINT('Ctrl Pts',(0.546879651692226,2.48687647289487,2.79634515495426));
#12424=CARTESIAN_POINT('Ctrl Pts',(0.462748127960112,2.48114690268412,2.81177890098223));
#12425=CARTESIAN_POINT('Ctrl Pts',(0.378079282353485,2.4754175597458,2.82341062940693));
#12426=CARTESIAN_POINT('Ctrl Pts',(0.255750957563129,2.46713988784921,2.84021598257331));
#12427=CARTESIAN_POINT('Ctrl Pts',(0.132273370076185,2.45886120387561,2.84908296321122));
#12428=CARTESIAN_POINT('Ctrl Pts',(0.00875639082543048,2.45058178679057,
2.84962297824459));
#12429=CARTESIAN_POINT('Ctrl Pts',(-0.0202735153242608,2.44863589479733,
2.84974989671226));
#12430=CARTESIAN_POINT('Ctrl Pts',(-0.0493055530627788,2.44668996230848,
2.84941707206123));
#12431=CARTESIAN_POINT('Ctrl Pts',(-0.0783252583048325,2.44474399294569,
2.84861987761965));
#12432=CARTESIAN_POINT('Ctrl Pts',(-0.201972236186597,2.43645261890334,
2.84522319654853));
#12433=CARTESIAN_POINT('Ctrl Pts',(-0.325394706421818,2.42816057543787,
2.83339201024013));
#12434=CARTESIAN_POINT('Ctrl Pts',(-0.447496781829693,2.41986814269175,
2.81355910618427));
#12435=CARTESIAN_POINT('Ctrl Pts',(-0.527029194075716,2.41446678339885,
2.80064074508239));
#12436=CARTESIAN_POINT('Ctrl Pts',(-0.606001457979839,2.4090652589459,2.78432861551543));
#12437=CARTESIAN_POINT('Ctrl Pts',(-0.684114254614127,2.40366364675096,
2.76475364718617));
#12438=CARTESIAN_POINT('Ctrl Pts',(-0.818136932673682,2.39439578587031,
2.73116773307915));
#12439=CARTESIAN_POINT('Ctrl Pts',(-0.949739937308827,2.38512918943378,
2.68795570610072));
#12440=CARTESIAN_POINT('Ctrl Pts',(-1.07763376262398,2.37586345593199,2.63566953190969));
#12441=CARTESIAN_POINT('Ctrl Pts',(-1.20431846106865,2.36668532202559,2.58387767883239));
#12442=CARTESIAN_POINT('Ctrl Pts',(-1.32736492605692,2.35750803481446,2.52318189258877));
#12443=CARTESIAN_POINT('Ctrl Pts',(-1.44550074330027,2.3483312040696,2.45407242604945));
#12444=CARTESIAN_POINT('Ctrl Pts',(-1.51594067256431,2.34285940623877,2.41286505940909));
#12445=CARTESIAN_POINT('Ctrl Pts',(-1.58463427958763,2.33738777069478,2.36866554426707));
#12446=CARTESIAN_POINT('Ctrl Pts',(-1.65130600877161,2.33191621471365,2.32157107421747));
#12447=CARTESIAN_POINT('Ctrl Pts',(-1.75184851670552,2.32366498188413,2.25055152535383));
#12448=CARTESIAN_POINT('Ctrl Pts',(-1.84777688142223,2.31541235096666,2.17295356714672));
#12449=CARTESIAN_POINT('Ctrl Pts',(-1.9380254250103,2.30715890415833,2.08921697074446));
#12450=CARTESIAN_POINT('Ctrl Pts',(-2.03126753674888,2.2986316883282,2.00270280920868));
#12451=CARTESIAN_POINT('Ctrl Pts',(-2.11844575454504,2.29010360158284,1.90963650255824));
#12452=CARTESIAN_POINT('Ctrl Pts',(-2.19898427330714,2.28157528599718,1.81115156281633));
#12453=CARTESIAN_POINT('Ctrl Pts',(-2.26639938968078,2.27443662245438,1.72871431693944));
#12454=CARTESIAN_POINT('Ctrl Pts',(-2.32916283406357,2.26729779857235,1.64248150554385));
#12455=CARTESIAN_POINT('Ctrl Pts',(-2.38696115341166,2.26015919092189,1.55313203489346));
#12456=CARTESIAN_POINT('Ctrl Pts',(-2.46323386771049,2.2507388308153,1.43522330113557));
#12457=CARTESIAN_POINT('Ctrl Pts',(-2.53094821808017,2.24131998429432,1.31176553557256));
#12458=CARTESIAN_POINT('Ctrl Pts',(-2.58945805705541,2.23190201879764,1.18408840259321));
#12459=CARTESIAN_POINT('Ctrl Pts',(-2.64684412511343,2.2226649397281,1.05886350416706));
#12460=CARTESIAN_POINT('Ctrl Pts',(-2.69537627053228,2.21342870816502,0.929578579642012));
#12461=CARTESIAN_POINT('Ctrl Pts',(-2.73439894914873,2.20419272729932,0.797471141416176));
#12462=CARTESIAN_POINT('Ctrl Pts',(-2.75662093382076,2.19893317484148,0.722240799179309));
#12463=CARTESIAN_POINT('Ctrl Pts',(-2.77575823263306,2.19367370368192,0.646094931826458));
#12464=CARTESIAN_POINT('Ctrl Pts',(-2.79168214922777,2.18841420360768,0.56926171586123));
#12465=CARTESIAN_POINT('Ctrl Pts',(-2.81069174901636,2.18213553523456,0.477540016787891));
#12466=CARTESIAN_POINT('Ctrl Pts',(-2.82511457512874,2.17585595672354,0.384865577083334));
#12467=CARTESIAN_POINT('Ctrl Pts',(-2.83472867179422,2.1695758005696,0.291690675508813));
#12468=CARTESIAN_POINT('Ctrl Pts',(-2.84825497168096,2.16074010040666,0.160600703724005));
#12469=CARTESIAN_POINT('Ctrl Pts',(-2.85226036880898,2.15190325683758,0.028520551691609));
#12470=CARTESIAN_POINT('Ctrl Pts',(-2.84707363368557,2.14306619583182,-0.103208249395973));
#12471=CARTESIAN_POINT('Ctrl Pts',(-2.84190671011819,2.13426288937977,-0.234433891470715));
#12472=CARTESIAN_POINT('Ctrl Pts',(-2.827618090831,2.12545936714896,-0.365309681728793));
#12473=CARTESIAN_POINT('Ctrl Pts',(-2.80458334954684,2.11665654453875,-0.494518897726551));
#12474=CARTESIAN_POINT('',(-2.11596363778888,2.11666666302544,-0.373098825439504));
#12475=CARTESIAN_POINT('Ctrl Pts',(-2.11596363778888,2.11666666302544,-0.373098825439504));
#12476=CARTESIAN_POINT('Ctrl Pts',(-2.11596363651329,2.11665130912368,-0.37309881786039));
#12477=CARTESIAN_POINT('Ctrl Pts',(-2.1159636365634,2.11663595520812,-0.373098810515882));
#12478=CARTESIAN_POINT('Ctrl Pts',(-2.11596363793934,2.11662060127888,-0.373098803405978));
#12479=CARTESIAN_POINT('Ctrl Pts',(-2.11596683312042,2.08096600528101,-0.373082292924252));
#12480=CARTESIAN_POINT('Ctrl Pts',(-2.12311934727396,2.0452337361124,-0.374330868757299));
#12481=CARTESIAN_POINT('Ctrl Pts',(-2.13605487204922,2.01089616470858,-0.376602271121508));
#12482=CARTESIAN_POINT('Ctrl Pts',(-2.14744386484174,1.98066388886159,-0.378602111530333));
#12483=CARTESIAN_POINT('Ctrl Pts',(-2.16331663724392,1.95151252630738,-0.38139500483258));
#12484=CARTESIAN_POINT('Ctrl Pts',(-2.18273341382768,1.92448634192568,-0.384814546287745));
#12485=CARTESIAN_POINT('Ctrl Pts',(-2.19478368808634,1.90771358190755,-0.386936752937024));
#12486=CARTESIAN_POINT('Ctrl Pts',(-2.20819877256644,1.89176014158068,-0.389300287494568));
#12487=CARTESIAN_POINT('Ctrl Pts',(-2.22275031585101,1.87688528762621,-0.391864731679025));
#12488=CARTESIAN_POINT('Ctrl Pts',(-2.22303912351179,1.87659006314788,-0.391915628763385));
#12489=CARTESIAN_POINT('Ctrl Pts',(-2.22332838298208,1.87629525933482,-0.391966606159889));
#12490=CARTESIAN_POINT('Ctrl Pts',(-2.22361809235949,1.87600087842983,-0.392017663531752));
#12491=CARTESIAN_POINT('Ctrl Pts',(-2.24414409427434,1.85514389729317,-0.395635094634655));
#12492=CARTESIAN_POINT('Ctrl Pts',(-2.26693329697911,1.83641063434651,-0.399654824590917));
#12493=CARTESIAN_POINT('Ctrl Pts',(-2.29128006082217,1.82059521922762,-0.403951952341833));
#12494=CARTESIAN_POINT('Ctrl Pts',(-2.31715625200098,1.80378630335581,-0.408519019239073));
#12495=CARTESIAN_POINT('Ctrl Pts',(-2.34479013883076,1.79027596583773,-0.413399137995121));
#12496=CARTESIAN_POINT('Ctrl Pts',(-2.37328386590736,1.78098419803457,-0.418433352695355));
#12497=CARTESIAN_POINT('Ctrl Pts',(-2.39813004265473,1.77288189170896,-0.422823125500084));
#12498=CARTESIAN_POINT('Ctrl Pts',(-2.42362820852464,1.76798772624127,-0.427329750155805));
#12499=CARTESIAN_POINT('Ctrl Pts',(-2.44917202781645,1.76686823687416,-0.431845791537889));
#12500=CARTESIAN_POINT('Ctrl Pts',(-2.45292199576584,1.76670388990637,-0.432508770329255));
#12501=CARTESIAN_POINT('Ctrl Pts',(-2.4566729502669,1.766620801847,-0.433171952337485));
#12502=CARTESIAN_POINT('Ctrl Pts',(-2.460422980835,1.76662066484191,-0.433834998833824));
#12503=CARTESIAN_POINT('Ctrl Pts',(-2.46095539978625,1.76662064539031,-0.433929136338518));
#12504=CARTESIAN_POINT('Ctrl Pts',(-2.46148780012147,1.76662229797987,-0.434023271112983));
#12505=CARTESIAN_POINT('Ctrl Pts',(-2.46202017631675,1.7666256170716,-0.434117402177783));
#12506=CARTESIAN_POINT('Ctrl Pts',(-2.49337021729807,1.76682106845124,-0.439660498892463));
#12507=CARTESIAN_POINT('Ctrl Pts',(-2.52470190520736,1.77280099958023,-0.445197320624149));
#12508=CARTESIAN_POINT('Ctrl Pts',(-2.55492178827082,1.78347584413678,-0.450535391174815));
#12509=CARTESIAN_POINT('Ctrl Pts',(-2.57526760252786,1.79066278142951,-0.454129296276524));
#12510=CARTESIAN_POINT('Ctrl Pts',(-2.59510952423172,1.79997638628388,-0.457633124067283));
#12511=CARTESIAN_POINT('Ctrl Pts',(-2.61412174689286,1.81107368218895,-0.460989551695197));
#12512=CARTESIAN_POINT('Ctrl Pts',(-2.64023837149477,1.8263177657669,-0.465600194118444));
#12513=CARTESIAN_POINT('Ctrl Pts',(-2.66478693875802,1.8449270679929,-0.46993226175055));
#12514=CARTESIAN_POINT('Ctrl Pts',(-2.6870038349963,1.8660042935492,-0.47385152302486));
#12515=CARTESIAN_POINT('Ctrl Pts',(-2.69130665910911,1.87008639364914,-0.474610580083713));
#12516=CARTESIAN_POINT('Ctrl Pts',(-2.69552217701995,1.87426106856329,-0.475354180395831));
#12517=CARTESIAN_POINT('Ctrl Pts',(-2.6996450775538,1.87852182289951,-0.476081390939429));
#12518=CARTESIAN_POINT('Ctrl Pts',(-2.71349628945441,1.89283616560143,-0.478524512536237));
#12519=CARTESIAN_POINT('Ctrl Pts',(-2.72630673440351,1.90812665369922,-0.48078284574271));
#12520=CARTESIAN_POINT('Ctrl Pts',(-2.73788531809392,1.9241607224898,-0.482822724168243));
#12521=CARTESIAN_POINT('Ctrl Pts',(-2.75564388146651,1.94875285174769,-0.485951371959786));
#12522=CARTESIAN_POINT('Ctrl Pts',(-2.77050254115736,1.97509252268725,-0.488565753139015));
#12523=CARTESIAN_POINT('Ctrl Pts',(-2.78163830746197,2.00236904489192,-0.490520971618943));
#12524=CARTESIAN_POINT('Ctrl Pts',(-2.79136325815834,2.02618984234338,-0.492228479014286));
#12525=CARTESIAN_POINT('Ctrl Pts',(-2.79824948844992,2.05072567441806,-0.49343337360953));
#12526=CARTESIAN_POINT('Ctrl Pts',(-2.80177308229317,2.07545781701756,-0.494043524091528));
#12527=CARTESIAN_POINT('Ctrl Pts',(-2.80372504497939,2.08915866383823,-0.494381528704665));
#12528=CARTESIAN_POINT('Ctrl Pts',(-2.80464571747422,2.10292010438476,-0.494537132455511));
#12529=CARTESIAN_POINT('Ctrl Pts',(-2.80458334954684,2.11665654453875,-0.494518897726551));
#12530=CARTESIAN_POINT('Ctrl Pts',(2.14860532739796,6.34999974434397,2.61193398279736E-6));
#12531=CARTESIAN_POINT('Ctrl Pts',(2.14880376471062,6.340662649241,0.105046613947578));
#12532=CARTESIAN_POINT('Ctrl Pts',(2.14144274304709,6.33132557235638,0.210199967010338));
#12533=CARTESIAN_POINT('Ctrl Pts',(2.12639571524597,6.32198850691087,0.314230311092142));
#12534=CARTESIAN_POINT('Ctrl Pts',(2.11302081122913,6.31368903702332,0.406700125418489));
#12535=CARTESIAN_POINT('Ctrl Pts',(2.09357387058337,6.30538957617378,0.498281788208163));
#12536=CARTESIAN_POINT('Ctrl Pts',(2.06800062383508,6.29709011960108,0.588110040716897));
#12537=CARTESIAN_POINT('Ctrl Pts',(2.04328873085351,6.28907020391933,0.67491271323503));
#12538=CARTESIAN_POINT('Ctrl Pts',(2.01285670810749,6.28105029223114,0.760077599724587));
#12539=CARTESIAN_POINT('Ctrl Pts',(1.97717697406473,6.27303038024048,0.842964335289945));
#12540=CARTESIAN_POINT('Ctrl Pts',(1.93376225290463,6.26327183657012,0.943820034161666));
#12541=CARTESIAN_POINT('Ctrl Pts',(1.88259112117066,6.2535132075724,1.04129200227137));
#12542=CARTESIAN_POINT('Ctrl Pts',(1.82444223822442,6.24375455353849,1.13440813463617));
#12543=CARTESIAN_POINT('Ctrl Pts',(1.76550266292752,6.23386320403898,1.22879043429179));
#12544=CARTESIAN_POINT('Ctrl Pts',(1.69939356847182,6.22397182881777,1.31869878887616));
#12545=CARTESIAN_POINT('Ctrl Pts',(1.62687779287196,6.21408049065924,1.40309928835906));
#12546=CARTESIAN_POINT('Ctrl Pts',(1.58284130110669,6.20807380000796,1.45435298963604));
#12547=CARTESIAN_POINT('Ctrl Pts',(1.53644130771525,6.20206712302445,1.50357504259231));
#12548=CARTESIAN_POINT('Ctrl Pts',(1.48784192275397,6.19606047376889,1.55052731215525));
#12549=CARTESIAN_POINT('Ctrl Pts',(1.41581017995234,6.18715769825804,1.62011777729805));
#12550=CARTESIAN_POINT('Ctrl Pts',(1.33889901588293,6.17825493322457,1.68476045955435));
#12551=CARTESIAN_POINT('Ctrl Pts',(1.2577527291572,6.16935216964046,1.74355725382114));
#12552=CARTESIAN_POINT('Ctrl Pts',(1.22781639563224,6.1660677790577,1.76524845516124));
#12553=CARTESIAN_POINT('Ctrl Pts',(1.19730405087015,6.16278338867221,1.78614435142343));
#12554=CARTESIAN_POINT('Ctrl Pts',(1.16624930383038,6.15949899803066,1.80620114089016));
#12555=CARTESIAN_POINT('Ctrl Pts',(1.08206834466982,6.15059590974889,1.8605696331799));
#12556=CARTESIAN_POINT('Ctrl Pts',(0.993900225083129,6.14169281958567,1.90876882406862));
#12557=CARTESIAN_POINT('Ctrl Pts',(0.902819134132778,6.13278971851196,1.95055782333801));
#12558=CARTESIAN_POINT('Ctrl Pts',(0.856105440240191,6.12822349369061,1.97199057627915));
#12559=CARTESIAN_POINT('Ctrl Pts',(0.808625878921926,6.12365726599931,1.99173792876364));
#12560=CARTESIAN_POINT('Ctrl Pts',(0.760526869968194,6.11909103421993,2.00977246655487));
#12561=CARTESIAN_POINT('Ctrl Pts',(0.653502716799387,6.10893080223198,2.0499007597751));
#12562=CARTESIAN_POINT('Ctrl Pts',(0.543315077176724,6.09877051545036,2.08159140603936));
#12563=CARTESIAN_POINT('Ctrl Pts',(0.431339421902752,6.08861022307749,2.10457030743763));
#12564=CARTESIAN_POINT('Ctrl Pts',(0.320792725181825,6.07857958957245,2.12725596743792));
#12565=CARTESIAN_POINT('Ctrl Pts',(0.208501993543669,6.06854895061798,2.14145099637505));
#12566=CARTESIAN_POINT('Ctrl Pts',(0.0957817413243718,6.05851835355675,
2.14684298427428));
#12567=CARTESIAN_POINT('Ctrl Pts',(0.034359674707909,6.05305260992357,2.14978111680522));
#12568=CARTESIAN_POINT('Ctrl Pts',(-0.0271899640555367,6.04758687872947,
2.15010455086845));
#12569=CARTESIAN_POINT('Ctrl Pts',(-0.0886534609856654,6.04212116763432,
2.14775622505523));
#12570=CARTESIAN_POINT('Ctrl Pts',(-0.16441281023487,6.03538418167625,2.14486169994162));
#12571=CARTESIAN_POINT('Ctrl Pts',(-0.24001500802354,6.02864720091353,2.13790744511307));
#12572=CARTESIAN_POINT('Ctrl Pts',(-0.315006532193144,6.021910216931,2.12679827092486));
#12573=CARTESIAN_POINT('Ctrl Pts',(-0.424539553847577,6.01207014206099,
2.1105721516348));
#12574=CARTESIAN_POINT('Ctrl Pts',(-0.532768639141451,6.00223006032192,
2.08547983748586));
#12575=CARTESIAN_POINT('Ctrl Pts',(-0.63842842684824,5.99238994549198,2.05221400133585));
#12576=CARTESIAN_POINT('Ctrl Pts',(-0.735920068252026,5.98331053158066,
2.0215198173012));
#12577=CARTESIAN_POINT('Ctrl Pts',(-0.831223638478912,5.97423108949699,
1.9838679974274));
#12578=CARTESIAN_POINT('Ctrl Pts',(-0.92336388243848,5.96515159864248,1.93983728460326));
#12579=CARTESIAN_POINT('Ctrl Pts',(-1.05354848936501,5.9523232198886,1.87762645472721));
#12580=CARTESIAN_POINT('Ctrl Pts',(-1.17769422010297,5.93949491342787,1.80256132904901));
#12581=CARTESIAN_POINT('Ctrl Pts',(-1.2932278247383,5.92666663225393,1.71602372051491));
#12582=CARTESIAN_POINT('Ctrl Pts',(-1.40034941353704,5.91477237979598,1.63578692580678));
#12583=CARTESIAN_POINT('Ctrl Pts',(-1.50006803701196,5.90287814907656,1.54568645828586));
#12584=CARTESIAN_POINT('Ctrl Pts',(-1.59029140712846,5.89098390262751,1.44680014240826));
#12585=CARTESIAN_POINT('Ctrl Pts',(-1.59737644411084,5.89004987438338,1.43903482390886));
#12586=CARTESIAN_POINT('Ctrl Pts',(-1.60440290204282,5.88911584604226,1.43121531786644));
#12587=CARTESIAN_POINT('Ctrl Pts',(-1.61136975410245,5.88818181758599,1.42334214208012));
#12588=CARTESIAN_POINT('Ctrl Pts',(-1.62094055997566,5.88689868354518,1.4125262619076));
#12589=CARTESIAN_POINT('Ctrl Pts',(-1.63039714217838,5.88561554994813,1.40161105365249));
#12590=CARTESIAN_POINT('Ctrl Pts',(-1.63973690885178,5.88433241671821,1.39059802595259));
#12591=CARTESIAN_POINT('Ctrl Pts',(-1.75049262821925,5.86911636808519,1.25999992345493));
#12592=CARTESIAN_POINT('Ctrl Pts',(-1.84481868938701,5.85390037108115,1.11564909326681));
#12593=CARTESIAN_POINT('Ctrl Pts',(-1.92110731644144,5.83868429795035,0.962331968016694));
#12594=CARTESIAN_POINT('Ctrl Pts',(-1.96701951219276,5.82952692607041,0.870062305574195));
#12595=CARTESIAN_POINT('Ctrl Pts',(-2.00639931667232,5.8203695266181,0.774544462738395));
#12596=CARTESIAN_POINT('Ctrl Pts',(-2.03890199800151,5.81121207174598,0.676814504551522));
#12597=CARTESIAN_POINT('Ctrl Pts',(-2.07883143620631,5.79996216824644,0.556753569065732));
#12598=CARTESIAN_POINT('Ctrl Pts',(-2.1084572478166,5.78871235944162,0.433114934641564));
#12599=CARTESIAN_POINT('Ctrl Pts',(-2.12702197944784,5.77746258842401,0.307856734199112));
#12600=CARTESIAN_POINT('Ctrl Pts',(-2.14391388897004,5.76722650648383,0.193885240788101));
#12601=CARTESIAN_POINT('Ctrl Pts',(-2.15164844402679,5.75699045582787,0.0785742535437493));
#12602=CARTESIAN_POINT('Ctrl Pts',(-2.14968871231329,5.74675439358754,-0.036584698704585));
#12603=CARTESIAN_POINT('Ctrl Pts',(-2.14889022610864,5.74258374388453,-0.0835058328982378));
#12604=CARTESIAN_POINT('Ctrl Pts',(-2.14648276546956,5.73841309225837,-0.130401630189374));
#12605=CARTESIAN_POINT('Ctrl Pts',(-2.14250453145903,5.73424243580935,-0.17717227139658));
#12606=CARTESIAN_POINT('Ctrl Pts',(-2.13253902319035,5.72379490778094,-0.294333104683244));
#12607=CARTESIAN_POINT('Ctrl Pts',(-2.11273259117636,5.71334734433916,-0.410580783624014));
#12608=CARTESIAN_POINT('Ctrl Pts',(-2.08371969928467,5.70289976543379,-0.524488619165007));
#12609=CARTESIAN_POINT('Ctrl Pts',(-2.05374754544138,5.69210675509167,-0.64216262365711));
#12610=CARTESIAN_POINT('Ctrl Pts',(-2.01394981846877,5.68131372824648,-0.757340867267386));
#12611=CARTESIAN_POINT('Ctrl Pts',(-1.96497129776221,5.67052070689296,-0.868449422790271));
#12612=CARTESIAN_POINT('Ctrl Pts',(-1.94493138059279,5.66610466388447,-0.91391029456369));
#12613=CARTESIAN_POINT('Ctrl Pts',(-1.92335391171395,5.66168862179535,-0.958689730844809));
#12614=CARTESIAN_POINT('Ctrl Pts',(-1.90028070903563,5.65727258213216,-1.00267903367898));
#12615=CARTESIAN_POINT('Ctrl Pts',(-1.85254375919245,5.6481360844016,-1.09369002908814));
#12616=CARTESIAN_POINT('Ctrl Pts',(-1.79834239655419,5.63899961794059,-1.18142666041962));
#12617=CARTESIAN_POINT('Ctrl Pts',(-1.73808607165971,5.6298631690235,-1.26478002970971));
#12618=CARTESIAN_POINT('Ctrl Pts',(-1.69259856836636,5.6229660631855,-1.32770349320893));
#12619=CARTESIAN_POINT('Ctrl Pts',(-1.64366163074749,5.61606896734535,-1.38812906495699));
#12620=CARTESIAN_POINT('Ctrl Pts',(-1.59146897410807,5.60917187559826,-1.44558863599498));
#12621=CARTESIAN_POINT('Ctrl Pts',(-1.52248449585653,5.60005579861998,-1.52153454072249));
#12622=CARTESIAN_POINT('Ctrl Pts',(-1.44781169944092,5.59093972879212,-1.59229708604899));
#12623=CARTESIAN_POINT('Ctrl Pts',(-1.36849398618179,5.58182365248058,-1.65734003225809));
#12624=CARTESIAN_POINT('Ctrl Pts',(-1.36408398969738,5.58131680649582,-1.66095636399952));
#12625=CARTESIAN_POINT('Ctrl Pts',(-1.35965964204295,5.58080996049102,-1.66455502598097));
#12626=CARTESIAN_POINT('Ctrl Pts',(-1.355221125012,5.58030311446383,-1.66813593002742));
#12627=CARTESIAN_POINT('Ctrl Pts',(-1.269060793176,5.57046423774273,-1.73764830967226));
#12628=CARTESIAN_POINT('Ctrl Pts',(-1.17755335950336,5.56062527924614,-1.80048101079417));
#12629=CARTESIAN_POINT('Ctrl Pts',(-1.08184958870044,5.55078630172061,-1.85609286767396));
#12630=CARTESIAN_POINT('Ctrl Pts',(-0.985603365185632,5.54089155648608,
-1.9120199347312));
#12631=CARTESIAN_POINT('Ctrl Pts',(-0.885111900569775,5.53099679200629,
-1.96064473276489));
#12632=CARTESIAN_POINT('Ctrl Pts',(-0.781515883586216,5.5211020721009,-2.00137462967412));
#12633=CARTESIAN_POINT('Ctrl Pts',(-0.719503403348289,5.51517910188969,
-2.02575550840595));
#12634=CARTESIAN_POINT('Ctrl Pts',(-0.656378011428396,5.50925614765042,
-2.04730662538622));
#12635=CARTESIAN_POINT('Ctrl Pts',(-0.592382047293052,5.50333322307176,
-2.06589217974674));
#12636=CARTESIAN_POINT('Ctrl Pts',(-0.495077335604388,5.49432752284883,
-2.09415118065497));
#12637=CARTESIAN_POINT('Ctrl Pts',(-0.395728162407976,5.48532182713199,
-2.11555758228668));
#12638=CARTESIAN_POINT('Ctrl Pts',(-0.295343829160877,5.47631612587051,
-2.12958822780567));
#12639=CARTESIAN_POINT('Ctrl Pts',(-0.277744101562778,5.47473721525861,
-2.13204812897922));
#12640=CARTESIAN_POINT('Ctrl Pts',(-0.260112597674987,5.47315830447628,
-2.13428143399914));
#12641=CARTESIAN_POINT('Ctrl Pts',(-0.242454802330516,5.47157939346935,
-2.13628548398197));
#12642=CARTESIAN_POINT('Ctrl Pts',(-0.141589680320261,5.46256031445918,
-2.14773304819311));
#12643=CARTESIAN_POINT('Ctrl Pts',(-0.0398667183094937,5.45354122812046,
-2.15169583131827));
#12644=CARTESIAN_POINT('Ctrl Pts',(0.0616071250593509,5.44452212435753,
-2.14844214333508));
#12645=CARTESIAN_POINT('Ctrl Pts',(0.129706859397744,5.43846934711135,-2.14625857287082));
#12646=CARTESIAN_POINT('Ctrl Pts',(0.197694264497796,5.43241656201761,-2.14082596253566));
#12647=CARTESIAN_POINT('Ctrl Pts',(0.265237158184707,5.42636376602485,-2.13223832829264));
#12648=CARTESIAN_POINT('Ctrl Pts',(0.382371048324121,5.41586691724992,-2.11734552534815));
#12649=CARTESIAN_POINT('Ctrl Pts',(0.49831454004301,5.40537003965045,-2.09295237197418));
#12650=CARTESIAN_POINT('Ctrl Pts',(0.611562267195913,5.39487316597188,-2.0594489299804));
#12651=CARTESIAN_POINT('Ctrl Pts',(0.722308338854742,5.38460816945648,-2.02668558292576));
#12652=CARTESIAN_POINT('Ctrl Pts',(0.830477706126031,5.37434317669068,-1.98520949062172));
#12653=CARTESIAN_POINT('Ctrl Pts',(0.93464491267495,5.36407821829738,-1.9353401923379));
#12654=CARTESIAN_POINT('Ctrl Pts',(0.984316346245632,5.35918344175655,-1.91156035203127));
#12655=CARTESIAN_POINT('Ctrl Pts',(1.03307739142291,5.35428867303132,-1.88587144447327));
#12656=CARTESIAN_POINT('Ctrl Pts',(1.08077076705523,5.34939391544197,-1.85830486182312));
#12657=CARTESIAN_POINT('Ctrl Pts',(1.13078671291648,5.34426079312997,-1.82939584275852));
#12658=CARTESIAN_POINT('Ctrl Pts',(1.17960617224486,5.33912767551624,-1.79843411893778));
#12659=CARTESIAN_POINT('Ctrl Pts',(1.2270341705754,5.3339945580915,-1.76547079971493));
#12660=CARTESIAN_POINT('Ctrl Pts',(1.32471108062967,5.3234230166678,-1.69758357528728));
#12661=CARTESIAN_POINT('Ctrl Pts',(1.41648363708775,5.31285147604563,-1.62120442851145));
#12662=CARTESIAN_POINT('Ctrl Pts',(1.50135016528333,5.30227989683554,-1.53778457154753));
#12663=CARTESIAN_POINT('Ctrl Pts',(1.58124141099987,5.29232807424726,-1.45925518626405));
#12664=CARTESIAN_POINT('Ctrl Pts',(1.65501230994021,5.28237621746289,-1.37448765350144));
#12665=CARTESIAN_POINT('Ctrl Pts',(1.72186324495689,5.27242429362231,-1.28471467058922));
#12666=CARTESIAN_POINT('Ctrl Pts',(1.81836964190101,5.25805763873146,-1.15511787255459));
#12667=CARTESIAN_POINT('Ctrl Pts',(1.90070202076568,5.24369111383716,-1.01477291661791));
#12668=CARTESIAN_POINT('Ctrl Pts',(1.96642481069052,5.22932461427314,-0.867071437992345));
#12669=CARTESIAN_POINT('Ctrl Pts',(2.01660616146925,5.21835535452459,-0.754296862872764));
#12670=CARTESIAN_POINT('Ctrl Pts',(2.05710374954887,5.20738610954305,-0.637233730207292));
#12671=CARTESIAN_POINT('Ctrl Pts',(2.08681487532426,5.19641683273928,-0.517400885311197));
#12672=CARTESIAN_POINT('Ctrl Pts',(2.08768368483754,5.19609607033825,-0.513896746274617));
#12673=CARTESIAN_POINT('Ctrl Pts',(2.08854326971608,5.19577530791001,-0.510390239614455));
#12674=CARTESIAN_POINT('Ctrl Pts',(2.08939363433078,5.19545454545339,-0.506881411421222));
#12675=CARTESIAN_POINT('Ctrl Pts',(2.12478138995841,5.18210607912133,-0.360862218600595));
#12676=CARTESIAN_POINT('Ctrl Pts',(2.14413645684879,5.16875764625848,-0.211109615031524));
#12677=CARTESIAN_POINT('Ctrl Pts',(2.14794363642467,5.15540918199055,-0.06094667525413));
#12678=CARTESIAN_POINT('Ctrl Pts',(2.15145408794799,5.14310108467356,0.0775127039739754));
#12679=CARTESIAN_POINT('Ctrl Pts',(2.14174521530511,5.13079296065605,0.216322310287955));
#12680=CARTESIAN_POINT('Ctrl Pts',(2.11916587699683,5.11848475908094,0.35290065136281));
#12681=CARTESIAN_POINT('Ctrl Pts',(2.10039841736405,5.10825444705588,0.46642162650563));
#12682=CARTESIAN_POINT('Ctrl Pts',(2.07270108649064,5.09802420591568,0.578596776354617));
#12683=CARTESIAN_POINT('Ctrl Pts',(2.03621821645373,5.0877939988326,0.687825029565731));
#12684=CARTESIAN_POINT('Ctrl Pts',(2.00179883488851,5.07814241712515,0.790875280852756));
#12685=CARTESIAN_POINT('Ctrl Pts',(1.95956019064648,5.06849086573123,0.891301421975115));
#12686=CARTESIAN_POINT('Ctrl Pts',(1.90966579129595,5.05883931372533,0.987763415838006));
#12687=CARTESIAN_POINT('Ctrl Pts',(1.87981301268525,5.05306460455893,1.04547848174961));
#12688=CARTESIAN_POINT('Ctrl Pts',(1.84722039009149,5.04728989517344,1.1017746186486));
#12689=CARTESIAN_POINT('Ctrl Pts',(1.81210119078509,5.04151517894493,1.15645675235276));
#12690=CARTESIAN_POINT('Ctrl Pts',(1.75066236072355,5.03141267615376,1.25211970556366));
#12691=CARTESIAN_POINT('Ctrl Pts',(1.68154128808941,5.02131011601506,1.34277513267819));
#12692=CARTESIAN_POINT('Ctrl Pts',(1.60581470583693,5.01120753771401,1.42753203538759));
#12693=CARTESIAN_POINT('Ctrl Pts',(1.52826415897905,5.0008616268249,1.51433040868771));
#12694=CARTESIAN_POINT('Ctrl Pts',(1.443785182022,4.99051569688795,1.59494374835389));
#12695=CARTESIAN_POINT('Ctrl Pts',(1.35348823723746,4.98016978998863,1.66838712784109));
#12696=CARTESIAN_POINT('Ctrl Pts',(1.30803241324631,4.97496162127189,1.70535880323111));
#12697=CARTESIAN_POINT('Ctrl Pts',(1.26110159502111,4.96975345839323,1.74051296377186));
#12698=CARTESIAN_POINT('Ctrl Pts',(1.21283431888366,4.96454530672151,1.7737200509744));
#12699=CARTESIAN_POINT('Ctrl Pts',(1.12974779416806,4.9555800769173,1.83088220497145));
#12700=CARTESIAN_POINT('Ctrl Pts',(1.04261723061714,4.94661486682201,1.88232639240326));
#12701=CARTESIAN_POINT('Ctrl Pts',(0.952263314461416,4.93764966669292,1.92728410921836));
#12702=CARTESIAN_POINT('Ctrl Pts',(0.897179510252508,4.93218407815381,1.95469235200503));
#12703=CARTESIAN_POINT('Ctrl Pts',(0.840898457955948,4.92671849331882,1.97969045585849));
#12704=CARTESIAN_POINT('Ctrl Pts',(0.783611574738666,4.92125290998036,2.00211210972785));
#12705=CARTESIAN_POINT('Ctrl Pts',(0.689741169800707,4.91229699385456,2.0388522779809));
#12706=CARTESIAN_POINT('Ctrl Pts',(0.593169828820591,4.90334108174698,2.06867185494086));
#12707=CARTESIAN_POINT('Ctrl Pts',(0.495016264703413,4.89438516394511,2.09155192935259));
#12708=CARTESIAN_POINT('Ctrl Pts',(0.470140463553974,4.89211539786627,2.0973505998998));
#12709=CARTESIAN_POINT('Ctrl Pts',(0.445163078199004,4.88984563142169,2.10270380045615));
#12710=CARTESIAN_POINT('Ctrl Pts',(0.420102366121439,4.88757586445325,2.10761174972201));
#12711=CARTESIAN_POINT('Ctrl Pts',(0.310810276068341,4.87767720015569,2.12901577174183));
#12712=CARTESIAN_POINT('Ctrl Pts',(0.199882936393077,4.86777845891062,2.14196622068233));
#12713=CARTESIAN_POINT('Ctrl Pts',(0.0886129714964294,4.85787970263818,
2.14648118705205));
#12714=CARTESIAN_POINT('Ctrl Pts',(-0.022450796580891,4.84799928996872,
2.15098778663828));
#12715=CARTESIAN_POINT('Ctrl Pts',(-0.13385729235645,4.83811886232756,2.14709013848741));
#12716=CARTESIAN_POINT('Ctrl Pts',(-0.24432546663264,4.82823848129131,2.13475568838697));
#12717=CARTESIAN_POINT('Ctrl Pts',(-0.310039445163978,4.82236095908592,
2.12741831910024));
#12718=CARTESIAN_POINT('Ctrl Pts',(-0.375421367891689,4.81648345337251,
2.11709447375088));
#12719=CARTESIAN_POINT('Ctrl Pts',(-0.440199281626035,4.81060597711322,
2.10376877792093));
#12720=CARTESIAN_POINT('Ctrl Pts',(-0.539190248072235,4.80162425754816,
2.08340499290951));
#12721=CARTESIAN_POINT('Ctrl Pts',(-0.636768480871051,4.79264254195598,
2.05602620706925));
#12722=CARTESIAN_POINT('Ctrl Pts',(-0.731816032994038,4.7836608170803,2.02161947317196));
#12723=CARTESIAN_POINT('Ctrl Pts',(-0.829615042770138,4.77441908723767,
1.98621672549856));
#12724=CARTESIAN_POINT('Ctrl Pts',(-0.924733513944005,4.76517734756626,
1.94337333383143));
#12725=CARTESIAN_POINT('Ctrl Pts',(-1.01624004259855,4.75593558362472,1.89387054506982));
#12726=CARTESIAN_POINT('Ctrl Pts',(-1.08983740092588,4.74850256849036,1.85405617842014));
#12727=CARTESIAN_POINT('Ctrl Pts',(-1.16109841751715,4.7410695376563,1.80993521110809));
#12728=CARTESIAN_POINT('Ctrl Pts',(-1.22955343864502,4.73363648360911,1.76193346081459));
#12729=CARTESIAN_POINT('Ctrl Pts',(-1.3313510344479,4.72258299156411,1.69055136650364));
#12730=CARTESIAN_POINT('Ctrl Pts',(-1.4271061270336,4.71152950431796,1.61048339724775));
#12731=CARTESIAN_POINT('Ctrl Pts',(-1.51542254683858,4.70047603071412,1.52291719146958));
#12732=CARTESIAN_POINT('Ctrl Pts',(-1.6008248474513,4.68978728135569,1.43824035056166));
#12733=CARTESIAN_POINT('Ctrl Pts',(-1.67927212165502,4.67909854475413,1.34655087460194));
#12734=CARTESIAN_POINT('Ctrl Pts',(-1.74946300834417,4.66840982890598,1.24889502111413));
#12735=CARTESIAN_POINT('Ctrl Pts',(-1.77516813001075,4.66449543553818,1.21313175163907));
#12736=CARTESIAN_POINT('Ctrl Pts',(-1.79976549737413,4.66058104495373,1.17656810305738));
#12737=CARTESIAN_POINT('Ctrl Pts',(-1.82318948990156,4.65666665754538,1.13925490583306));
#12738=CARTESIAN_POINT('Ctrl Pts',(-1.84430714638878,4.65313768234824,1.10561558151633));
#12739=CARTESIAN_POINT('Ctrl Pts',(-1.86446248188883,4.64960871019584,1.0713806031278));
#12740=CARTESIAN_POINT('Ctrl Pts',(-1.88360724270868,4.6460797394394,1.03659237669773));
#12741=CARTESIAN_POINT('Ctrl Pts',(-1.94789431407824,4.63422964650719,0.919775393901501));
#12742=CARTESIAN_POINT('Ctrl Pts',(-2.00078253174395,4.62237956931563,0.796719402573613));
#12743=CARTESIAN_POINT('Ctrl Pts',(-2.04194024364151,4.61052944543686,0.669845135897601));
#12744=CARTESIAN_POINT('Ctrl Pts',(-2.07763572815337,4.60025200546567,0.5598089309609));
#12745=CARTESIAN_POINT('Ctrl Pts',(-2.10450838578849,4.58997453037713,0.446901634662001));
#12746=CARTESIAN_POINT('Ctrl Pts',(-2.12237362560969,4.57969697944582,0.332700398221384));
#12747=CARTESIAN_POINT('Ctrl Pts',(-2.14719082634332,4.56542009052269,0.174059650202283));
#12748=CARTESIAN_POINT('Ctrl Pts',(-2.15469089740905,4.55114335207784,0.0125183563644346));
#12749=CARTESIAN_POINT('Ctrl Pts',(-2.14418756886859,4.5368666433287,-0.147802409798827));
#12750=CARTESIAN_POINT('Ctrl Pts',(-2.13723154232329,4.52741162488803,-0.253977847508746));
#12751=CARTESIAN_POINT('Ctrl Pts',(-2.12237988566817,4.51795661947189,-0.359616808663046));
#12752=CARTESIAN_POINT('Ctrl Pts',(-2.09944170626511,4.50850159199649,-0.463513238179406));
#12753=CARTESIAN_POINT('Ctrl Pts',(-2.09477215260164,4.50657682031299,-0.484663563344447));
#12754=CARTESIAN_POINT('Ctrl Pts',(-2.08976750615382,4.50465204771533,-0.50574165910436));
#12755=CARTESIAN_POINT('Ctrl Pts',(-2.08443318488955,4.50272727390753,-0.52673887188011));
#12756=CARTESIAN_POINT('Ctrl Pts',(-2.0528249925357,4.49132214516846,-0.651156563922029));
#12757=CARTESIAN_POINT('Ctrl Pts',(-2.00969503857243,4.47991701802016,-0.772541532210201));
#12758=CARTESIAN_POINT('Ctrl Pts',(-1.95623195885362,4.46851187550785,-0.889203652466676));
#12759=CARTESIAN_POINT('Ctrl Pts',(-1.90007420389999,4.45653188479675,-1.0117458403876));
#12760=CARTESIAN_POINT('Ctrl Pts',(-1.832515037961,4.4445518771338,-1.12907841821667));
#12761=CARTESIAN_POINT('Ctrl Pts',(-1.75487604325656,4.43257183286906,-1.23923821120557));
#12762=CARTESIAN_POINT('Ctrl Pts',(-1.74015542163619,4.43030037508824,-1.26012488853235));
#12763=CARTESIAN_POINT('Ctrl Pts',(-1.72507229226648,4.42802891599161,-1.28075366099619));
#12764=CARTESIAN_POINT('Ctrl Pts',(-1.70963547178022,4.42575745544522,-1.30111106658976));
#12765=CARTESIAN_POINT('Ctrl Pts',(-1.64425450402648,4.41613693230257,-1.38733263532844));
#12766=CARTESIAN_POINT('Ctrl Pts',(-1.57242672947706,4.40651646136546,-1.46881371158882));
#12767=CARTESIAN_POINT('Ctrl Pts',(-1.49486263555717,4.39689601833018,-1.54439705008315));
#12768=CARTESIAN_POINT('Ctrl Pts',(-1.42506126093028,4.38823840222916,-1.61241590596306));
#12769=CARTESIAN_POINT('Ctrl Pts',(-1.35061536726574,4.37958080872456,-1.67565804297037));
#12770=CARTESIAN_POINT('Ctrl Pts',(-1.27207216031375,4.37092322010378,-1.73330101803169));
#12771=CARTESIAN_POINT('Ctrl Pts',(-1.20513370597715,4.36354478951702,-1.78242724808653));
#12772=CARTESIAN_POINT('Ctrl Pts',(-1.13521995499769,4.35616636247752,-1.82748687396669));
#12773=CARTESIAN_POINT('Ctrl Pts',(-1.06291994134801,4.34878792802094,-1.86831238411785));
#12774=CARTESIAN_POINT('Ctrl Pts',(-0.965762182306972,4.33887268567387,
-1.92317426972154));
#12775=CARTESIAN_POINT('Ctrl Pts',(-0.864335597444932,4.32895737015848,
-1.97037545764872));
#12776=CARTESIAN_POINT('Ctrl Pts',(-0.759915575653579,4.31904203459314,
-2.0096134761703));
#12777=CARTESIAN_POINT('Ctrl Pts',(-0.653808176651047,4.30896647198526,
-2.04948556215451));
#12778=CARTESIAN_POINT('Ctrl Pts',(-0.544608532407727,4.29889088867419,
-2.08113553109579));
#12779=CARTESIAN_POINT('Ctrl Pts',(-0.433629444273735,4.28881534039535,
-2.10419960703838));
#12780=CARTESIAN_POINT('Ctrl Pts',(-0.371222605833282,4.28314956025416,
-2.11716922217335));
#12781=CARTESIAN_POINT('Ctrl Pts',(-0.308252733748727,4.27748379119067,
-2.12742297787052));
#12782=CARTESIAN_POINT('Ctrl Pts',(-0.244952189086059,4.27181804311557,
-2.13488900026679));
#12783=CARTESIAN_POINT('Ctrl Pts',(-0.145431729722479,4.262910412793,-2.14662700319324));
#12784=CARTESIAN_POINT('Ctrl Pts',(-0.0450219341622343,4.25400279354217,
-2.15147742757369));
#12785=CARTESIAN_POINT('Ctrl Pts',(0.0552171185010954,4.2450951771393,-2.14912756247981));
#12786=CARTESIAN_POINT('Ctrl Pts',(0.0993365333513108,4.24117456124197,
-2.1480932882108));
#12787=CARTESIAN_POINT('Ctrl Pts',(0.143422701192644,4.23725394589637,-2.1456647903115));
#12788=CARTESIAN_POINT('Ctrl Pts',(0.187384846907493,4.23333333040127,-2.14181860089706));
#12789=CARTESIAN_POINT('Ctrl Pts',(0.287266585265252,4.22442571488989,-2.13308008100634));
#12790=CARTESIAN_POINT('Ctrl Pts',(0.386507179702926,4.21551809860677,-2.11702004911881));
#12791=CARTESIAN_POINT('Ctrl Pts',(0.484109414113608,4.20661047332809,-2.09410887618576));
#12792=CARTESIAN_POINT('Ctrl Pts',(0.527068254042148,4.20268985357178,-2.08402470734937));
#12793=CARTESIAN_POINT('Ctrl Pts',(0.569709868528226,4.19876923207281,-2.07261397057064));
#12794=CARTESIAN_POINT('Ctrl Pts',(0.611950397910045,4.19484860812996,-2.05991973801053));
#12795=CARTESIAN_POINT('Ctrl Pts',(0.72031208345076,4.18479084074316,-2.02735460549466));
#12796=CARTESIAN_POINT('Ctrl Pts',(0.826122770602239,4.17473301047741,-1.986321847705));
#12797=CARTESIAN_POINT('Ctrl Pts',(0.928169509366776,4.16467517176985,-1.93743193176917));
#12798=CARTESIAN_POINT('Ctrl Pts',(1.02922438286487,4.15471509239287,-1.88901721190607));
#12799=CARTESIAN_POINT('Ctrl Pts',(1.12658932179402,4.14475500473742,-1.83289666383873));
#12800=CARTESIAN_POINT('Ctrl Pts',(1.21906484916275,4.13479496166867,-1.7696182042326));
#12801=CARTESIAN_POINT('Ctrl Pts',(1.27141877703239,4.1291562008934,-1.73379385151805));
#12802=CARTESIAN_POINT('Ctrl Pts',(1.32220509692019,4.12351745440871,-1.69567453684527));
#12803=CARTESIAN_POINT('Ctrl Pts',(1.37120083966543,4.11787873180722,-1.65535441079667));
#12804=CARTESIAN_POINT('Ctrl Pts',(1.43531317852335,4.11050030107228,-1.60259436596047));
#12805=CARTESIAN_POINT('Ctrl Pts',(1.49634026065668,4.10312187494314,-1.54607890137562));
#12806=CARTESIAN_POINT('Ctrl Pts',(1.55373108906351,4.09574344359535,-1.48607526842546));
#12807=CARTESIAN_POINT('Ctrl Pts',(1.62856052425888,4.08612302399678,-1.40783910965279));
#12808=CARTESIAN_POINT('Ctrl Pts',(1.69720621922258,4.07650259552624,-1.32367226301154));
#12809=CARTESIAN_POINT('Ctrl Pts',(1.75912692331253,4.06688213640668,-1.23481791804035));
#12810=CARTESIAN_POINT('Ctrl Pts',(1.81485044483566,4.05822451746178,-1.15485634335877));
#12811=CARTESIAN_POINT('Ctrl Pts',(1.86512796421619,4.04956687369575,-1.07109975029203));
#12812=CARTESIAN_POINT('Ctrl Pts',(1.90959783197144,4.04090918923747,-0.9844691833771));
#12813=CARTESIAN_POINT('Ctrl Pts',(1.97123887704193,4.02890850776849,-0.864387902517969));
#12814=CARTESIAN_POINT('Ctrl Pts',(2.02184616441858,4.01690787343384,-0.738562419696407));
#12815=CARTESIAN_POINT('Ctrl Pts',(2.06046390294875,4.00490726149064,-0.609168226113287));
#12816=CARTESIAN_POINT('Ctrl Pts',(2.09724139047428,3.99347851468055,-0.485940053737005));
#12817=CARTESIAN_POINT('Ctrl Pts',(2.12314494697457,3.98204978817869,-0.359473900304984));
#12818=CARTESIAN_POINT('Ctrl Pts',(2.13730195886065,3.97062106061345,-0.231649889169576));
#12819=CARTESIAN_POINT('Ctrl Pts',(2.14006086779408,3.96839383788938,-0.20673963204283));
#12820=CARTESIAN_POINT('Ctrl Pts',(2.14237351304075,3.96616661512494,-0.181777842159215));
#12821=CARTESIAN_POINT('Ctrl Pts',(2.14423320644537,3.96393939216193,-0.156778500878331));
#12822=CARTESIAN_POINT('Ctrl Pts',(2.14584035961558,3.96201461873592,-0.135173987740378));
#12823=CARTESIAN_POINT('Ctrl Pts',(2.14710880128732,3.96008984632443,-0.11354706786211));
#12824=CARTESIAN_POINT('Ctrl Pts',(2.14803469848385,3.95816507465925,-0.0919072041729757));
#12825=CARTESIAN_POINT('Ctrl Pts',(2.15490242896436,3.94388831360785,0.0686038676925654));
#12826=CARTESIAN_POINT('Ctrl Pts',(2.14292173815727,3.92961159361594,0.229824217247526));
#12827=CARTESIAN_POINT('Ctrl Pts',(2.11346589439703,3.91533480522002,0.38778518067942));
#12828=CARTESIAN_POINT('Ctrl Pts',(2.09395834183425,3.90587979852159,0.492397081193876));
#12829=CARTESIAN_POINT('Ctrl Pts',(2.06678697144009,3.89642476182156,0.595580002711112));
#12830=CARTESIAN_POINT('Ctrl Pts',(2.03235718415981,3.88696966332459,0.696192242023687));
#12831=CARTESIAN_POINT('Ctrl Pts',(1.98920577051361,3.87511943424862,0.822291201657256));
#12832=CARTESIAN_POINT('Ctrl Pts',(1.93455889875707,3.86326931194115,0.944616676195892));
#12833=CARTESIAN_POINT('Ctrl Pts',(1.86911866174675,3.85141922753818,1.06083676473496));
#12834=CARTESIAN_POINT('Ctrl Pts',(1.81236306818258,3.84114178043831,1.16163316172961));
#12835=CARTESIAN_POINT('Ctrl Pts',(1.74748992338059,3.83086436184984,1.25783628961372));
#12836=CARTESIAN_POINT('Ctrl Pts',(1.674988639014,3.82058692684825,1.34792917439058));
#12837=CARTESIAN_POINT('Ctrl Pts',(1.65009381796463,3.81705795619006,1.37886443662677));
#12838=CARTESIAN_POINT('Ctrl Pts',(1.62429984567893,3.81352898359671,1.40907937140894));
#12839=CARTESIAN_POINT('Ctrl Pts',(1.59766160651677,3.81000000724943,1.43854059611177));
#12840=CARTESIAN_POINT('Ctrl Pts',(1.51729984919832,3.79935385533692,1.5274186850673));
#12841=CARTESIAN_POINT('Ctrl Pts',(1.42935673322849,3.788707678032,1.60933109459253));
#12842=CARTESIAN_POINT('Ctrl Pts',(1.33529447087369,3.77806148606583,1.68349262622453));
#12843=CARTESIAN_POINT('Ctrl Pts',(1.23773059337837,3.76701897291787,1.76041493710537));
#12844=CARTESIAN_POINT('Ctrl Pts',(1.13358247687332,3.75597644399672,1.82899949817504));
#12845=CARTESIAN_POINT('Ctrl Pts',(1.0244378094136,3.74493391127711,1.88833689452043));
#12846=CARTESIAN_POINT('Ctrl Pts',(0.985218829988154,3.74096599535768,1.90965861532084));
#12847=CARTESIAN_POINT('Ctrl Pts',(0.945354382089341,3.73699807894779,1.92978598521962));
#12848=CARTESIAN_POINT('Ctrl Pts',(0.904917226262744,3.73303016260304,1.94867544599454));
#12849=CARTESIAN_POINT('Ctrl Pts',(0.810733708389469,3.72378835732925,1.99267151421802));
#12850=CARTESIAN_POINT('Ctrl Pts',(0.7133192154603,3.71454658877054,2.03000494321816));
#12851=CARTESIAN_POINT('Ctrl Pts',(0.613707760854252,3.70530484082039,2.06003066325302));
#12852=CARTESIAN_POINT('Ctrl Pts',(0.533591656612385,3.69787183178464,2.08417993128412));
#12853=CARTESIAN_POINT('Ctrl Pts',(0.452055362080121,3.69043883608009,2.10360258824914));
#12854=CARTESIAN_POINT('Ctrl Pts',(0.36964756560502,3.68300584532693,2.11798505125678));
#12855=CARTESIAN_POINT('Ctrl Pts',(0.270069332753102,3.67402412131944,2.13536423516435));
#12856=CARTESIAN_POINT('Ctrl Pts',(0.169219256536759,3.66504240454161,2.14538279323063));
#12857=CARTESIAN_POINT('Ctrl Pts',(0.0681960517151269,3.65606068020844,
2.1482476056522));
#12858=CARTESIAN_POINT('Ctrl Pts',(-0.0424951484675184,3.64621939821879,
2.15138658273971));
#12859=CARTESIAN_POINT('Ctrl Pts',(-0.153392117145235,3.63637803514527,
2.14594608438397));
#12860=CARTESIAN_POINT('Ctrl Pts',(-0.263251987505055,3.62653665222612,
2.13220831198733));
#12861=CARTESIAN_POINT('Ctrl Pts',(-0.374061522960836,3.61661019713436,
2.11835178573727));
#12862=CARTESIAN_POINT('Ctrl Pts',(-0.483817310267165,3.6066837218524,2.09605372877359));
#12863=CARTESIAN_POINT('Ctrl Pts',(-0.591242871291941,3.59675728922043,
2.06555172845434));
#12864=CARTESIAN_POINT('Ctrl Pts',(-0.654973047937661,3.59086843652037,
2.04745642739331));
#12865=CARTESIAN_POINT('Ctrl Pts',(-0.717882993580609,3.58497959883076,
2.0264728153448));
#12866=CARTESIAN_POINT('Ctrl Pts',(-0.779703005872109,3.57909078927208,
2.00264238198665));
#12867=CARTESIAN_POINT('Ctrl Pts',(-0.873721151897173,3.57013487133419,
1.96640018338044));
#12868=CARTESIAN_POINT('Ctrl Pts',(-0.965256992030045,3.5611789590792,1.92355258044361));
#12869=CARTESIAN_POINT('Ctrl Pts',(-1.05320797236887,3.55222304345234,1.87429990683767));
#12870=CARTESIAN_POINT('Ctrl Pts',(-1.07549803889703,3.54995327960918,1.86181743799949));
#12871=CARTESIAN_POINT('Ctrl Pts',(-1.09755792374472,3.54768351554944,1.84892381735926));
#12872=CARTESIAN_POINT('Ctrl Pts',(-1.11936987351294,3.54541375112573,1.83562280614203));
#12873=CARTESIAN_POINT('Ctrl Pts',(-1.20552346155375,3.53644855767956,1.78308601538688));
#12874=CARTESIAN_POINT('Ctrl Pts',(-1.28780634668958,3.52748335855489,1.72419020306907));
#12875=CARTESIAN_POINT('Ctrl Pts',(-1.36552068167549,3.51851814466872,1.65981285611839));
#12876=CARTESIAN_POINT('Ctrl Pts',(-1.41289880986703,3.51305255002855,1.62056555126769));
#12877=CARTESIAN_POINT('Ctrl Pts',(-1.45857956462854,3.50758694990203,1.57928181390491));
#12878=CARTESIAN_POINT('Ctrl Pts',(-1.50241189349563,3.50212134223111,1.5361667894027));
#12879=CARTESIAN_POINT('Ctrl Pts',(-1.58533092929737,3.49178187522451,1.4546047014942));
#12880=CARTESIAN_POINT('Ctrl Pts',(-1.66173246807074,3.4814423680699,1.36640237637631));
#12881=CARTESIAN_POINT('Ctrl Pts',(-1.73071604045821,3.47110286104971,1.27273692558878));
#12882=CARTESIAN_POINT('Ctrl Pts',(-1.79843625189437,3.46095271113256,1.18078685817321));
#12883=CARTESIAN_POINT('Ctrl Pts',(-1.8590084362504,3.45080256134496,1.08357076733883));
#12884=CARTESIAN_POINT('Ctrl Pts',(-1.91153970529294,3.44065244979636,0.982175567345101));
#12885=CARTESIAN_POINT('Ctrl Pts',(-1.938281193755,3.43548544934477,0.930559480009675));
#12886=CARTESIAN_POINT('Ctrl Pts',(-1.9629382272084,3.43031845880245,0.877860092613464));
#12887=CARTESIAN_POINT('Ctrl Pts',(-1.98538790967749,3.42515148319672,0.824219506712342));
#12888=CARTESIAN_POINT('Ctrl Pts',(-2.01047811662508,3.41937676957128,0.764269732237709));
#12889=CARTESIAN_POINT('Ctrl Pts',(-2.03279986241567,3.41360206091566,0.703169210488066));
#12890=CARTESIAN_POINT('Ctrl Pts',(-2.05217699413633,3.40782735126269,0.641147085472373));
#12891=CARTESIAN_POINT('Ctrl Pts',(-2.08650455004101,3.39759716491195,0.531271795646451));
#12892=CARTESIAN_POINT('Ctrl Pts',(-2.11158768355524,3.38736697543116,0.418503998794418));
#12893=CARTESIAN_POINT('Ctrl Pts',(-2.12751323101412,3.37713674964412,0.304449183630048));
#12894=CARTESIAN_POINT('Ctrl Pts',(-2.14253799199325,3.36748516952673,0.196845577487949));
#12895=CARTESIAN_POINT('Ctrl Pts',(-2.14941231931092,3.3578335570941,0.0880975860949286));
#12896=CARTESIAN_POINT('Ctrl Pts',(-2.14825154044069,3.34818188448715,-0.0204499931582646));
#12897=CARTESIAN_POINT('Ctrl Pts',(-2.14664614148736,3.33483327391323,-0.170575201834474));
#12898=CARTESIAN_POINT('Ctrl Pts',(-2.12967714969834,3.32148476313739,-0.3206566064012));
#12899=CARTESIAN_POINT('Ctrl Pts',(-2.09747674712209,3.30813627916616,-0.46737274837291));
#12900=CARTESIAN_POINT('Ctrl Pts',(-2.06778615671754,3.29582822279411,-0.602653320306828));
#12901=CARTESIAN_POINT('Ctrl Pts',(-2.0251455732522,3.283520189211,-0.735073410914382));
#12902=CARTESIAN_POINT('Ctrl Pts',(-1.96963201681683,3.27121212119573,-0.862000140862884));
#12903=CARTESIAN_POINT('Ctrl Pts',(-1.96818526952361,3.27089135875086,-0.865307997804165));
#12904=CARTESIAN_POINT('Ctrl Pts',(-1.96672984517333,3.27057059632982,-0.868611967399311));
#12905=CARTESIAN_POINT('Ctrl Pts',(-1.965265747465,3.27024983393156,-0.871912003499029));
#12906=CARTESIAN_POINT('Ctrl Pts',(-1.8996909223591,3.25588334865774,-1.01971586170543));
#12907=CARTESIAN_POINT('Ctrl Pts',(-1.81672182290529,3.24151690909339,-1.15962744970581));
#12908=CARTESIAN_POINT('Ctrl Pts',(-1.71938423090768,3.22715042128175,-1.28871874275917));
#12909=CARTESIAN_POINT('Ctrl Pts',(-1.64506358019347,3.21618110613098,-1.38728445313241));
#12910=CARTESIAN_POINT('Ctrl Pts',(-1.56236501271207,3.20521176285271,-1.47954265375796));
#12911=CARTESIAN_POINT('Ctrl Pts',(-1.47261591349647,3.19424234962399,-1.56419538135796));
#12912=CARTESIAN_POINT('Ctrl Pts',(-1.38612102881625,3.18367067658749,-1.64577868387154));
#12913=CARTESIAN_POINT('Ctrl Pts',(-1.29291648826503,3.17309908312012,-1.72044327963702));
#12914=CARTESIAN_POINT('Ctrl Pts',(-1.19420413823089,3.1625275255954,-1.7869012585407));
#12915=CARTESIAN_POINT('Ctrl Pts',(-1.10127855845529,3.15257569979269,-1.84946330086065));
#12916=CARTESIAN_POINT('Ctrl Pts',(-1.0034731816617,3.14262390584207,-1.90475212557082));
#12917=CARTESIAN_POINT('Ctrl Pts',(-0.901821977267037,3.13267210734858,
-1.95172157886228));
#12918=CARTESIAN_POINT('Ctrl Pts',(-0.849390496460778,3.1275389902861,-1.97594832564208));
#12919=CARTESIAN_POINT('Ctrl Pts',(-0.79593626755812,3.122405872015,-1.99796226104316));
#12920=CARTESIAN_POINT('Ctrl Pts',(-0.741660178022841,3.11727274754091,
-2.01774690915893));
#12921=CARTESIAN_POINT('Ctrl Pts',(-0.633624534486916,3.10705534959171,
-2.05712791854301));
#12922=CARTESIAN_POINT('Ctrl Pts',(-0.522430016986537,3.09683790245466,
-2.08764666535729));
#12923=CARTESIAN_POINT('Ctrl Pts',(-0.409527264222796,3.08662043823546,
-2.10925869119181));
#12924=CARTESIAN_POINT('Ctrl Pts',(-0.293519898919739,3.07612201304093,
-2.13146500693302));
#12925=CARTESIAN_POINT('Ctrl Pts',(-0.175707713868161,3.06562356981184,
-2.1442683506305));
#12926=CARTESIAN_POINT('Ctrl Pts',(-0.0576437673723606,3.05512514337599,
-2.14757037715293));
#12927=CARTESIAN_POINT('Ctrl Pts',(-0.00208063382617425,3.05018438468214,
-2.14912437349207));
#12928=CARTESIAN_POINT('Ctrl Pts',(0.0535384230342057,3.04524362970769,
-2.1485732579766));
#12929=CARTESIAN_POINT('Ctrl Pts',(0.109051688665274,3.04030288208286,-2.14590278660309));
#12930=CARTESIAN_POINT('Ctrl Pts',(0.210388807281865,3.03128375625016,-2.14102795405156));
#12931=CARTESIAN_POINT('Ctrl Pts',(0.311481707292144,3.02226465441966,-2.12908060919421));
#12932=CARTESIAN_POINT('Ctrl Pts',(0.411193133653393,3.013245565563,-2.10995375633487));
#12933=CARTESIAN_POINT('Ctrl Pts',(0.478110136128969,3.00719279494911,-2.09711759796421));
#12934=CARTESIAN_POINT('Ctrl Pts',(0.544404650338317,3.00114003017844,-2.08104895318567));
#12935=CARTESIAN_POINT('Ctrl Pts',(0.609733450344373,2.99508726791757,-2.06172867262875));
#12936=CARTESIAN_POINT('Ctrl Pts',(0.706933970211559,2.98608156693525,-2.03298267830558));
#12937=CARTESIAN_POINT('Ctrl Pts',(0.801995196015169,2.97707587150898,-1.99703639806845));
#12938=CARTESIAN_POINT('Ctrl Pts',(0.894009539879667,2.96807017065937,-1.95457232965125));
#12939=CARTESIAN_POINT('Ctrl Pts',(0.910141835246869,2.96649125785085,-1.94712737199109));
#12940=CARTESIAN_POINT('Ctrl Pts',(0.926180537486656,2.96491234487564,-1.93948218095153));
#12941=CARTESIAN_POINT('Ctrl Pts',(0.942120844041218,2.96333343167455,-1.93164057257274));
#12942=CARTESIAN_POINT('Ctrl Pts',(1.04169895621625,2.95347005826233,-1.88265452854005));
#12943=CARTESIAN_POINT('Ctrl Pts',(1.13747236916903,2.94360660484181,-1.82599127228637));
#12944=CARTESIAN_POINT('Ctrl Pts',(1.22844424331902,2.93374313446163,-1.76245278614713));
#12945=CARTESIAN_POINT('Ctrl Pts',(1.31952357108006,2.92386801360685,-1.69883925000107));
#12946=CARTESIAN_POINT('Ctrl Pts',(1.40579110765157,2.91399287575234,-1.62833341128625));
#12947=CARTESIAN_POINT('Ctrl Pts',(1.48621992686302,2.90411778417053,-1.55169643628954));
#12948=CARTESIAN_POINT('Ctrl Pts',(1.53442058880381,2.898199682231,-1.50576821105636));
#12949=CARTESIAN_POINT('Ctrl Pts',(1.58052365801219,2.89228159691056,-1.45763717410918));
#12950=CARTESIAN_POINT('Ctrl Pts',(1.62430103503315,2.88636354182797,-1.40746151925886));
#12951=CARTESIAN_POINT('Ctrl Pts',(1.69173498938177,2.87724746673555,-1.3301717625663));
#12952=CARTESIAN_POINT('Ctrl Pts',(1.75365442585972,2.8681313954874,-1.24801752262837));
#12953=CARTESIAN_POINT('Ctrl Pts',(1.80912283730287,2.85901531580153,-1.16170605324713));
#12954=CARTESIAN_POINT('Ctrl Pts',(1.81220681460461,2.85850847267946,-1.1569072388314));
#12955=CARTESIAN_POINT('Ctrl Pts',(1.81527086018526,2.85800162953131,-1.15209558261765));
#12956=CARTESIAN_POINT('Ctrl Pts',(1.81831481673788,2.85749478635496,-1.14727120926561));
#12957=CARTESIAN_POINT('Ctrl Pts',(1.87318565161585,2.84835835232332,-1.0603063038826));
#12958=CARTESIAN_POINT('Ctrl Pts',(1.92152469700568,2.83922190913028,-0.96920711629221));
#12959=CARTESIAN_POINT('Ctrl Pts',(1.96308343251013,2.83008544441134,-0.87512601001788));
#12960=CARTESIAN_POINT('Ctrl Pts',(1.9944561004723,2.82318833191511,-0.804104231495727));
#12961=CARTESIAN_POINT('Ctrl Pts',(2.02196578264352,2.81629120715186,-0.731383902142148));
#12962=CARTESIAN_POINT('Ctrl Pts',(2.04552456127386,2.80939406480244,-0.657465805531989));
#12963=CARTESIAN_POINT('Ctrl Pts',(2.08241088493445,2.79859510832741,-0.541731162462456));
#12964=CARTESIAN_POINT('Ctrl Pts',(2.10967171517931,2.78779614223852,-0.422897417519029));
#12965=CARTESIAN_POINT('Ctrl Pts',(2.12696593385866,2.77699718589282,-0.302632173723326));
#12966=CARTESIAN_POINT('Ctrl Pts',(2.14377041553965,2.76650403396443,-0.185772596329485));
#12967=CARTESIAN_POINT('Ctrl Pts',(2.15116481342204,2.75601089123524,-0.0675600796035336));
#12968=CARTESIAN_POINT('Ctrl Pts',(2.14878813127568,2.74551777546388,0.0504759594829834));
#12969=CARTESIAN_POINT('Ctrl Pts',(2.14779957088035,2.74115325465865,0.0995720296670876));
#12970=CARTESIAN_POINT('Ctrl Pts',(2.14511995457142,2.73678873851731,0.148637459180571));
#12971=CARTESIAN_POINT('Ctrl Pts',(2.14072071578196,2.73242422831781,0.19756138083896));
#12972=CARTESIAN_POINT('Ctrl Pts',(2.13651687479091,2.72825357340213,0.244312284155051));
#12973=CARTESIAN_POINT('Ctrl Pts',(2.13074439087573,2.72408292230982,0.290913680125547));
#12974=CARTESIAN_POINT('Ctrl Pts',(2.12338297676972,2.71991227241574,0.337260632528063));
#12975=CARTESIAN_POINT('Ctrl Pts',(2.10352655248463,2.70866250536706,0.462275301988544));
#12976=CARTESIAN_POINT('Ctrl Pts',(2.0721060016905,2.69741274703639,0.585437161112324));
#12977=CARTESIAN_POINT('Ctrl Pts',(2.03016918451094,2.68616294590418,0.704921112297282));
#12978=CARTESIAN_POINT('Ctrl Pts',(1.99201131259478,2.67592686935963,0.81363831145501));
#12979=CARTESIAN_POINT('Ctrl Pts',(1.94514810499035,2.66569075737976,0.919309952190526));
#12980=CARTESIAN_POINT('Ctrl Pts',(1.89039889086094,2.65545457115502,1.0205837859347));
#12981=CARTESIAN_POINT('Ctrl Pts',(1.80901360106348,2.64023837133247,1.17112841820445));
#12982=CARTESIAN_POINT('Ctrl Pts',(1.70998760896235,2.62502233564322,1.31236306612878));
#12983=CARTESIAN_POINT('Ctrl Pts',(1.59571189358983,2.60980632287908,1.43987397263786));
#12984=CARTESIAN_POINT('Ctrl Pts',(1.52693807041457,2.6006489671989,1.51661304627731));
#12985=CARTESIAN_POINT('Ctrl Pts',(1.45264173282485,2.591491619822,1.5883807320115));
#12986=CARTESIAN_POINT('Ctrl Pts',(1.3733508076554,2.58233424996849,1.6542090433471));
#12987=CARTESIAN_POINT('Ctrl Pts',(1.36224054081993,2.58105111671754,1.66343292492881));
#12988=CARTESIAN_POINT('Ctrl Pts',(1.35103221931852,2.57976798302529,1.6725401883537));
#12989=CARTESIAN_POINT('Ctrl Pts',(1.33972865760694,2.57848484880706,1.68152979797504));
#12990=CARTESIAN_POINT('Ctrl Pts',(1.23494836182595,2.56659061702923,1.76486051966376));
#12991=CARTESIAN_POINT('Ctrl Pts',(1.122164294256,2.55469639933387,1.83794380682689));
#12992=CARTESIAN_POINT('Ctrl Pts',(1.00362766456432,2.54280216347611,1.90008356090546));
#12993=CARTESIAN_POINT('Ctrl Pts',(0.878254391920993,2.53022192326716,1.96580724775522));
#12994=CARTESIAN_POINT('Ctrl Pts',(0.746444791840392,2.51764166274032,2.01928946994072));
#12995=CARTESIAN_POINT('Ctrl Pts',(0.610817914220216,2.50506134374346,2.05967163702932));
#12996=CARTESIAN_POINT('Ctrl Pts',(0.598073850852332,2.50387924484612,2.06346611276554));
#12997=CARTESIAN_POINT('Ctrl Pts',(0.585296060455977,2.50269714543254,2.06714489505422));
#12998=CARTESIAN_POINT('Ctrl Pts',(0.572486702820834,2.50151504547105,2.07070725264017));
#12999=CARTESIAN_POINT('Ctrl Pts',(0.465857401602194,2.49167485703586,2.10036148752846));
#13000=CARTESIAN_POINT('Ctrl Pts',(0.356869727964285,2.48183472835482,2.12199121968651));
#13001=CARTESIAN_POINT('Ctrl Pts',(0.246875167750652,2.47199463026813,2.13508829993763));
#13002=CARTESIAN_POINT('Ctrl Pts',(0.145383698683764,2.46291521753498,2.14717291496397));
#13003=CARTESIAN_POINT('Ctrl Pts',(0.04303616977167,2.45383583084887,2.15199328339809));
#13004=CARTESIAN_POINT('Ctrl Pts',(-0.0590937688555852,2.44475644730326,
2.14918773647839));
#13005=CARTESIAN_POINT('Ctrl Pts',(-0.134875091103585,2.43801946400991,
2.14710599572674));
#13006=CARTESIAN_POINT('Ctrl Pts',(-0.2105363151451,2.43128248244564,2.14082641582439));
#13007=CARTESIAN_POINT('Ctrl Pts',(-0.285647338284483,2.42454549325238,
2.13052149366505));
#13008=CARTESIAN_POINT('Ctrl Pts',(-0.396965761014252,2.41456092667886,
2.11524906582178));
#13009=CARTESIAN_POINT('Ctrl Pts',(-0.507018890481444,2.40457629337122,
2.09114945184087));
#13010=CARTESIAN_POINT('Ctrl Pts',(-0.6145848234177,2.39459164121287,2.05877934147919));
#13011=CARTESIAN_POINT('Ctrl Pts',(-0.724190762137535,2.38441762846799,
2.02579532659821));
#13012=CARTESIAN_POINT('Ctrl Pts',(-0.831215595269355,2.37424359615059,
1.98422376310785));
#13013=CARTESIAN_POINT('Ctrl Pts',(-0.934359320682798,2.3640695949205,1.93460088691591));
#13014=CARTESIAN_POINT('Ctrl Pts',(-0.990097929254591,2.35857159036521,
1.90778481001756));
#13015=CARTESIAN_POINT('Ctrl Pts',(-1.04470289635645,2.35307359488832,1.87861664475033));
#13016=CARTESIAN_POINT('Ctrl Pts',(-1.09796608325633,2.34757561648456,1.84717540290619));
#13017=CARTESIAN_POINT('Ctrl Pts',(-1.18421742323335,2.33867250662407,1.79626126506656));
#13018=CARTESIAN_POINT('Ctrl Pts',(-1.26701772081672,2.32976941108325,1.73934057733943));
#13019=CARTESIAN_POINT('Ctrl Pts',(-1.34533819526139,2.32086632059572,1.67681359440466));
#13020=CARTESIAN_POINT('Ctrl Pts',(-1.38550722784109,2.31630010040375,1.64474473332553));
#13021=CARTESIAN_POINT('Ctrl Pts',(-1.42449815487176,2.31173388154103,1.61120193998494));
#13022=CARTESIAN_POINT('Ctrl Pts',(-1.46217489296344,2.30716766275741,1.57624382072239));
#13023=CARTESIAN_POINT('Ctrl Pts',(-1.53563328275405,2.29826489950704,1.50808592592571));
#13024=CARTESIAN_POINT('Ctrl Pts',(-1.60409331664952,2.28936213655732,1.43454604043423));
#13025=CARTESIAN_POINT('Ctrl Pts',(-1.66706033649241,2.28045936464286,1.35660998984868));
#13026=CARTESIAN_POINT('Ctrl Pts',(-1.69029001396386,2.27717497035691,1.32785796501062));
#13027=CARTESIAN_POINT('Ctrl Pts',(-1.71277250270999,2.27389057485086,1.29850792734728));
#13028=CARTESIAN_POINT('Ctrl Pts',(-1.73448450182989,2.27060617765949,1.26861028057278));
#13029=CARTESIAN_POINT('Ctrl Pts',(-1.79972704223425,2.26073686920573,1.17877062937763));
#13030=CARTESIAN_POINT('Ctrl Pts',(-1.85806026613614,2.25086748884915,1.08392925964598));
#13031=CARTESIAN_POINT('Ctrl Pts',(-1.90894278137274,2.2409980982588,0.985246190110895));
#13032=CARTESIAN_POINT('Ctrl Pts',(-1.95948299046544,2.23119510283425,0.887226999333456));
#13033=CARTESIAN_POINT('Ctrl Pts',(-2.00267295250023,2.22139209731318,0.785416381034645));
#13034=CARTESIAN_POINT('Ctrl Pts',(-2.03793790884311,2.21158914212838,0.680927388260187));
#13035=CARTESIAN_POINT('Ctrl Pts',(-2.05946575212243,2.20560483065381,0.617141043567426));
#13036=CARTESIAN_POINT('Ctrl Pts',(-2.07803935625401,2.19962053793762,0.552356188959628));
#13037=CARTESIAN_POINT('Ctrl Pts',(-2.09351843408538,2.19363627772794,0.486824635297257));
#13038=CARTESIAN_POINT('Ctrl Pts',(-2.11426298230575,2.1856163700929,0.399001414191062));
#13039=CARTESIAN_POINT('Ctrl Pts',(-2.12944394678572,2.17759645972531,0.309845908133398));
#13040=CARTESIAN_POINT('Ctrl Pts',(-2.13870728451891,2.16957654356607,0.22007078798899));
#13041=CARTESIAN_POINT('Ctrl Pts',(-2.1494919731514,2.16023948805461,0.115551580594407));
#13042=CARTESIAN_POINT('Ctrl Pts',(-2.15225428035161,2.15090242469288,0.0101933317018818));
#13043=CARTESIAN_POINT('Ctrl Pts',(-2.14728720710796,2.14156534865332,-0.0948041580853045));
#13044=CARTESIAN_POINT('Ctrl Pts',(-2.14287211193829,2.13326587785856,-0.188133546891817));
#13045=CARTESIAN_POINT('Ctrl Pts',(-2.13235100881986,2.12496639704717,-0.28117718946733));
#13046=CARTESIAN_POINT('Ctrl Pts',(-2.1159636378089,2.11666690282892,-0.373098825557915));
#13047=CARTESIAN_POINT('Ctrl Pts',(2.551614418722,6.316751913189,-1.211595605458));
#13048=CARTESIAN_POINT('Ctrl Pts',(2.842552710281,6.270890802077,-0.598880986523));
#13049=CARTESIAN_POINT('Ctrl Pts',(2.962035735699,6.179168579855,0.8419695182761));
#13050=CARTESIAN_POINT('Ctrl Pts',(1.670619315018,6.041585246522,2.587364402054));
#13051=CARTESIAN_POINT('Ctrl Pts',(-0.4512378705897,5.904001913189,3.046441196415));
#13052=CARTESIAN_POINT('Ctrl Pts',(-2.348791901428,5.766418579855,1.991932600627));
#13053=CARTESIAN_POINT('Ctrl Pts',(-3.079263577893,5.628835246522,-0.05240707813364));
#13054=CARTESIAN_POINT('Ctrl Pts',(-2.279655662895,5.491251913189,-2.07069305665));
#13055=CARTESIAN_POINT('Ctrl Pts',(-0.3472977925631,5.353668579855,-3.060063551872));
#13056=CARTESIAN_POINT('Ctrl Pts',(1.757631370145,5.216085246522,-2.528900044009));
#13057=CARTESIAN_POINT('Ctrl Pts',(2.989200566047,5.078501913189,-0.7411366794348));
#13058=CARTESIAN_POINT('Ctrl Pts',(2.735448240199,4.940918579855,1.414894540471));
#13059=CARTESIAN_POINT('Ctrl Pts',(1.122462847131,4.803335246522,2.86787042401));
#13060=CARTESIAN_POINT('Ctrl Pts',(-1.048269748206,4.665751913189,2.895813211186));
#13061=CARTESIAN_POINT('Ctrl Pts',(-2.698121387469,4.528168579855,1.484838239147));
#13062=CARTESIAN_POINT('Ctrl Pts',(-3.007287528446,4.390585246522,-0.6639467894038));
#13063=CARTESIAN_POINT('Ctrl Pts',(-1.822144778546,4.253001913189,-2.482819369995));
#13064=CARTESIAN_POINT('Ctrl Pts',(0.2684142700615,4.115418579855,-3.067989145611));
#13065=CARTESIAN_POINT('Ctrl Pts',(2.225599364098,3.977835246522,-2.12868764466));
#13066=CARTESIAN_POINT('Ctrl Pts',(3.076893223598,3.840251913189,-0.1316499467573));
#13067=CARTESIAN_POINT('Ctrl Pts',(2.399291406589,3.702668579855,1.930804071939));
#13068=CARTESIAN_POINT('Ctrl Pts',(0.5294914882953,3.565085246522,3.03384943313));
#13069=CARTESIAN_POINT('Ctrl Pts',(-1.603410587237,3.427501913189,2.629387400296));
#13070=CARTESIAN_POINT('Ctrl Pts',(-2.939584493455,3.289918579855,0.9183935111373));
#13071=CARTESIAN_POINT('Ctrl Pts',(-2.815090858966,3.152335246522,-1.248946378924));
#13072=CARTESIAN_POINT('Ctrl Pts',(-1.291790116112,3.014751913189,-2.795689854368));
#13073=CARTESIAN_POINT('Ctrl Pts',(0.8733960180478,2.877168579855,-2.953266681808));
#13074=CARTESIAN_POINT('Ctrl Pts',(2.604594646812,2.739585246522,-1.643376524728));
#13075=CARTESIAN_POINT('Ctrl Pts',(3.041583038692,2.602001913189,0.4830976119985));
#13076=CARTESIAN_POINT('Ctrl Pts',(1.967213008604,2.464418579855,2.369534101977));
#13077=CARTESIAN_POINT('Ctrl Pts',(-0.08462640871746,2.326835246522,3.078515543247));
#13078=CARTESIAN_POINT('Ctrl Pts',(-2.094529967139,2.189251913189,2.257956523383));
#13079=CARTESIAN_POINT('Ctrl Pts',(-3.063242229715,2.051668579855,0.3148260017099));
#13080=CARTESIAN_POINT('Ctrl Pts',(-2.695373355482,1.959946357633,-1.083386736722));
#13081=CARTESIAN_POINT('Ctrl Pts',(-2.302458293298,1.914085246522,-1.63627193969));
#13082=CARTESIAN_POINT('Ctrl Pts',(2.566245858361,6.354663466539,-1.218543123796));
#13083=CARTESIAN_POINT('Ctrl Pts',(2.858852445106,6.308802355428,-0.6023150833602));
#13084=CARTESIAN_POINT('Ctrl Pts',(2.979020608788,6.217080133205,0.8467975307274));
#13085=CARTESIAN_POINT('Ctrl Pts',(1.680198962119,6.079496799872,2.602200838859));
#13086=CARTESIAN_POINT('Ctrl Pts',(-0.4538253538779,5.941913466539,3.063910066379));
#13087=CARTESIAN_POINT('Ctrl Pts',(-2.362260318395,5.804330133205,2.003354718874));
#13088=CARTESIAN_POINT('Ctrl Pts',(-3.0969206576,5.666746799872,-0.05270759023089));
#13089=CARTESIAN_POINT('Ctrl Pts',(-2.292727639595,5.529163466539,-2.082566802247));
#13090=CARTESIAN_POINT('Ctrl Pts',(-0.3492892637867,5.391580133205,-3.077610534999));
#13091=CARTESIAN_POINT('Ctrl Pts',(1.767709960825,5.253996799872,-2.543401235127));
#13092=CARTESIAN_POINT('Ctrl Pts',(3.006341207411,5.116413466539,-0.7453864973187));
#13093=CARTESIAN_POINT('Ctrl Pts',(2.751133817737,4.978830133205,1.423007813351));
#13094=CARTESIAN_POINT('Ctrl Pts',(1.128899261377,4.841246799872,2.884315335393));
#13095=CARTESIAN_POINT('Ctrl Pts',(-1.054280725191,4.703663466539,2.912418351796));
#13096=CARTESIAN_POINT('Ctrl Pts',(-2.713592925774,4.566080133205,1.493352582423));
#13097=CARTESIAN_POINT('Ctrl Pts',(-3.024531883873,4.428496799872,-0.66775398586));
#13098=CARTESIAN_POINT('Ctrl Pts',(-1.832593301311,4.290913466539,-2.497056325814));
#13099=CARTESIAN_POINT('Ctrl Pts',(0.2699534082486,4.153330133205,-3.085581575591));
#13100=CARTESIAN_POINT('Ctrl Pts',(2.238361371758,4.015746799872,-2.140893942192));
#13101=CARTESIAN_POINT('Ctrl Pts',(3.094536711245,3.878163466539,-0.1324048524497));
#13102=CARTESIAN_POINT('Ctrl Pts',(2.413049397269,3.740580133205,1.941875667641));
#13103=CARTESIAN_POINT('Ctrl Pts',(0.5325276926267,3.602996799872,3.051246099542));
#13104=CARTESIAN_POINT('Ctrl Pts',(-1.612604846782,3.465413466539,2.64446480492));
#13105=CARTESIAN_POINT('Ctrl Pts',(-2.956440626875,3.327830133205,0.923659753217));
#13106=CARTESIAN_POINT('Ctrl Pts',(-2.831233122342,3.190246799872,-1.256108073662));
#13107=CARTESIAN_POINT('Ctrl Pts',(-1.299197484941,3.052663466539,-2.811720868715));
#13108=CARTESIAN_POINT('Ctrl Pts',(0.8784042359921,2.915080133205,-2.970201271484));
#13109=CARTESIAN_POINT('Ctrl Pts',(2.619529885098,2.777496799872,-1.652799956517));
#13110=CARTESIAN_POINT('Ctrl Pts',(3.059024051061,2.639913466539,0.4858677850693));
#13111=CARTESIAN_POINT('Ctrl Pts',(1.978493380035,2.502330133205,2.383121458644));
#13112=CARTESIAN_POINT('Ctrl Pts',(-0.08511167254962,2.364746799872,3.096168333582));
#13113=CARTESIAN_POINT('Ctrl Pts',(-2.106540398089,2.227163466539,2.270904073113));
#13114=CARTESIAN_POINT('Ctrl Pts',(-3.080807439981,2.089580133205,0.3166312735437));
#13115=CARTESIAN_POINT('Ctrl Pts',(-2.710829136052,1.997857910983,-1.089599081161));
#13116=CARTESIAN_POINT('Ctrl Pts',(-2.315661024593,1.951996799872,-1.645654632444));
#13117=CARTESIAN_POINT('Ctrl Pts',(2.610640441769,6.569665066603,-1.239623221859));
#13118=CARTESIAN_POINT('Ctrl Pts',(2.908308954861,6.523803955492,-0.6127347892973));
#13119=CARTESIAN_POINT('Ctrl Pts',(3.030555958942,6.432081733269,0.8614466429648));
#13120=CARTESIAN_POINT('Ctrl Pts',(1.709265441748,6.294498399936,2.647217422835));
#13121=CARTESIAN_POINT('Ctrl Pts',(-0.4616762725496,6.156915066603,3.116913955525));
#13122=CARTESIAN_POINT('Ctrl Pts',(-2.403126068804,6.019331733269,2.038011607992));
#13123=CARTESIAN_POINT('Ctrl Pts',(-3.150495611065,5.881748399936,-0.05361940135107));
#13124=CARTESIAN_POINT('Ctrl Pts',(-2.332390514489,5.744165066603,-2.118594015035));
#13125=CARTESIAN_POINT('Ctrl Pts',(-0.3553317679779,5.606581733269,-3.130851434404));
#13126=CARTESIAN_POINT('Ctrl Pts',(1.798290330606,5.468998399936,-2.587400619639));
#13127=CARTESIAN_POINT('Ctrl Pts',(3.058349188273,5.331415066603,-0.7582812567662));
#13128=CARTESIAN_POINT('Ctrl Pts',(2.798726856939,5.193831733269,1.447625033425));
#13129=CARTESIAN_POINT('Ctrl Pts',(1.148428571967,5.056248399936,2.934212338565));
#13130=CARTESIAN_POINT('Ctrl Pts',(-1.072519177847,4.918665066603,2.962801521053));
#13131=CARTESIAN_POINT('Ctrl Pts',(-2.760536529048,4.781081733269,1.519186726709));
#13132=CARTESIAN_POINT('Ctrl Pts',(-3.076854553017,4.643498399936,-0.679305747327));
#13133=CARTESIAN_POINT('Ctrl Pts',(-1.864296115717,4.505915066603,-2.540253969941));
#13134=CARTESIAN_POINT('Ctrl Pts',(0.2746234475825,4.368331733269,-3.138960369433));
#13135=CARTESIAN_POINT('Ctrl Pts',(2.27708374136,4.230748399936,-2.177930181092));
#13136=CARTESIAN_POINT('Ctrl Pts',(3.148070423804,4.093165066603,-0.1346953805558));
#13137=CARTESIAN_POINT('Ctrl Pts',(2.454793769651,3.955581733269,1.975469004389));
#13138=CARTESIAN_POINT('Ctrl Pts',(0.5417401166782,3.817998399936,3.104030909316));
#13139=CARTESIAN_POINT('Ctrl Pts',(-1.640501986934,3.680415066603,2.6902125313));
#13140=CARTESIAN_POINT('Ctrl Pts',(-3.007585356276,3.542831733269,0.9396385378769));
#13141=CARTESIAN_POINT('Ctrl Pts',(-2.880211833633,3.405248399936,-1.27783802384));
#13142=CARTESIAN_POINT('Ctrl Pts',(-1.321672857253,3.267665066603,-2.860362029195));
#13143=CARTESIAN_POINT('Ctrl Pts',(0.8936001261264,3.130081733269,-3.021584052154));
#13144=CARTESIAN_POINT('Ctrl Pts',(2.664846251648,2.992498399936,-1.681392449043));
#13145=CARTESIAN_POINT('Ctrl Pts',(3.11194341494,2.854915066603,0.4942730194467));
#13146=CARTESIAN_POINT('Ctrl Pts',(2.012720182232,2.717331733269,2.424348094831));
#13147=CARTESIAN_POINT('Ctrl Pts',(-0.08658405573291,2.579748399936,3.149730272273));
#13148=CARTESIAN_POINT('Ctrl Pts',(-2.142982340353,2.442165066603,2.310189412808));
#13149=CARTESIAN_POINT('Ctrl Pts',(-3.134103644012,2.304581733269,0.3221088132102));
#13150=CARTESIAN_POINT('Ctrl Pts',(-2.757724927347,2.212859511047,-1.108448521144));
#13151=CARTESIAN_POINT('Ctrl Pts',(-2.355720633912,2.166998399936,-1.674123514957));
#13152=CARTESIAN_POINT('Ctrl Pts',(2.258338232158,6.959666666667,-1.072337833508));
#13153=CARTESIAN_POINT('Ctrl Pts',(2.51583680334,6.913805555556,-0.5300471021225));
#13154=CARTESIAN_POINT('Ctrl Pts',(2.621586748321,6.822083333333,0.7451956453465));
#13155=CARTESIAN_POINT('Ctrl Pts',(1.478602504675,6.6845,2.289979201721));
#13156=CARTESIAN_POINT('Ctrl Pts',(-0.3993737170763,6.546916666667,2.696290856254));
#13157=CARTESIAN_POINT('Ctrl Pts',(-2.078827628288,6.409333333333,1.762984843976));
#13158=CARTESIAN_POINT('Ctrl Pts',(-2.725340715205,6.27175,-0.04638353950209));
#13159=CARTESIAN_POINT('Ctrl Pts',(-2.017637736288,6.134166666667,-1.832692769952));
#13160=CARTESIAN_POINT('Ctrl Pts',(-0.3073802519435,5.996583333333,-2.708347492208));
#13161=CARTESIAN_POINT('Ctrl Pts',(1.555613611568,5.859,-2.238234590927));
#13162=CARTESIAN_POINT('Ctrl Pts',(2.645629320936,5.721416666667,-0.6559522810899));
#13163=CARTESIAN_POINT('Ctrl Pts',(2.421042653468,5.583833333333,1.252270096834));
#13164=CARTESIAN_POINT('Ctrl Pts',(0.9934497717423,5.44625,2.538244562304));
#13165=CARTESIAN_POINT('Ctrl Pts',(-0.9277842422502,5.308666666667,2.562975675332));
#13166=CARTESIAN_POINT('Ctrl Pts',(-2.388006055937,5.171083333333,1.314174641526));
#13167=CARTESIAN_POINT('Ctrl Pts',(-2.661637413063,5.0335,-0.5876344041747));
#13168=CARTESIAN_POINT('Ctrl Pts',(-1.612712009983,4.895916666667,-2.19745031446));
#13169=CARTESIAN_POINT('Ctrl Pts',(0.2375634044427,4.758333333333,-2.715362138003));
#13170=CARTESIAN_POINT('Ctrl Pts',(1.969794533427,4.62075,-1.884021604905));
#13171=CARTESIAN_POINT('Ctrl Pts',(2.723242803511,4.483166666667,-0.1165184307794));
#13172=CARTESIAN_POINT('Ctrl Pts',(2.12352284649,4.345583333333,1.708882275658));
#13173=CARTESIAN_POINT('Ctrl Pts',(0.4686330594646,4.208,2.685146358783));
#13174=CARTESIAN_POINT('Ctrl Pts',(-1.419118580157,4.070416666667,2.327172181531));
#13175=CARTESIAN_POINT('Ctrl Pts',(-2.601715995771,3.932833333333,0.812835655399));
#13176=CARTESIAN_POINT('Ctrl Pts',(-2.491531348606,3.79525,-1.105395602386));
#13177=CARTESIAN_POINT('Ctrl Pts',(-1.143314987458,3.657666666667,-2.474360247008));
#13178=CARTESIAN_POINT('Ctrl Pts',(0.7730100617475,3.520083333333,-2.613825587577));
#13179=CARTESIAN_POINT('Ctrl Pts',(2.305229045192,3.3825,-1.45449093264));
#13180=CARTESIAN_POINT('Ctrl Pts',(2.691991083042,3.244916666667,0.4275715794031));
#13181=CARTESIAN_POINT('Ctrl Pts',(1.741106460104,3.107333333333,2.097185772127));
#13182=CARTESIAN_POINT('Ctrl Pts',(-0.07489966072249,2.96975,2.724678657793));
#13183=CARTESIAN_POINT('Ctrl Pts',(-1.853789925502,2.832166666667,1.998432641661));
#13184=CARTESIAN_POINT('Ctrl Pts',(-2.711160820761,2.694583333333,0.2786406876064));
#13185=CARTESIAN_POINT('Ctrl Pts',(-2.385573875881,2.602861111111,-0.9588649718392));
#13186=CARTESIAN_POINT('Ctrl Pts',(-2.037819489321,2.557,-1.448202930857));
#13187=CARTESIAN_POINT('Ctrl Pts',(1.906036022547,6.569665066603,-0.905052445157));
#13188=CARTESIAN_POINT('Ctrl Pts',(2.123364651819,6.523803955492,-0.4473594149477));
#13189=CARTESIAN_POINT('Ctrl Pts',(2.212617537701,6.432081733269,0.6289446477281));
#13190=CARTESIAN_POINT('Ctrl Pts',(1.247939567603,6.294498399936,1.932740980607));
#13191=CARTESIAN_POINT('Ctrl Pts',(-0.337071161603,6.156915066603,2.275667756983));
#13192=CARTESIAN_POINT('Ctrl Pts',(-1.754529187773,6.019331733269,1.487958079961));
#13193=CARTESIAN_POINT('Ctrl Pts',(-2.300185819346,5.881748399936,-0.03914767765311));
#13194=CARTESIAN_POINT('Ctrl Pts',(-1.702884958088,5.744165066603,-1.54679152487));
#13195=CARTESIAN_POINT('Ctrl Pts',(-0.2594287359091,5.606581733269,-2.285843550012));
#13196=CARTESIAN_POINT('Ctrl Pts',(1.312936892531,5.468998399936,-1.889068562215));
#13197=CARTESIAN_POINT('Ctrl Pts',(2.2329094536,5.331415066603,-0.5536233054136));
#13198=CARTESIAN_POINT('Ctrl Pts',(2.043358449998,5.193831733269,1.056915160243));
#13199=CARTESIAN_POINT('Ctrl Pts',(0.8384709715172,5.056248399936,2.142276786043));
#13200=CARTESIAN_POINT('Ctrl Pts',(-0.7830493066535,4.918665066603,2.16314982961));
#13201=CARTESIAN_POINT('Ctrl Pts',(-2.015475582826,4.781081733269,1.109162556342));
#13202=CARTESIAN_POINT('Ctrl Pts',(-2.246420273109,4.643498399936,-0.4959630610224));
#13203=CARTESIAN_POINT('Ctrl Pts',(-1.361127904248,4.505915066603,-1.85464665898));
#13204=CARTESIAN_POINT('Ctrl Pts',(0.200503361303,4.368331733269,-2.291763906573));
#13205=CARTESIAN_POINT('Ctrl Pts',(1.662505325493,4.230748399936,-1.590113028717));
#13206=CARTESIAN_POINT('Ctrl Pts',(2.298415183218,4.093165066603,-0.09834148100305));
#13207=CARTESIAN_POINT('Ctrl Pts',(1.792251923328,3.955581733269,1.442295546927));
#13208=CARTESIAN_POINT('Ctrl Pts',(0.395526002251,3.817998399936,2.266261808251));
#13209=CARTESIAN_POINT('Ctrl Pts',(-1.19773517338,3.680415066603,1.964131831763));
#13210=CARTESIAN_POINT('Ctrl Pts',(-2.195846635266,3.542831733269,0.6860327729212));
#13211=CARTESIAN_POINT('Ctrl Pts',(-2.10285086358,3.405248399936,-0.9329531809324));
#13212=CARTESIAN_POINT('Ctrl Pts',(-0.964957117664,3.267665066603,-2.088358464821));
#13213=CARTESIAN_POINT('Ctrl Pts',(0.6524199973687,3.130081733269,-2.206067123));
#13214=CARTESIAN_POINT('Ctrl Pts',(1.945611838737,2.992498399936,-1.227589416237));
#13215=CARTESIAN_POINT('Ctrl Pts',(2.272038751145,2.854915066603,0.3608701393595));
#13216=CARTESIAN_POINT('Ctrl Pts',(1.469492737975,2.717331733269,1.770023449422));
#13217=CARTESIAN_POINT('Ctrl Pts',(-0.06321526571209,2.579748399936,2.299627043313));
#13218=CARTESIAN_POINT('Ctrl Pts',(-1.56459751065,2.442165066603,1.686675870514));
#13219=CARTESIAN_POINT('Ctrl Pts',(-2.28821799751,2.304581733269,0.2351725620026));
#13220=CARTESIAN_POINT('Ctrl Pts',(-2.013422824415,2.212859511047,-0.8092814225342));
#13221=CARTESIAN_POINT('Ctrl Pts',(-1.719918344731,2.166998399936,-1.222282346756));
#13222=CARTESIAN_POINT('Ctrl Pts',(1.950430605956,6.354663466539,-0.9261325432193));
#13223=CARTESIAN_POINT('Ctrl Pts',(2.172821161573,6.308802355428,-0.4577791208848));
#13224=CARTESIAN_POINT('Ctrl Pts',(2.264152887855,6.217080133205,0.6435937599656));
#13225=CARTESIAN_POINT('Ctrl Pts',(1.277006047232,6.079496799872,1.977757564583));
#13226=CARTESIAN_POINT('Ctrl Pts',(-0.3449220802747,5.941913466539,2.328671646129));
#13227=CARTESIAN_POINT('Ctrl Pts',(-1.795394938182,5.804330133205,1.522614969079));
#13228=CARTESIAN_POINT('Ctrl Pts',(-2.353760772811,5.666746799872,-0.04005948877329));
#13229=CARTESIAN_POINT('Ctrl Pts',(-1.742547832982,5.529163466539,-1.582818737658));
#13230=CARTESIAN_POINT('Ctrl Pts',(-0.2654712401003,5.391580133205,-2.339084449417));
#13231=CARTESIAN_POINT('Ctrl Pts',(1.343517262312,5.253996799872,-1.933067946727));
#13232=CARTESIAN_POINT('Ctrl Pts',(2.284917434461,5.116413466539,-0.5665180648611));
#13233=CARTESIAN_POINT('Ctrl Pts',(2.0909514892,4.978830133205,1.081532380318));
#13234=CARTESIAN_POINT('Ctrl Pts',(0.8580002821075,4.841246799872,2.192173789215));
#13235=CARTESIAN_POINT('Ctrl Pts',(-0.8012877593092,4.703663466539,2.213532998868));
#13236=CARTESIAN_POINT('Ctrl Pts',(-2.0624191861,4.566080133205,1.134996700628));
#13237=CARTESIAN_POINT('Ctrl Pts',(-2.298742942253,4.428496799872,-0.5075148224894));
#13238=CARTESIAN_POINT('Ctrl Pts',(-1.392830718655,4.290913466539,-1.897844303107));
#13239=CARTESIAN_POINT('Ctrl Pts',(0.2051734006369,4.153330133205,-2.345142700415));
#13240=CARTESIAN_POINT('Ctrl Pts',(1.701227695095,4.015746799872,-1.627149267617));
#13241=CARTESIAN_POINT('Ctrl Pts',(2.351948895778,3.878163466539,-0.1006320091092));
#13242=CARTESIAN_POINT('Ctrl Pts',(1.833996295711,3.740580133205,1.475888883674));
#13243=CARTESIAN_POINT('Ctrl Pts',(0.4047384263025,3.602996799872,2.319046618024));
#13244=CARTESIAN_POINT('Ctrl Pts',(-1.225632313532,3.465413466539,2.009879558143));
#13245=CARTESIAN_POINT('Ctrl Pts',(-2.246991364667,3.327830133205,0.7020115575811));
#13246=CARTESIAN_POINT('Ctrl Pts',(-2.151829574871,3.190246799872,-0.9546831311102));
#13247=CARTESIAN_POINT('Ctrl Pts',(-0.9874324899755,3.052663466539,-2.1369996253));
#13248=CARTESIAN_POINT('Ctrl Pts',(0.6676158875029,2.915080133205,-2.25744990367));
#13249=CARTESIAN_POINT('Ctrl Pts',(1.990928205287,2.777496799872,-1.256181908764));
#13250=CARTESIAN_POINT('Ctrl Pts',(2.324958115024,2.639913466539,0.3692753737369));
#13251=CARTESIAN_POINT('Ctrl Pts',(1.503719540172,2.502330133205,1.811250085609));
#13252=CARTESIAN_POINT('Ctrl Pts',(-0.06468764889537,2.364746799872,2.353188982004));
#13253=CARTESIAN_POINT('Ctrl Pts',(-1.601039452915,2.227163466539,1.725961210209));
#13254=CARTESIAN_POINT('Ctrl Pts',(-2.34151420154,2.089580133205,0.2406501016691));
#13255=CARTESIAN_POINT('Ctrl Pts',(-2.060318615711,1.997857910983,-0.8281308625178));
#13256=CARTESIAN_POINT('Ctrl Pts',(-1.759977954049,1.951996799872,-1.250751229269));
#13257=CARTESIAN_POINT('Ctrl Pts',(1.965062045595,6.316751913189,-0.9330800615582));
#13258=CARTESIAN_POINT('Ctrl Pts',(2.189120896398,6.270890802077,-0.461213217722));
#13259=CARTESIAN_POINT('Ctrl Pts',(2.281137760944,6.179168579855,0.6484217724168));
#13260=CARTESIAN_POINT('Ctrl Pts',(1.286585694332,6.041585246522,1.992594001388));
#13261=CARTESIAN_POINT('Ctrl Pts',(-0.3475095635628,5.904001913189,2.346140516093));
#13262=CARTESIAN_POINT('Ctrl Pts',(-1.808863355149,5.766418579855,1.534037087326));
#13263=CARTESIAN_POINT('Ctrl Pts',(-2.371417852518,5.628835246522,-0.04036000087055));
#13264=CARTESIAN_POINT('Ctrl Pts',(-1.755619809682,5.491251913189,-1.594692483255));
#13265=CARTESIAN_POINT('Ctrl Pts',(-0.2674627113239,5.353668579855,-2.356631432544));
#13266=CARTESIAN_POINT('Ctrl Pts',(1.353595852992,5.216085246522,-1.947569137845));
#13267=CARTESIAN_POINT('Ctrl Pts',(2.302058075825,5.078501913189,-0.570767882745));
#13268=CARTESIAN_POINT('Ctrl Pts',(2.106637066738,4.940918579855,1.089645653198));
#13269=CARTESIAN_POINT('Ctrl Pts',(0.8644366963533,4.803335246522,2.208618700598));
#13270=CARTESIAN_POINT('Ctrl Pts',(-0.8072987362944,4.665751913189,2.230138139478));
#13271=CARTESIAN_POINT('Ctrl Pts',(-2.077890724405,4.528168579855,1.143511043905));
#13272=CARTESIAN_POINT('Ctrl Pts',(-2.31598729768,4.390585246522,-0.5113220189456));
#13273=CARTESIAN_POINT('Ctrl Pts',(-1.403279241419,4.253001913189,-1.912081258926));
#13274=CARTESIAN_POINT('Ctrl Pts',(0.206712538824,4.115418579855,-2.362735130395));
#13275=CARTESIAN_POINT('Ctrl Pts',(1.713989702755,3.977835246522,-1.639355565149));
#13276=CARTESIAN_POINT('Ctrl Pts',(2.369592383424,3.840251913189,-0.1013869148015));
#13277=CARTESIAN_POINT('Ctrl Pts',(1.847754286391,3.702668579855,1.486960479376));
#13278=CARTESIAN_POINT('Ctrl Pts',(0.4077746306339,3.565085246522,2.336443284436));
#13279=CARTESIAN_POINT('Ctrl Pts',(-1.234826573077,3.427501913189,2.024956962767));
#13280=CARTESIAN_POINT('Ctrl Pts',(-2.263847498087,3.289918579855,0.7072777996607));
#13281=CARTESIAN_POINT('Ctrl Pts',(-2.167971838247,3.152335246522,-0.961844825848));
#13282=CARTESIAN_POINT('Ctrl Pts',(-0.9948398588049,3.014751913189,-2.153030639647));
#13283=CARTESIAN_POINT('Ctrl Pts',(0.6726241054473,2.877168579855,-2.274384493346));
#13284=CARTESIAN_POINT('Ctrl Pts',(2.005863443573,2.739585246522,-1.265605340552));
#13285=CARTESIAN_POINT('Ctrl Pts',(2.342399127393,2.602001913189,0.3720455468077));
#13286=CARTESIAN_POINT('Ctrl Pts',(1.514999911603,2.464418579855,1.824837442277));
#13287=CARTESIAN_POINT('Ctrl Pts',(-0.06517291272752,2.326835246522,2.370841772339));
#13288=CARTESIAN_POINT('Ctrl Pts',(-1.613049883864,2.189251913189,1.738908759939));
#13289=CARTESIAN_POINT('Ctrl Pts',(-2.359079411806,2.051668579855,0.2424553735028));
#13290=CARTESIAN_POINT('Ctrl Pts',(-2.075774396281,1.959946357633,-0.8343432069565));
#13291=CARTESIAN_POINT('Ctrl Pts',(-1.773180685345,1.914085246522,-1.260133922024));
#13292=CARTESIAN_POINT('Ctrl Pts',(-2.80488203134928,2.11666634473297,-0.494572811624998));
#13293=CARTESIAN_POINT('Ctrl Pts',(-2.80487937558295,2.14660584631654,-0.494558004365478));
#13294=CARTESIAN_POINT('Ctrl Pts',(-2.79983346453888,2.17665566318614,-0.493655688297967));
#13295=CARTESIAN_POINT('Ctrl Pts',(-2.7905135174355,2.2059245277796,-0.492002307694268));
#13296=CARTESIAN_POINT('Ctrl Pts',(-2.78143449325766,2.23443678502249,-0.490391667385945));
#13297=CARTESIAN_POINT('Ctrl Pts',(-2.76829948694453,2.26220798327608,-0.488068281113208));
#13298=CARTESIAN_POINT('Ctrl Pts',(-2.75185030367526,2.2883767040173,-0.485163523889622));
#13299=CARTESIAN_POINT('Ctrl Pts',(-2.73697041671003,2.31204885845072,-0.482535888313992));
#13300=CARTESIAN_POINT('Ctrl Pts',(-2.71937882394718,2.33440936083768,-0.479432564842254));
#13301=CARTESIAN_POINT('Ctrl Pts',(-2.69964797550406,2.35479239767097,-0.475954789776935));
#13302=CARTESIAN_POINT('Ctrl Pts',(-2.67769398815498,2.37747205759862,-0.472085162476968));
#13303=CARTESIAN_POINT('Ctrl Pts',(-2.65308669226524,2.39770433951941,-0.467748957240234));
#13304=CARTESIAN_POINT('Ctrl Pts',(-2.62668935647612,2.41451402502038,-0.463099122677085));
#13305=CARTESIAN_POINT('Ctrl Pts',(-2.59782850631059,2.43289246360406,-0.458015345295399));
#13306=CARTESIAN_POINT('Ctrl Pts',(-2.56682898609739,2.44717752991955,-0.452556858916761));
#13307=CARTESIAN_POINT('Ctrl Pts',(-2.53488055017212,2.45610210728703,-0.446934213906201));
#13308=CARTESIAN_POINT('Ctrl Pts',(-2.51095355439453,2.4627859501358,-0.442723272132987));
#13309=CARTESIAN_POINT('Ctrl Pts',(-2.4864958736503,2.46646307575719,-0.438420524025264));
#13310=CARTESIAN_POINT('Ctrl Pts',(-2.46201974870111,2.46661565567391,-0.434116553411453));
#13311=CARTESIAN_POINT('Ctrl Pts',(-2.4614874708036,2.46661897380198,-0.434022955734777));
#13312=CARTESIAN_POINT('Ctrl Pts',(-2.46095516857897,2.46662062601791,-0.433929353220448));
#13313=CARTESIAN_POINT('Ctrl Pts',(-2.46042284748648,2.46662060679558,-0.433835746825998));
#13314=CARTESIAN_POINT('Ctrl Pts',(-2.4341026224681,2.46661965636165,-0.429207447478404));
#13315=CARTESIAN_POINT('Ctrl Pts',(-2.4077358960525,2.46252740142272,-0.424569585932339));
#13316=CARTESIAN_POINT('Ctrl Pts',(-2.38198601504193,2.45495667506435,-0.420038577079773));
#13317=CARTESIAN_POINT('Ctrl Pts',(-2.35468695727497,2.44693047501666,-0.415234971488041));
#13318=CARTESIAN_POINT('Ctrl Pts',(-2.32808303963376,2.43499588080182,-0.410551788797338));
#13319=CARTESIAN_POINT('Ctrl Pts',(-2.30295408710686,2.41994167565776,-0.40612600330845));
#13320=CARTESIAN_POINT('Ctrl Pts',(-2.27843778078218,2.40525449343672,-0.401808118881841));
#13321=CARTESIAN_POINT('Ctrl Pts',(-2.2553269609863,2.38759986147607,-0.397735514989597));
#13322=CARTESIAN_POINT('Ctrl Pts',(-2.23431049879009,2.36773953428499,-0.39402922589206));
#13323=CARTESIAN_POINT('Ctrl Pts',(-2.23039092446436,2.3640355793647,-0.393338002247719));
#13324=CARTESIAN_POINT('Ctrl Pts',(-2.22654405866287,2.36025494368539,-0.392659495570005));
#13325=CARTESIAN_POINT('Ctrl Pts',(-2.22277416406729,2.35640260460539,-0.391994454672969));
#13326=CARTESIAN_POINT('Ctrl Pts',(-2.19954128922871,2.33266164596257,-0.387895981484488));
#13327=CARTESIAN_POINT('Ctrl Pts',(-2.17920592227961,2.306174071094,-0.384307040881674));
#13328=CARTESIAN_POINT('Ctrl Pts',(-2.16269258007162,2.27798421341354,-0.381390012556976));
#13329=CARTESIAN_POINT('Ctrl Pts',(-2.14410185480835,2.24624806377481,-0.378106021255483));
#13330=CARTESIAN_POINT('Ctrl Pts',(-2.13035431230019,2.21235423640297,-0.375673478333305));
#13331=CARTESIAN_POINT('Ctrl Pts',(-2.1227482802833,2.17772617536897,-0.374320245893729));
#13332=CARTESIAN_POINT('Ctrl Pts',(-2.11831275250703,2.15753250195116,-0.373531095905909));
#13333=CARTESIAN_POINT('Ctrl Pts',(-2.11596549328742,2.13708792799894,-0.373108934523806));
#13334=CARTESIAN_POINT('Ctrl Pts',(-2.11596363797559,2.11666691256093,-0.373098826465249));
#13335=CARTESIAN_POINT('Ctrl Pts',(-2.723241031212,2.083418579855,0.7501055518504));
#13336=CARTESIAN_POINT('Ctrl Pts',(-2.90336253938,2.037557468744,0.09617854059695));
#13337=CARTESIAN_POINT('Ctrl Pts',(-2.770829284715,1.945835246522,-1.343530217087));
#13338=CARTESIAN_POINT('Ctrl Pts',(-1.195947740385,1.808251913189,-2.838156522639));
#13339=CARTESIAN_POINT('Ctrl Pts',(0.9733915155363,1.670668579855,-2.921802275403));
#13340=CARTESIAN_POINT('Ctrl Pts',(2.659003940873,1.533085246522,-1.553807235173));
#13341=CARTESIAN_POINT('Ctrl Pts',(3.023382251462,1.395501913189,0.586319405716));
#13342=CARTESIAN_POINT('Ctrl Pts',(1.885450495222,1.257918579855,2.435092627868));
#13343=CARTESIAN_POINT('Ctrl Pts',(-0.1893529006074,1.120335246522,3.07388193938));
#13344=CARTESIAN_POINT('Ctrl Pts',(-2.1700678844,0.9827519131886,2.185270885497));
#13345=CARTESIAN_POINT('Ctrl Pts',(-3.072484926538,0.8451685798553,0.2108079169741));
#13346=CARTESIAN_POINT('Ctrl Pts',(-2.448196776368,0.7075852465219,-1.868404715163));
#13347=CARTESIAN_POINT('Ctrl Pts',(-0.6074096414087,0.5700019131886,-3.019214656103));
#13348=CARTESIAN_POINT('Ctrl Pts',(1.535196862268,0.4324185798553,-2.669789170172));
#13349=CARTESIAN_POINT('Ctrl Pts',(2.914970315305,0.2948352465219,-0.9937563478226));
#13350=CARTESIAN_POINT('Ctrl Pts',(2.846306923502,0.1572519131886,1.176069944827));
#13351=CARTESIAN_POINT('Ctrl Pts',(1.363325245947,0.01966857985526,2.761511885139));
#13352=CARTESIAN_POINT('Ctrl Pts',(-0.7970871784129,-0.1179147534781,2.974769847899));
#13353=CARTESIAN_POINT('Ctrl Pts',(-2.561430239181,-0.2554980868114,1.70987682241));
#13354=CARTESIAN_POINT('Ctrl Pts',(-3.053009075134,-0.3930814201447,-0.4046470129032));
#13355=CARTESIAN_POINT('Ctrl Pts',(-2.02756017042,-0.5306647534781,-2.318103400039));
#13356=CARTESIAN_POINT('Ctrl Pts',(0.005375102551742,-0.6682480868114,-3.079703675251));
#13357=CARTESIAN_POINT('Ctrl Pts',(2.035639508015,-0.8058314201447,-2.311011770959));
#13358=CARTESIAN_POINT('Ctrl Pts',(3.054402959379,-0.9434147534781,-0.3939875596977));
#13359=CARTESIAN_POINT('Ctrl Pts',(2.55544604064,-1.080998086811,1.718807474687));
#13360=CARTESIAN_POINT('Ctrl Pts',(0.7866984730786,-1.218581420145,2.977534043191));
#13361=CARTESIAN_POINT('Ctrl Pts',(-1.372956547484,-1.356164753478,2.756736298041));
#13362=CARTESIAN_POINT('Ctrl Pts',(-2.850394340374,-1.493748086811,1.166126828691));
#13363=CARTESIAN_POINT('Ctrl Pts',(-2.911485537975,-1.631331420145,-1.003923625649));
#13364=CARTESIAN_POINT('Ctrl Pts',(-1.525861343972,-1.768914753478,-2.67513850868));
#13365=CARTESIAN_POINT('Ctrl Pts',(0.6179193574188,-1.906498086811,-3.017050753102));
#13366=CARTESIAN_POINT('Ctrl Pts',(2.454799386092,-2.044081420145,-1.859941778329));
#13367=CARTESIAN_POINT('Ctrl Pts',(3.071373658657,-2.181664753478,0.2218833436086));
#13368=CARTESIAN_POINT('Ctrl Pts',(2.466296445201,-2.2733869757,1.534974329146));
#13369=CARTESIAN_POINT('Ctrl Pts',(1.983343137733,-2.319248086811,2.011230979028));
#13370=CARTESIAN_POINT('Ctrl Pts',(-2.738856610305,2.121330133205,0.7544067989448));
#13371=CARTESIAN_POINT('Ctrl Pts',(-2.920010969265,2.075469022094,0.09673004653804));
#13372=CARTESIAN_POINT('Ctrl Pts',(-2.786717743854,1.983746799872,-1.35123427344));
#13373=CARTESIAN_POINT('Ctrl Pts',(-1.202805530906,1.846163466539,-2.854431048893));
#13374=CARTESIAN_POINT('Ctrl Pts',(0.9789731265745,1.708580133205,-2.938556442222));
#13375=CARTESIAN_POINT('Ctrl Pts',(2.674251172341,1.570996799872,-1.562717059716));
#13376=CARTESIAN_POINT('Ctrl Pts',(3.040718897075,1.433413466539,0.5896814720732));
#13377=CARTESIAN_POINT('Ctrl Pts',(1.896262024938,1.295830133205,2.449055909521));
#13378=CARTESIAN_POINT('Ctrl Pts',(-0.19043868595,1.158246799872,3.091508159754));
#13379=CARTESIAN_POINT('Ctrl Pts',(-2.182511464053,1.020663466539,2.197801642033));
#13380=CARTESIAN_POINT('Ctrl Pts',(-3.090103136176,0.8830801332053,0.2120167294381));
#13381=CARTESIAN_POINT('Ctrl Pts',(-2.462235199687,0.745496799872,-1.879118501153));
#13382=CARTESIAN_POINT('Ctrl Pts',(-0.610892643166,0.6079134665387,-3.036527403935));
#13383=CARTESIAN_POINT('Ctrl Pts',(1.543999971413,0.4703301332053,-2.685098246184));
#13384=CARTESIAN_POINT('Ctrl Pts',(2.931685306373,0.332746799872,-0.9994547346604));
#13385=CARTESIAN_POINT('Ctrl Pts',(2.862628185696,0.1951634665387,1.18281375231));
#13386=CARTESIAN_POINT('Ctrl Pts',(1.37114281074,0.05758013320533,2.777346916547));
#13387=CARTESIAN_POINT('Ctrl Pts',(-0.8016578270393,-0.08000320012801,2.991827740796));
#13388=CARTESIAN_POINT('Ctrl Pts',(-2.57611796459,-0.2175865334613,1.719681579482));
#13389=CARTESIAN_POINT('Ctrl Pts',(-3.070515606557,-0.3551698667947,-0.4069673354021));
#13390=CARTESIAN_POINT('Ctrl Pts',(-2.03918658389,-0.492753200128,-2.331395843335));
#13391=CARTESIAN_POINT('Ctrl Pts',(0.005405924406315,-0.6303365334613,-3.097363278559));
#13392=CARTESIAN_POINT('Ctrl Pts',(2.047312249934,-0.7679198667947,-2.324263549512));
#13393=CARTESIAN_POINT('Ctrl Pts',(3.071917483598,-0.905503200128,-0.396246758876));
#13394=CARTESIAN_POINT('Ctrl Pts',(2.570099451523,-1.043086533461,1.728663441808));
#13395=CARTESIAN_POINT('Ctrl Pts',(0.7912095509038,-1.180669866795,2.994607786506));
#13396=CARTESIAN_POINT('Ctrl Pts',(-1.380829339981,-1.318253200128,2.772543945329));
#13397=CARTESIAN_POINT('Ctrl Pts',(-2.866739040589,-1.455836533461,1.172813620464));
#13398=CARTESIAN_POINT('Ctrl Pts',(-2.928180546671,-1.593419866795,-1.009680313581));
#13399=CARTESIAN_POINT('Ctrl Pts',(-1.53461092149,-1.731003200128,-2.690478258812));
#13400=CARTESIAN_POINT('Ctrl Pts',(0.6214626238752,-1.868586533461,-3.034351092706));
#13401=CARTESIAN_POINT('Ctrl Pts',(2.468875670024,-2.006169866795,-1.870607036239));
#13402=CARTESIAN_POINT('Ctrl Pts',(3.088985496074,-2.143753200128,0.2231556646635));
#13403=CARTESIAN_POINT('Ctrl Pts',(2.480438655444,-2.23547542235,1.543776162244));
#13404=CARTESIAN_POINT('Ctrl Pts',(1.994716002375,-2.281336533461,2.022763757826));
#13405=CARTESIAN_POINT('Ctrl Pts',(-2.786237260851,2.336331733269,0.7674576044437));
#13406=CARTESIAN_POINT('Ctrl Pts',(-2.970525486456,2.290470622158,0.09840342093635));
#13407=CARTESIAN_POINT('Ctrl Pts',(-2.834926364595,2.198748399936,-1.374609852386));
#13408=CARTESIAN_POINT('Ctrl Pts',(-1.223613377626,2.061165066603,-2.903811071025));
#13409=CARTESIAN_POINT('Ctrl Pts',(0.9959088009101,1.923581733269,-2.989391785472));
#13410=CARTESIAN_POINT('Ctrl Pts',(2.720514185816,1.785998399936,-1.589751169728));
#13411=CARTESIAN_POINT('Ctrl Pts',(3.093321592276,1.648415066603,0.5998826237716));
#13412=CARTESIAN_POINT('Ctrl Pts',(1.929066271794,1.510831733269,2.491423173941));
#13413=CARTESIAN_POINT('Ctrl Pts',(-0.193733166134,1.373248399936,3.144989480107));
#13414=CARTESIAN_POINT('Ctrl Pts',(-2.220267662242,1.235665066603,2.235822351543));
#13415=CARTESIAN_POINT('Ctrl Pts',(-3.143560150426,1.098081733269,0.2156844974145));
#13416=CARTESIAN_POINT('Ctrl Pts',(-2.504830458278,0.960498399936,-1.911626174867));
#13417=CARTESIAN_POINT('Ctrl Pts',(-0.6214607359745,0.8229150666027,-3.089057588706));
#13418=CARTESIAN_POINT('Ctrl Pts',(1.570710286518,0.6853317332693,-2.731548907824));
#13419=CARTESIAN_POINT('Ctrl Pts',(2.982401782909,0.547748399936,-1.016744729084));
#13420=CARTESIAN_POINT('Ctrl Pts',(2.9121500136,0.4101650666027,1.203275752711));
#13421=CARTESIAN_POINT('Ctrl Pts',(1.394862795977,0.2725817332693,2.825393427343));
#13422=CARTESIAN_POINT('Ctrl Pts',(-0.8155260482588,0.134998399936,3.043584646998));
#13423=CARTESIAN_POINT('Ctrl Pts',(-2.620683329782,-0.002584933397334,1.749431085776));
#13424=CARTESIAN_POINT('Ctrl Pts',(-3.123633767764,-0.1401682667307,-0.4140076371944));
#13425=CARTESIAN_POINT('Ctrl Pts',(-2.074463343749,-0.277751600064,-2.371727656005));
#13426=CARTESIAN_POINT('Ctrl Pts',(0.005499443802035,-0.4153349333973,-3.150945889114));
#13427=CARTESIAN_POINT('Ctrl Pts',(2.082729579161,-0.5529182667307,-2.364471977585));
#13428=CARTESIAN_POINT('Ctrl Pts',(3.125059896475,-0.690501600064,-0.4031016008351));
#13429=CARTESIAN_POINT('Ctrl Pts',(2.614560699886,-0.8280849333973,1.758568329176));
#13430=CARTESIAN_POINT('Ctrl Pts',(0.804897022931,-0.9656682667307,3.046412785907));
#13431=CARTESIAN_POINT('Ctrl Pts',(-1.404716896626,-1.103251600064,2.820507367475));
#13432=CARTESIAN_POINT('Ctrl Pts',(-2.916331983928,-1.240834933397,1.193102624313));
#13433=CARTESIAN_POINT('Ctrl Pts',(-2.978836392872,-1.378418266731,-1.027147204663));
#13434=CARTESIAN_POINT('Ctrl Pts',(-1.561158811409,-1.516001600064,-2.737021991588));
#13435=CARTESIAN_POINT('Ctrl Pts',(0.6322135712956,-1.653584933397,-3.086843628539));
#13436=CARTESIAN_POINT('Ctrl Pts',(2.511585804947,-1.791168266731,-1.902967466485));
#13437=CARTESIAN_POINT('Ctrl Pts',(3.142423175791,-1.928751600064,0.227016129839));
#13438=CARTESIAN_POINT('Ctrl Pts',(2.523348823392,-2.020473822286,1.570482605578));
#13439=CARTESIAN_POINT('Ctrl Pts',(2.029223446646,-2.066334933397,2.057756412201));
#13440=CARTESIAN_POINT('Ctrl Pts',(-2.410238510585,2.726333333333,0.663890293717));
#13441=CARTESIAN_POINT('Ctrl Pts',(-2.569657302604,2.680472222222,0.08512401942456));
#13442=CARTESIAN_POINT('Ctrl Pts',(-2.452357089121,2.58875,-1.18910821049));
#13443=CARTESIAN_POINT('Ctrl Pts',(-1.058488494954,2.451166666667,-2.511945902522));
#13444=CARTESIAN_POINT('Ctrl Pts',(0.8615123265745,2.313583333333,-2.585977621436));
#13445=CARTESIAN_POINT('Ctrl Pts',(2.353384670925,2.176,-1.375216513455));
#13446=CARTESIAN_POINT('Ctrl Pts',(2.675882248826,2.038416666667,0.5189293180307));
#13447=CARTESIAN_POINT('Ctrl Pts',(1.668741525741,1.900833333333,2.155209164837));
#13448=CARTESIAN_POINT('Ctrl Pts',(-0.1675891512739,1.76325,2.720577628778));
#13449=CARTESIAN_POINT('Ctrl Pts',(-1.92064570327,1.625666666667,1.934101309402));
#13450=CARTESIAN_POINT('Ctrl Pts',(-2.719341185102,1.488083333333,0.1865781816606));
#13451=CARTESIAN_POINT('Ctrl Pts',(-2.166807155247,1.3505,-1.653654945056));
#13452=CARTESIAN_POINT('Ctrl Pts',(-0.5375954947229,1.212916666667,-2.672193666465));
#13453=CARTESIAN_POINT('Ctrl Pts',(1.358745170317,1.075333333333,-2.362930272913));
#13454=CARTESIAN_POINT('Ctrl Pts',(2.579930909764,0.93775,-0.8795364759154));
#13455=CARTESIAN_POINT('Ctrl Pts',(2.519159516672,0.8001666666667,1.040895403556));
#13456=CARTESIAN_POINT('Ctrl Pts',(1.206628048187,0.6625833333333,2.444110608175));
#13457=CARTESIAN_POINT('Ctrl Pts',(-0.7054719694972,0.525,2.632857233479));
#13458=CARTESIAN_POINT('Ctrl Pts',(-2.267025846736,0.3874166666667,1.513347852245));
#13459=CARTESIAN_POINT('Ctrl Pts',(-2.702103839402,0.2498333333333,-0.3581378961739));
#13460=CARTESIAN_POINT('Ctrl Pts',(-1.794517469906,0.11225,-2.05166638658));
#13461=CARTESIAN_POINT('Ctrl Pts',(0.004757301693121,-0.02533333333332,
-2.725730228873));
#13462=CARTESIAN_POINT('Ctrl Pts',(1.801668188622,-0.1629166666667,-2.045389851629));
#13463=CARTESIAN_POINT('Ctrl Pts',(2.703337514074,-0.3005,-0.3487036138892));
#13464=CARTESIAN_POINT('Ctrl Pts',(2.261729457025,-0.4380833333333,1.521252037661));
#13465=CARTESIAN_POINT('Ctrl Pts',(0.6962773159997,-0.5756666666667,2.63530371907));
#13466=CARTESIAN_POINT('Ctrl Pts',(-1.215152351987,-0.71325,2.439883915127));
#13467=CARTESIAN_POINT('Ctrl Pts',(-2.52277713606,-0.8508333333333,1.032095124347));
#13468=CARTESIAN_POINT('Ctrl Pts',(-2.576846664034,-0.9884166666667,-0.8885351522298));
#13469=CARTESIAN_POINT('Ctrl Pts',(-1.350482653171,-1.126,-2.367664771818));
#13470=CARTESIAN_POINT('Ctrl Pts',(0.5468972502313,-1.263583333333,-2.670278477069));
#13471=CARTESIAN_POINT('Ctrl Pts',(2.172650877504,-1.401166666667,-1.64616471704));
#13472=CARTESIAN_POINT('Ctrl Pts',(2.718357643575,-1.53875,0.1963806264277));
#13473=CARTESIAN_POINT('Ctrl Pts',(2.182826493363,-1.630472222222,1.358548214596));
#13474=CARTESIAN_POINT('Ctrl Pts',(1.755382632488,-1.676333333333,1.780065114977));
#13475=CARTESIAN_POINT('Ctrl Pts',(-2.03423976032,2.336331733269,0.5603229829904));
#13476=CARTESIAN_POINT('Ctrl Pts',(-2.168789118751,2.290470622158,0.07184461791278));
#13477=CARTESIAN_POINT('Ctrl Pts',(-2.069787813647,2.198748399936,-1.003606568594));
#13478=CARTESIAN_POINT('Ctrl Pts',(-0.8933636122811,2.061165066603,-2.120080734019));
#13479=CARTESIAN_POINT('Ctrl Pts',(0.7271158522389,1.923581733269,-2.1825634574));
#13480=CARTESIAN_POINT('Ctrl Pts',(1.986255156035,1.785998399936,-1.160681857182));
#13481=CARTESIAN_POINT('Ctrl Pts',(2.258442905376,1.648415066603,0.4379760122899));
#13482=CARTESIAN_POINT('Ctrl Pts',(1.408416779688,1.510831733269,1.818995155733));
#13483=CARTESIAN_POINT('Ctrl Pts',(-0.1414451364138,1.373248399936,2.29616577745));
#13484=CARTESIAN_POINT('Ctrl Pts',(-1.621023744297,1.235665066603,1.632380267261));
#13485=CARTESIAN_POINT('Ctrl Pts',(-2.295122219778,1.098081733269,0.1574718659068));
#13486=CARTESIAN_POINT('Ctrl Pts',(-1.828783852216,0.960498399936,-1.395683715246));
#13487=CARTESIAN_POINT('Ctrl Pts',(-0.4537302534712,0.8229150666027,-2.255329744224));
#13488=CARTESIAN_POINT('Ctrl Pts',(1.146780054116,0.6853317332693,-1.994311638003));
#13489=CARTESIAN_POINT('Ctrl Pts',(2.177460036619,0.547748399936,-0.7423282227468));
#13490=CARTESIAN_POINT('Ctrl Pts',(2.126169019745,0.4101650666027,0.8785150544019));
#13491=CARTESIAN_POINT('Ctrl Pts',(1.018393300397,0.2725817332693,2.062827789006));
#13492=CARTESIAN_POINT('Ctrl Pts',(-0.5954178907355,0.134998399936,2.22212981996));
#13493=CARTESIAN_POINT('Ctrl Pts',(-1.913368363691,-0.002584933397335,1.277264618713));
#13494=CARTESIAN_POINT('Ctrl Pts',(-2.28057391104,-0.1401682667307,-0.3022681551533));
#13495=CARTESIAN_POINT('Ctrl Pts',(-1.514571596064,-0.277751600064,-1.731605117154));
#13496=CARTESIAN_POINT('Ctrl Pts',(0.004015159584192,-0.4153349333973,-2.300514568631));
#13497=CARTESIAN_POINT('Ctrl Pts',(1.520606798084,-0.5529182667307,-1.726307725673));
#13498=CARTESIAN_POINT('Ctrl Pts',(2.281615131673,-0.690501600064,-0.2943056269432));
#13499=CARTESIAN_POINT('Ctrl Pts',(1.908898214165,-0.8280849333973,1.283935746146));
#13500=CARTESIAN_POINT('Ctrl Pts',(0.5876576090685,-0.9656682667307,2.224194652233));
#13501=CARTESIAN_POINT('Ctrl Pts',(-1.025587807349,-1.103251600064,2.059260462779));
#13502=CARTESIAN_POINT('Ctrl Pts',(-2.129222288193,-1.240834933397,0.8710876243819));
#13503=CARTESIAN_POINT('Ctrl Pts',(-2.174856935197,-1.378418266731,-0.7499230997967));
#13504=CARTESIAN_POINT('Ctrl Pts',(-1.139806494933,-1.516001600064,-1.998307552049));
#13505=CARTESIAN_POINT('Ctrl Pts',(0.4615809291669,-1.653584933397,-2.2537133256));
#13506=CARTESIAN_POINT('Ctrl Pts',(1.833715950062,-1.791168266731,-1.389361967594));
#13507=CARTESIAN_POINT('Ctrl Pts',(2.294292111359,-1.928751600064,0.1657451230163));
#13508=CARTESIAN_POINT('Ctrl Pts',(1.842304163333,-2.020473822286,1.146613823613));
#13509=CARTESIAN_POINT('Ctrl Pts',(1.48154181833,-2.066334933397,1.502373817754));
#13510=CARTESIAN_POINT('Ctrl Pts',(-2.081620410866,2.121330133205,0.5733737884892));
#13511=CARTESIAN_POINT('Ctrl Pts',(-2.219303635942,2.075469022094,0.07351799231108));
#13512=CARTESIAN_POINT('Ctrl Pts',(-2.117996434389,1.983746799872,-1.02698214754));
#13513=CARTESIAN_POINT('Ctrl Pts',(-0.9141714590009,1.846163466539,-2.169460756152));
#13514=CARTESIAN_POINT('Ctrl Pts',(0.7440515265746,1.708580133205,-2.233398800651));
#13515=CARTESIAN_POINT('Ctrl Pts',(2.03251816951,1.570996799872,-1.187715967194));
#13516=CARTESIAN_POINT('Ctrl Pts',(2.311045600577,1.433413466539,0.4481771639882));
#13517=CARTESIAN_POINT('Ctrl Pts',(1.441221026544,1.295830133205,1.861362420153));
#13518=CARTESIAN_POINT('Ctrl Pts',(-0.1447396165978,1.158246799872,2.349647097803));
#13519=CARTESIAN_POINT('Ctrl Pts',(-1.658779942486,1.020663466539,1.670400976771));
#13520=CARTESIAN_POINT('Ctrl Pts',(-2.348579234028,0.8830801332053,0.1611396338832));
#13521=CARTESIAN_POINT('Ctrl Pts',(-1.871379110807,0.745496799872,-1.42819138896));
#13522=CARTESIAN_POINT('Ctrl Pts',(-0.4642983462798,0.6079134665387,-2.307859928994));
#13523=CARTESIAN_POINT('Ctrl Pts',(1.17349036922,0.4703301332053,-2.040762299642));
#13524=CARTESIAN_POINT('Ctrl Pts',(2.228176513155,0.332746799872,-0.7596182171705));
#13525=CARTESIAN_POINT('Ctrl Pts',(2.175690847649,0.1951634665387,0.8989770548032));
#13526=CARTESIAN_POINT('Ctrl Pts',(1.042113285635,0.05758013320533,2.110874299803));
#13527=CARTESIAN_POINT('Ctrl Pts',(-0.6092861119551,-0.08000320012801,2.273886726162));
#13528=CARTESIAN_POINT('Ctrl Pts',(-1.957933728882,-0.2175865334613,1.307014125008));
#13529=CARTESIAN_POINT('Ctrl Pts',(-2.333692072247,-0.3551698667947,-0.3093084569456));
#13530=CARTESIAN_POINT('Ctrl Pts',(-1.549848355923,-0.492753200128,-1.771936929824));
#13531=CARTESIAN_POINT('Ctrl Pts',(0.004108678979917,-0.6303365334613,-2.354097179186));
#13532=CARTESIAN_POINT('Ctrl Pts',(1.556024127311,-0.7679198667947,-1.766516153745));
#13533=CARTESIAN_POINT('Ctrl Pts',(2.33475754455,-0.905503200128,-0.3011604689023));
#13534=CARTESIAN_POINT('Ctrl Pts',(1.953359462527,-1.043086533461,1.313840633513));
#13535=CARTESIAN_POINT('Ctrl Pts',(0.6013450810956,-1.180669866795,2.275999651633));
#13536=CARTESIAN_POINT('Ctrl Pts',(-1.049475363994,-1.318253200128,2.107223884925));
#13537=CARTESIAN_POINT('Ctrl Pts',(-2.178815231532,-1.455836533461,0.8913766282303));
#13538=CARTESIAN_POINT('Ctrl Pts',(-2.225512781398,-1.593419866795,-0.7673899908785));
#13539=CARTESIAN_POINT('Ctrl Pts',(-1.166354384852,-1.731003200128,-2.044851284825));
#13540=CARTESIAN_POINT('Ctrl Pts',(0.4723318765873,-1.868586533461,-2.306205861433));
#13541=CARTESIAN_POINT('Ctrl Pts',(1.876426084985,-2.006169866795,-1.42172239784));
#13542=CARTESIAN_POINT('Ctrl Pts',(2.347729791075,-2.143753200128,0.1696055881918));
#13543=CARTESIAN_POINT('Ctrl Pts',(1.885214331281,-2.23547542235,1.173320266948));
#13544=CARTESIAN_POINT('Ctrl Pts',(1.516049262601,-2.281336533461,1.537366472129));
#13545=CARTESIAN_POINT('Ctrl Pts',(-2.097235989958,2.083418579855,0.5776750355837));
#13546=CARTESIAN_POINT('Ctrl Pts',(-2.235952065827,2.037557468744,0.07406949825217));
#13547=CARTESIAN_POINT('Ctrl Pts',(-2.133884893527,1.945835246522,-1.034686203893));
#13548=CARTESIAN_POINT('Ctrl Pts',(-0.9210292495221,1.808251913189,-2.185735282405));
#13549=CARTESIAN_POINT('Ctrl Pts',(0.7496331376127,1.670668579855,-2.25015296747));
#13550=CARTESIAN_POINT('Ctrl Pts',(2.047765400978,1.533085246522,-1.196625791736));
#13551=CARTESIAN_POINT('Ctrl Pts',(2.328382246189,1.395501913189,0.4515392303455));
#13552=CARTESIAN_POINT('Ctrl Pts',(1.452032556261,1.257918579855,1.875325701807));
#13553=CARTESIAN_POINT('Ctrl Pts',(-0.1458254019403,1.120335246522,2.367273318177));
#13554=CARTESIAN_POINT('Ctrl Pts',(-1.671223522139,0.9827519131886,1.682931733308));
#13555=CARTESIAN_POINT('Ctrl Pts',(-2.366197443666,0.8451685798553,0.1623484463472));
#13556=CARTESIAN_POINT('Ctrl Pts',(-1.885417534126,0.7075852465219,-1.43890517495));
#13557=CARTESIAN_POINT('Ctrl Pts',(-0.4677813480371,0.5700019131886,-2.325172676827));
#13558=CARTESIAN_POINT('Ctrl Pts',(1.182293478365,0.4324185798553,-2.056071375655));
#13559=CARTESIAN_POINT('Ctrl Pts',(2.244891504223,0.2948352465219,-0.7653166040083));
#13560=CARTESIAN_POINT('Ctrl Pts',(2.192012109843,0.1572519131886,0.9057208622855));
#13561=CARTESIAN_POINT('Ctrl Pts',(1.049930850427,0.01966857985526,2.12670933121));
#13562=CARTESIAN_POINT('Ctrl Pts',(-0.6138567605814,-0.1179147534781,2.290944619059));
#13563=CARTESIAN_POINT('Ctrl Pts',(-1.972621454292,-0.2554980868114,1.31681888208));
#13564=CARTESIAN_POINT('Ctrl Pts',(-2.35119860367,-0.3930814201447,-0.3116287794445));
#13565=CARTESIAN_POINT('Ctrl Pts',(-1.561474769393,-0.5306647534781,-1.785229373121));
#13566=CARTESIAN_POINT('Ctrl Pts',(0.004139500834489,-0.6682480868114,-2.371756782494));
#13567=CARTESIAN_POINT('Ctrl Pts',(1.56769686923,-0.8058314201447,-1.779767932299));
#13568=CARTESIAN_POINT('Ctrl Pts',(2.352272068769,-0.9434147534781,-0.3034196680806));
#13569=CARTESIAN_POINT('Ctrl Pts',(1.968012873411,-1.080998086811,1.323696600635));
#13570=CARTESIAN_POINT('Ctrl Pts',(0.6058561589209,-1.218581420145,2.293073394949));
#13571=CARTESIAN_POINT('Ctrl Pts',(-1.057348156491,-1.356164753478,2.123031532212));
#13572=CARTESIAN_POINT('Ctrl Pts',(-2.195159931747,-1.493748086811,0.8980634200042));
#13573=CARTESIAN_POINT('Ctrl Pts',(-2.242207790093,-1.631331420145,-0.7731466788102));
#13574=CARTESIAN_POINT('Ctrl Pts',(-1.175103962369,-1.768914753478,-2.060191034956));
#13575=CARTESIAN_POINT('Ctrl Pts',(0.4758751430437,-1.906498086811,-2.323506201036));
#13576=CARTESIAN_POINT('Ctrl Pts',(1.890502368917,-2.044081420145,-1.43238765575));
#13577=CARTESIAN_POINT('Ctrl Pts',(2.365341628493,-2.181664753478,0.1708779092467));
#13578=CARTESIAN_POINT('Ctrl Pts',(1.899356541525,-2.2733869757,1.182122100046));
#13579=CARTESIAN_POINT('Ctrl Pts',(1.527422127243,-2.319248086811,1.548899250927));
#13580=CARTESIAN_POINT('',(2.01902946446485,-2.11666642077307,0.73486384668651));
#13581=CARTESIAN_POINT('Ctrl Pts',(-2.1159627305594,2.11666642077307,-0.373103972679151));
#13582=CARTESIAN_POINT('Ctrl Pts',(-2.09791744924042,2.10732932202772,-0.476586603307615));
#13583=CARTESIAN_POINT('Ctrl Pts',(-2.07240856203006,2.09799224087489,-0.578864236800211));
#13584=CARTESIAN_POINT('Ctrl Pts',(-2.03952544136795,2.0886551715116,-0.678701259971635));
#13585=CARTESIAN_POINT('Ctrl Pts',(-2.01029652232723,2.08035570239182,-0.767443697087925));
#13586=CARTESIAN_POINT('Ctrl Pts',(-1.97524204365226,2.07205624258692,-0.854257078451053));
#13587=CARTESIAN_POINT('Ctrl Pts',(-1.93445881079141,2.06375678802135,-0.93827986748618));
#13588=CARTESIAN_POINT('Ctrl Pts',(-1.89504922115652,2.05573687209811,-1.01947263724898));
#13589=CARTESIAN_POINT('Ctrl Pts',(-1.8502908018872,2.04771696106718,-1.09805921260102));
#13590=CARTESIAN_POINT('Ctrl Pts',(-1.80075999246287,2.0396970512512,-1.17349099183197));
#13591=CARTESIAN_POINT('Ctrl Pts',(-1.74049142569068,2.02993850953002,-1.26527558562648));
#13592=CARTESIAN_POINT('Ctrl Pts',(-1.67317186324321,2.02017988192998,-1.35238096779209));
#13593=CARTESIAN_POINT('Ctrl Pts',(-1.59973693945821,2.01042122840127,-1.43398501440707));
#13594=CARTESIAN_POINT('Ctrl Pts',(-1.52530346600026,2.00052987914978,-1.51669869237808));
#13595=CARTESIAN_POINT('Ctrl Pts',(-1.44458628575752,1.99063850325969,-1.59376141933641));
#13596=CARTESIAN_POINT('Ctrl Pts',(-1.3585161844784,1.9807471631603,-1.66428745788304));
#13597=CARTESIAN_POINT('Ctrl Pts',(-1.3062486076442,1.97474047360196,-1.70711563031186));
#13598=CARTESIAN_POINT('Ctrl Pts',(-1.25200622931957,1.96873379724231,-1.74753260324364));
#13599=CARTESIAN_POINT('Ctrl Pts',(-1.19599201792712,1.96272714806199,-1.78533235701608));
#13600=CARTESIAN_POINT('Ctrl Pts',(-1.11297034403313,1.95382437040884,-1.84135740410602));
#13601=CARTESIAN_POINT('Ctrl Pts',(-1.02600255192884,1.94492160418517,-1.89166253407849));
#13602=CARTESIAN_POINT('Ctrl Pts',(-0.935879106074206,1.93601884024483,
-1.93547516733291));
#13603=CARTESIAN_POINT('Ctrl Pts',(-0.902630932934798,1.9327344492176,-1.95163844207593));
#13604=CARTESIAN_POINT('Ctrl Pts',(-0.868953602670152,1.92945005850113,
-1.96691847080026));
#13605=CARTESIAN_POINT('Ctrl Pts',(-0.834887819739237,1.92616566763619,
-1.98127795335741));
#13606=CARTESIAN_POINT('Ctrl Pts',(-0.742544771603072,1.91726257962103,
-2.02020259488623));
#13607=CARTESIAN_POINT('Ctrl Pts',(-0.647346424999575,1.90835949051486,
-2.05235929784953));
#13608=CARTESIAN_POINT('Ctrl Pts',(-0.550392479691278,1.89945639117047,
-2.07769736257899));
#13609=CARTESIAN_POINT('Ctrl Pts',(-0.500666710376223,1.89489016683808,
-2.09069275701725));
#13610=CARTESIAN_POINT('Ctrl Pts',(-0.450479375516837,1.89032393981257,
-2.1018953643128));
#13611=CARTESIAN_POINT('Ctrl Pts',(-0.399979430919417,1.88575770885988,
-2.11130361223012));
#13612=CARTESIAN_POINT('Ctrl Pts',(-0.28761302935216,1.87559748106223,-2.13223771368211));
#13613=CARTESIAN_POINT('Ctrl Pts',(-0.173596384538557,1.86543719671815,
-2.14431302429515));
#13614=CARTESIAN_POINT('Ctrl Pts',(-0.059331666635636,1.85527690565331,
-2.14749845845954));
#13615=CARTESIAN_POINT('Ctrl Pts',(0.0534748849115257,1.84524627311182,
-2.15064324234261));
#13616=CARTESIAN_POINT('Ctrl Pts',(0.166524593003937,1.83521563402004,-2.14512354089506));
#13617=CARTESIAN_POINT('Ctrl Pts',(0.278468664955484,1.82518503632032,-2.13085995349825));
#13618=CARTESIAN_POINT('Ctrl Pts',(0.339467829366259,1.81971928840212,-2.12308761774579));
#13619=CARTESIAN_POINT('Ctrl Pts',(0.400138589926789,1.81425355277422,-2.11271815102493));
#13620=CARTESIAN_POINT('Ctrl Pts',(0.460260570476484,1.80878783719352,-2.09973246983707));
#13621=CARTESIAN_POINT('Ctrl Pts',(0.534366335791568,1.80205084961594,-2.08372644618706));
#13622=CARTESIAN_POINT('Ctrl Pts',(0.607612372580839,1.79531386845014,-2.06374965831702));
#13623=CARTESIAN_POINT('Ctrl Pts',(0.679535519150437,1.78857688481004,-2.03978711598877));
#13624=CARTESIAN_POINT('Ctrl Pts',(0.784586812609899,1.77873681413512,-2.00478731152772));
#13625=CARTESIAN_POINT('Ctrl Pts',(0.886814383123217,1.7688967381816,-1.96128244214364));
#13626=CARTESIAN_POINT('Ctrl Pts',(0.985092375620573,1.75905662926039,-1.9101743840555));
#13627=CARTESIAN_POINT('Ctrl Pts',(1.07577295070114,1.74997721368467,-1.86301725374671));
#13628=CARTESIAN_POINT('Ctrl Pts',(1.16309051312948,1.74089777004143,-1.80938813864657));
#13629=CARTESIAN_POINT('Ctrl Pts',(1.24618512059533,1.73181827657948,-1.75002634145707));
#13630=CARTESIAN_POINT('Ctrl Pts',(1.36358913358838,1.71898989937323,-1.66615431388427));
#13631=CARTESIAN_POINT('Ctrl Pts',(1.47281388914806,1.70616159057245,-1.57067191622397));
#13632=CARTESIAN_POINT('Ctrl Pts',(1.57156518045832,1.69333330644984,-1.46538680864991));
#13633=CARTESIAN_POINT('Ctrl Pts',(1.66312630474595,1.68143906080139,-1.36776760091787));
#13634=CARTESIAN_POINT('Ctrl Pts',(1.7456841370641,1.66954483636822,-1.26172009680776));
#13635=CARTESIAN_POINT('Ctrl Pts',(1.81736534288417,1.65765059829595,-1.14866906455378));
#13636=CARTESIAN_POINT('Ctrl Pts',(1.82299436771583,1.65671656041675,-1.13979132511674));
#13637=CARTESIAN_POINT('Ctrl Pts',(1.82855629251586,1.65578252245344,-1.1308703926222));
#13638=CARTESIAN_POINT('Ctrl Pts',(1.83405019594872,1.65484848438915,-1.12190695532944));
#13639=CARTESIAN_POINT('Ctrl Pts',(1.84159744189999,1.65356535025961,-1.10959343969452));
#13640=CARTESIAN_POINT('Ctrl Pts',(1.84901495135613,1.65228221661491,-1.09720193972246));
#13641=CARTESIAN_POINT('Ctrl Pts',(1.85630043380627,1.65099908337441,-1.08473439120323));
#13642=CARTESIAN_POINT('Ctrl Pts',(1.94269536698868,1.63578304087669,-0.936887899410816));
#13643=CARTESIAN_POINT('Ctrl Pts',(2.01052212471306,1.62056705521867,-0.778350603268342));
#13644=CARTESIAN_POINT('Ctrl Pts',(2.05902851263356,1.60535099192654,-0.614115400509273));
#13645=CARTESIAN_POINT('Ctrl Pts',(2.08822076975288,1.59619361593938,-0.515274887485631));
#13646=CARTESIAN_POINT('Ctrl Pts',(2.11041582715717,1.58703621183384,-0.41436987553872));
#13647=CARTESIAN_POINT('Ctrl Pts',(2.12545410071187,1.57787875029803,-0.312480553990116));
#13648=CARTESIAN_POINT('Ctrl Pts',(2.14392857232465,1.56662883769515,-0.187309843951518));
#13649=CARTESIAN_POINT('Ctrl Pts',(2.1516346752806,1.55537901727325,-0.0604049918487018));
#13650=CARTESIAN_POINT('Ctrl Pts',(2.14816648894054,1.54412923482214,0.066174082986945));
#13651=CARTESIAN_POINT('Ctrl Pts',(2.14501081737324,1.53389315892013,0.181347245068504));
#13652=CARTESIAN_POINT('Ctrl Pts',(2.1326043268812,1.52365711445421,0.29624939231303));
#13653=CARTESIAN_POINT('Ctrl Pts',(2.11067724421865,1.51342106058787,0.409318422375977));
#13654=CARTESIAN_POINT('Ctrl Pts',(2.101743119398,1.50925041078825,0.455388063443951));
#13655=CARTESIAN_POINT('Ctrl Pts',(2.09122886378167,1.50507975942804,0.501153357089501));
#13656=CARTESIAN_POINT('Ctrl Pts',(2.07918943147896,1.50090910374499,0.546522634163261));
#13657=CARTESIAN_POINT('Ctrl Pts',(2.04903054684587,1.4904615742912,0.66017307537594));
#13658=CARTESIAN_POINT('Ctrl Pts',(2.00933880556038,1.48001401010943,0.771215375000161));
#13659=CARTESIAN_POINT('Ctrl Pts',(1.96098677543066,1.46956642993763,0.878354690721158));
#13660=CARTESIAN_POINT('Ctrl Pts',(1.91103606510354,1.45877341774391,0.989036391362615));
#13661=CARTESIAN_POINT('Ctrl Pts',(1.85184243190155,1.44798038848529,1.09555405084697));
#13662=CARTESIAN_POINT('Ctrl Pts',(1.78431417030651,1.43718736282047,1.19646961655335));
#13663=CARTESIAN_POINT('Ctrl Pts',(1.75668454824819,1.43277132703128,1.2377598685813));
#13664=CARTESIAN_POINT('Ctrl Pts',(1.72765906814075,1.42835529184374,1.27811204753106));
#13665=CARTESIAN_POINT('Ctrl Pts',(1.69729778749964,1.42393925867288,1.31742636891535));
#13666=CARTESIAN_POINT('Ctrl Pts',(1.63448216537924,1.41480275767311,1.3987652816308));
#13667=CARTESIAN_POINT('Ctrl Pts',(1.5658689249794,1.40566628773615,1.47575704033619));
#13668=CARTESIAN_POINT('Ctrl Pts',(1.49205385466478,1.39652983581773,1.54738069358613));
#13669=CARTESIAN_POINT('Ctrl Pts',(1.43633087498025,1.38963273035582,1.60144937303014));
#13670=CARTESIAN_POINT('Ctrl Pts',(1.3776446213347,1.3827356351622,1.65245912261462));
#13671=CARTESIAN_POINT('Ctrl Pts',(1.31626715210567,1.37583854462525,1.69998258358999));
#13672=CARTESIAN_POINT('Ctrl Pts',(1.23514282231084,1.36672246580394,1.76279568047367));
#13673=CARTESIAN_POINT('Ctrl Pts',(1.14931667202321,1.35760639511763,1.81951639687443));
#13674=CARTESIAN_POINT('Ctrl Pts',(1.05990936844222,1.34849031960903,1.869797824271));
#13675=CARTESIAN_POINT('Ctrl Pts',(1.05493841437683,1.34798347519258,1.87259341988702));
#13676=CARTESIAN_POINT('Ctrl Pts',(1.04995639555256,1.34747663076123,1.87536912224497));
#13677=CARTESIAN_POINT('Ctrl Pts',(1.04496350631085,1.34696978631274,1.87812487607801));
#13678=CARTESIAN_POINT('Ctrl Pts',(0.948041444385353,1.33713091213688,1.93161962245169));
#13679=CARTESIAN_POINT('Ctrl Pts',(0.847013429065949,1.32729195529011,1.97760765487141));
#13680=CARTESIAN_POINT('Ctrl Pts',(0.743106714900058,1.31745297843196,2.01575585739578));
#13681=CARTESIAN_POINT('Ctrl Pts',(0.638611050831489,1.30755823362359,2.05412028637235));
#13682=CARTESIAN_POINT('Ctrl Pts',(0.531202666028629,1.29766346857635,2.08455620521816));
#13683=CARTESIAN_POINT('Ctrl Pts',(0.422107829237246,1.2877687470214,2.10667806381857));
#13684=CARTESIAN_POINT('Ctrl Pts',(0.356803767358516,1.28184577644184,2.11992018659361));
#13685=CARTESIAN_POINT('Ctrl Pts',(0.290895084545275,1.27592282144646,2.13018228339791));
#13686=CARTESIAN_POINT('Ctrl Pts',(0.224644020099001,1.26999989570497,2.13737269833159));
#13687=CARTESIAN_POINT('Ctrl Pts',(0.123910472701584,1.26099419404722,2.14830559442287));
#13688=CARTESIAN_POINT('Ctrl Pts',(0.0223534651988909,1.25198849831628,
2.15213498225265));
#13689=CARTESIAN_POINT('Ctrl Pts',(-0.0789421896134073,1.24298279799778,
2.14852091627407));
#13690=CARTESIAN_POINT('Ctrl Pts',(-0.0967017060199631,1.24140388641607,
2.14788728530382));
#13691=CARTESIAN_POINT('Ctrl Pts',(-0.114453167950561,1.23982497469336,
2.14702498251185));
#13692=CARTESIAN_POINT('Ctrl Pts',(-0.132190712177884,1.23824606277296,
2.14593234183677));
#13693=CARTESIAN_POINT('Ctrl Pts',(-0.233511303782116,1.22922698505763,
2.13969094797804));
#13694=CARTESIAN_POINT('Ctrl Pts',(-0.334376984468477,1.22020790089213,
2.12592952298826));
#13695=CARTESIAN_POINT('Ctrl Pts',(-0.433744204604765,1.21118879971508,
2.10510452173353));
#13696=CARTESIAN_POINT('Ctrl Pts',(-0.500430189366313,1.20513602252326,
2.09112872856524));
#13697=CARTESIAN_POINT('Ctrl Pts',(-0.566441361409203,1.19908323766973,
2.07397276038877));
#13698=CARTESIAN_POINT('Ctrl Pts',(-0.631466910669559,1.19303044196224,
2.05378688774323));
#13699=CARTESIAN_POINT('Ctrl Pts',(-0.744235133770776,1.18253359842165,
2.01878026317985));
#13700=CARTESIAN_POINT('Ctrl Pts',(-0.854181326126747,1.17203672388374,
1.9746243355874));
#13701=CARTESIAN_POINT('Ctrl Pts',(-0.959890726345071,1.16153985212526,
1.92196464448792));
#13702=CARTESIAN_POINT('Ctrl Pts',(-1.06326499824549,1.15127485702525,1.87046820978422));
#13703=CARTESIAN_POINT('Ctrl Pts',(-1.16258876159359,1.14100986458324,1.81083883984471));
#13704=CARTESIAN_POINT('Ctrl Pts',(-1.25651370446884,1.13074490638656,1.7436387469327));
#13705=CARTESIAN_POINT('Ctrl Pts',(-1.30130124395243,1.12585012331342,1.71159479010437));
#13706=CARTESIAN_POINT('Ctrl Pts',(-1.34486071727869,1.12095534802699,1.67782885244961));
#13707=CARTESIAN_POINT('Ctrl Pts',(-1.38704268345722,1.11606058395213,1.64239916098616));
#13708=CARTESIAN_POINT('Ctrl Pts',(-1.43127877616563,1.110927460558,1.60524415712565));
#13709=CARTESIAN_POINT('Ctrl Pts',(-1.47398011128263,1.10579434261416,1.5662754013788));
#13710=CARTESIAN_POINT('Ctrl Pts',(-1.51496355146127,1.10066122536907,1.52557708359342));
#13711=CARTESIAN_POINT('Ctrl Pts',(-1.59936798859271,1.09008969038048,1.44175984936666));
#13712=CARTESIAN_POINT('Ctrl Pts',(-1.67648317419432,1.07951815835558,1.3506049926823));
#13713=CARTESIAN_POINT('Ctrl Pts',(-1.74557465267766,1.06894658778899,1.25371561483115));
#13714=CARTESIAN_POINT('Ctrl Pts',(-1.81061573468134,1.0589947615548,1.16250624851802));
#13715=CARTESIAN_POINT('Ctrl Pts',(-1.86854620040408,1.04904290116538,1.06621628618952));
#13716=CARTESIAN_POINT('Ctrl Pts',(-1.91879263515764,1.03909097199534,0.966198552429217));
#13717=CARTESIAN_POINT('Ctrl Pts',(-1.99132854275518,1.02472433646716,0.821812644658154));
#13718=CARTESIAN_POINT('Ctrl Pts',(-2.04803940956963,1.01035782592291,0.669303181233791));
#13719=CARTESIAN_POINT('Ctrl Pts',(-2.08711562508526,0.995991341057153,
0.512433188410289));
#13720=CARTESIAN_POINT('Ctrl Pts',(-2.11695159290074,0.985022060270358,
0.392657821340147));
#13721=CARTESIAN_POINT('Ctrl Pts',(-2.13650618310517,0.974052794453662,
0.27034060601716));
#13722=CARTESIAN_POINT('Ctrl Pts',(-2.14495718917906,0.96308349940367,0.147168803041655));
#13723=CARTESIAN_POINT('Ctrl Pts',(-2.14520431216876,0.962762737004021,
0.143567032562207));
#13724=CARTESIAN_POINT('Ctrl Pts',(-2.14544193953318,0.962441974579376,
0.139964532269499));
#13725=CARTESIAN_POINT('Ctrl Pts',(-2.14567008358036,0.962121212128629,
0.13636134679483));
#13726=CARTESIAN_POINT('Ctrl Pts',(-2.15516426399469,0.948772730697037,
-0.0135846780317181));
#13727=CARTESIAN_POINT('Ctrl Pts',(-2.14822099037921,0.935424286247537,
-0.164423349917931));
#13728=CARTESIAN_POINT('Ctrl Pts',(-2.12589474834246,0.922075809850497,
-0.312966252775792));
#13729=CARTESIAN_POINT('Ctrl Pts',(-2.10530864227326,0.90976773084108,-0.449931531080373));
#13730=CARTESIAN_POINT('Ctrl Pts',(-2.07164326047299,0.897459624670079,
-0.584946205874195));
#13731=CARTESIAN_POINT('Ctrl Pts',(-2.02569043015659,0.885151437301664,
-0.715528591157759));
#13732=CARTESIAN_POINT('Ctrl Pts',(-1.98749536130351,0.874921119370076,
-0.824066044945969));
#13733=CARTESIAN_POINT('Ctrl Pts',(-1.94073977799007,0.864690870679638,
-0.929727460777095));
#13734=CARTESIAN_POINT('Ctrl Pts',(-1.8858438432095,0.854460656230511,-1.03096115210299));
#13735=CARTESIAN_POINT('Ctrl Pts',(-1.83405290034749,0.844809077217991,
-1.126468922289));
#13736=CARTESIAN_POINT('Ctrl Pts',(-1.77501716663259,0.83515752868288,-1.21803465117041));
#13737=CARTESIAN_POINT('Ctrl Pts',(-1.70913035983726,0.825505981234695,
-1.30436705469545));
#13738=CARTESIAN_POINT('Ctrl Pts',(-1.6697089960266,0.819731271823253,-1.35602141849824));
#13739=CARTESIAN_POINT('Ctrl Pts',(-1.62783580702056,0.813956562800911,
-1.40580264114003));
#13740=CARTESIAN_POINT('Ctrl Pts',(-1.58375469431755,0.808181847872517,
-1.45355564552886));
#13741=CARTESIAN_POINT('Ctrl Pts',(-1.50663754512336,0.798079345340714,
-1.53709653953341));
#13742=CARTESIAN_POINT('Ctrl Pts',(-1.42282440888977,0.787976785588606,
-1.61437197301895));
#13743=CARTESIAN_POINT('Ctrl Pts',(-1.33353038165379,0.777874206994567,
-1.68469145621377));
#13744=CARTESIAN_POINT('Ctrl Pts',(-1.24208559852269,0.767528295434824,
-1.75670467019557));
#13745=CARTESIAN_POINT('Ctrl Pts',(-1.14489166109636,0.757182364114533,
-1.82142370215485));
#13746=CARTESIAN_POINT('Ctrl Pts',(-1.04321319294084,0.746836454252634,
-1.87807141801992));
#13747=CARTESIAN_POINT('Ctrl Pts',(-0.99202792284582,0.741628289729049,
-1.90658806160648));
#13748=CARTESIAN_POINT('Ctrl Pts',(-0.939705677254979,0.73642013064334,
-1.93305867581673));
#13749=CARTESIAN_POINT('Ctrl Pts',(-0.886405385013102,0.731211982253794,
-1.95737972730217));
#13750=CARTESIAN_POINT('Ctrl Pts',(-0.794655020321894,0.722246749719266,
-1.99924563928135));
#13751=CARTESIAN_POINT('Ctrl Pts',(-0.699914968864438,0.713281537187404,
-2.0347782125959));
#13752=CARTESIAN_POINT('Ctrl Pts',(-0.603126898273636,0.70431633524596,
-2.06336312897213));
#13753=CARTESIAN_POINT('Ctrl Pts',(-0.544120557004141,0.698850746748558,
-2.08078977381131));
#13754=CARTESIAN_POINT('Ctrl Pts',(-0.484353672977853,0.693385162187266,
-2.09563499587624));
#13755=CARTESIAN_POINT('Ctrl Pts',(-0.424043634817683,0.687919579429389,
-2.10776825003111));
#13756=CARTESIAN_POINT('Ctrl Pts',(-0.325219461550571,0.678963662405497,
-2.12764982940785));
#13757=CARTESIAN_POINT('Ctrl Pts',(-0.224937133287094,0.670007750223784,
-2.14024694311598));
#13758=CARTESIAN_POINT('Ctrl Pts',(-0.124301651299459,0.661051833501158,
-2.14573522960947));
#13759=CARTESIAN_POINT('Ctrl Pts',(-0.0987968483685675,0.6587820685379,
-2.14712616710666));
#13760=CARTESIAN_POINT('Ctrl Pts',(-0.0732693595882916,0.656512303282978,
-2.14806076265642));
#13761=CARTESIAN_POINT('Ctrl Pts',(-0.0477371270765782,0.65424253758365,
-2.14854240201057));
#13762=CARTESIAN_POINT('Ctrl Pts',(0.0636113333177027,0.644343876510439,
-2.15064287640213));
#13763=CARTESIAN_POINT('Ctrl Pts',(0.17510225252277,0.634445137226091,-2.14413424933341));
#13764=CARTESIAN_POINT('Ctrl Pts',(0.285465785627553,0.624546381844607,
-2.12925879840794));
#13765=CARTESIAN_POINT('Ctrl Pts',(0.395624804477018,0.614665969810136,
-2.11441091312561));
#13766=CARTESIAN_POINT('Ctrl Pts',(0.50466196196004,0.604785541738159,-2.09122694606622));
#13767=CARTESIAN_POINT('Ctrl Pts',(0.611310018100132,0.594905159398069,
-2.05989728951752));
#13768=CARTESIAN_POINT('Ctrl Pts',(0.674751543483836,0.589027635233859,
-2.04126027658795));
#13769=CARTESIAN_POINT('Ctrl Pts',(0.737347461353159,0.583150127252695,
-2.01973981883648));
#13770=CARTESIAN_POINT('Ctrl Pts',(0.798827280241264,0.577272648457316,
-1.99536799962312));
#13771=CARTESIAN_POINT('Ctrl Pts',(0.892778217051504,0.568290926505382,
-1.95812398543641));
#13772=CARTESIAN_POINT('Ctrl Pts',(0.984119740890388,0.559309210317195,
-1.9142168626982));
#13773=CARTESIAN_POINT('Ctrl Pts',(1.07174864050312,0.550327485872927,-1.86382801026776));
#13774=CARTESIAN_POINT('Ctrl Pts',(1.16191422281691,0.541085758334656,-1.81198050058097));
#13775=CARTESIAN_POINT('Ctrl Pts',(1.24814793734788,0.531844022055364,-1.75327086036017));
#13776=CARTESIAN_POINT('Ctrl Pts',(1.3296681927492,0.522602261762046,-1.68863020361191));
#13777=CARTESIAN_POINT('Ctrl Pts',(1.39523376777737,0.515169246189157,-1.63664064826724));
#13778=CARTESIAN_POINT('Ctrl Pts',(1.45775066054175,0.507736215082205,-1.58081561857954));
#13779=CARTESIAN_POINT('Ctrl Pts',(1.51683029451761,0.500303160495069,-1.52165601801066));
#13780=CARTESIAN_POINT('Ctrl Pts',(1.6046859462726,0.489249675371074,-1.43368145019824));
#13781=CARTESIAN_POINT('Ctrl Pts',(1.68508261411045,0.478196192393638,-1.338202241932));
#13782=CARTESIAN_POINT('Ctrl Pts',(1.75685157244071,0.467142721989082,-1.23663042913025));
#13783=CARTESIAN_POINT('Ctrl Pts',(1.82625242210846,0.456453974991759,-1.13841010832946));
#13784=CARTESIAN_POINT('Ctrl Pts',(1.88758618313705,0.445765239751282,-1.03449142167311));
#13785=CARTESIAN_POINT('Ctrl Pts',(1.93975294714389,0.435076525695469,-0.926130709139889));
#13786=CARTESIAN_POINT('Ctrl Pts',(1.95885737315287,0.431162122517544,-0.886447028269824));
#13787=CARTESIAN_POINT('Ctrl Pts',(1.97673188425863,0.42724772218082,-0.846167484490858));
#13788=CARTESIAN_POINT('Ctrl Pts',(1.99332068309008,0.423333325148358,-0.805353531339599));
#13789=CARTESIAN_POINT('Ctrl Pts',(2.00827610756237,0.419804349375709,-0.768558221445805));
#13790=CARTESIAN_POINT('Ctrl Pts',(2.0221803966365,0.416275377002179,-0.731343412060049));
#13791=CARTESIAN_POINT('Ctrl Pts',(2.03499339342307,0.412746406294115,-0.693759244140605));
#13792=CARTESIAN_POINT('Ctrl Pts',(2.07801870352698,0.400896324569193,-0.567553758674014));
#13793=CARTESIAN_POINT('Ctrl Pts',(2.10873496467875,0.38904626162368,-0.437183446883494));
#13794=CARTESIAN_POINT('Ctrl Pts',(2.12723591878782,0.377196151815658,-0.305089849806085));
#13795=CARTESIAN_POINT('Ctrl Pts',(2.14328155922495,0.366918703420348,-0.190526765639993));
#13796=CARTESIAN_POINT('Ctrl Pts',(2.1501398316329,0.35664121977568,-0.0746682717553836));
#13797=CARTESIAN_POINT('Ctrl Pts',(2.14790281915223,0.346363658059301,0.0409003818768428));
#13798=CARTESIAN_POINT('Ctrl Pts',(2.14479530958078,0.332086750048781,0.201440700907735));
#13799=CARTESIAN_POINT('Ctrl Pts',(2.12413003425264,0.317809987717386,0.361830411071172));
#13800=CARTESIAN_POINT('Ctrl Pts',(2.0859467663204,0.303533255949083,0.517891861201881));
#13801=CARTESIAN_POINT('Ctrl Pts',(2.06065926664616,0.294078254596637,0.62124613345392));
#13802=CARTESIAN_POINT('Ctrl Pts',(2.02768927911112,0.284623266649076,0.72270102301507));
#13803=CARTESIAN_POINT('Ctrl Pts',(1.98705824020302,0.275168258668891,0.82103565699802));
#13804=CARTESIAN_POINT('Ctrl Pts',(1.97878691214473,0.273243486994341,0.841053801722414));
#13805=CARTESIAN_POINT('Ctrl Pts',(1.97019812461692,0.271318714489611,0.860942626125018));
#13806=CARTESIAN_POINT('Ctrl Pts',(1.96129871595332,0.269393940872609,0.880694548915241));
#13807=CARTESIAN_POINT('Ctrl Pts',(1.90856578436955,0.257988806071383,0.99773342559981));
#13808=CARTESIAN_POINT('Ctrl Pts',(1.84501274575367,0.246583674668671,1.10978491333392));
#13809=CARTESIAN_POINT('Ctrl Pts',(1.77210366778145,0.235178527568502,1.21539096611084));
#13810=CARTESIAN_POINT('Ctrl Pts',(1.69551977918379,0.223198530848588,1.32631984363946));
#13811=CARTESIAN_POINT('Ctrl Pts',(1.60861231781684,0.211218516808914,1.43013841101961));
#13812=CARTESIAN_POINT('Ctrl Pts',(1.51302369362006,0.199238463318028,1.52514280501988));
#13813=CARTESIAN_POINT('Ctrl Pts',(1.494899900635,0.196967021383977,1.54315582679942));
#13814=CARTESIAN_POINT('Ctrl Pts',(1.47646389638305,0.194695578031699,1.56085191741852));
#13815=CARTESIAN_POINT('Ctrl Pts',(1.45772670097547,0.192424133110347,1.57821935062689));
#13816=CARTESIAN_POINT('Ctrl Pts',(1.37836677344921,0.182803605575825,1.6517777573549));
#13817=CARTESIAN_POINT('Ctrl Pts',(1.29348115512078,0.173183129264224,1.71954821041346));
#13818=CARTESIAN_POINT('Ctrl Pts',(1.20397049377609,0.163562681136566,1.7805144196128));
#13819=CARTESIAN_POINT('Ctrl Pts',(1.12341823457021,0.154905066282492,1.83537901129886));
#13820=CARTESIAN_POINT('Ctrl Pts',(1.03912148844003,0.14624747425328,1.8847329446552));
#13821=CARTESIAN_POINT('Ctrl Pts',(0.951761962758758,0.137589888258096,
1.92786129340198));
#13822=CARTESIAN_POINT('Ctrl Pts',(0.877309773645605,0.130211457288489,
1.96461744508656));
#13823=CARTESIAN_POINT('Ctrl Pts',(0.800633647658955,0.122833030701572,
1.9968521186444));
#13824=CARTESIAN_POINT('Ctrl Pts',(0.722342758034967,0.115454598103574,
2.02450263203523));
#13825=CARTESIAN_POINT('Ctrl Pts',(0.617134365294067,0.105539357156503,
2.06165977875155));
#13826=CARTESIAN_POINT('Ctrl Pts',(0.509052265328476,0.0956240427058641,
2.09053133521612));
#13827=CARTESIAN_POINT('Ctrl Pts',(0.399404995198041,0.0857087073856261,
2.11104089390714));
#13828=CARTESIAN_POINT('Ctrl Pts',(0.287985874873716,0.0756331447401773,
2.1318818777718));
#13829=CARTESIAN_POINT('Ctrl Pts',(0.174949242882979,0.0655575605451831,
2.14408869178551));
#13830=CARTESIAN_POINT('Ctrl Pts',(0.0616511258305347,0.0554820100277887,
2.14753105216021));
#13831=CARTESIAN_POINT('Ctrl Pts',(-0.00205973434369371,0.0498162319293323,
2.14946679254326));
#13832=CARTESIAN_POINT('Ctrl Pts',(-0.0658534701497418,0.0441504644802167,
2.14863016618283));
#13833=CARTESIAN_POINT('Ctrl Pts',(-0.12948877016016,0.0384847175007255,
2.14499074027714));
#13834=CARTESIAN_POINT('Ctrl Pts',(-0.229535572857717,0.0295770849430313,
2.13926887009724));
#13835=CARTESIAN_POINT('Ctrl Pts',(-0.32926218534485,0.0206694642280899,
2.12660962764732));
#13836=CARTESIAN_POINT('Ctrl Pts',(-0.427570331839619,0.0117618471326195,
2.10688913349251));
#13837=CARTESIAN_POINT('Ctrl Pts',(-0.470839874821073,0.00784123084071015,
2.09820931600158));
#13838=CARTESIAN_POINT('Ctrl Pts',(-0.513834571500548,0.00392061524998314,
2.08816222949006));
#13839=CARTESIAN_POINT('Ctrl Pts',(-0.556460950674994,-3.40744243931823E-10,
2.07674052552866));
#13840=CARTESIAN_POINT('Ctrl Pts',(-0.653307832806579,-0.00890761584438663,
2.05079048147811));
#13841=CARTESIAN_POINT('Ctrl Pts',(-0.748251944292738,-0.0178152313480485,
2.01774148912384));
#13842=CARTESIAN_POINT('Ctrl Pts',(-0.840392897999384,-0.0267228550750663,
1.97822993810398));
#13843=CARTESIAN_POINT('Ctrl Pts',(-0.880947998121618,-0.0306434740568333,
1.96083924652619));
#13844=CARTESIAN_POINT('Ctrl Pts',(-0.920960336094546,-0.0345640946316652,
1.94219722621708));
#13845=CARTESIAN_POINT('Ctrl Pts',(-0.960354805675053,-0.0384847175007351,
1.92236085704252));
#13846=CARTESIAN_POINT('Ctrl Pts',(-1.06141534381935,-0.0485424809692676,
1.871473659805));
#13847=CARTESIAN_POINT('Ctrl Pts',(-1.1584932522127,-0.0586003089435517,
1.8126904579763));
#13848=CARTESIAN_POINT('Ctrl Pts',(-1.25050001533805,-0.0686581464875737,
1.74682307061668));
#13849=CARTESIAN_POINT('Ctrl Pts',(-1.34161250164382,-0.0786182250118753,
1.68159589355988));
#13850=CARTESIAN_POINT('Ctrl Pts',(-1.42775300990498,-0.0885783129207585,
1.60942070905301));
#13851=CARTESIAN_POINT('Ctrl Pts',(-1.50783543107933,-0.0985383568645636,
1.53104539645999));
#13852=CARTESIAN_POINT('Ctrl Pts',(-1.55317317335856,-0.104177121262445,
1.48667411408254));
#13853=CARTESIAN_POINT('Ctrl Pts',(-1.59656860554779,-0.109815871568963,
1.4403149458517));
#13854=CARTESIAN_POINT('Ctrl Pts',(-1.6378184947156,-0.115454598103576,
1.39209933035345));
#13855=CARTESIAN_POINT('Ctrl Pts',(-1.69179513731939,-0.122833030701568,
1.32900783851737));
#13856=CARTESIAN_POINT('Ctrl Pts',(-1.74208127350863,-0.130211457288479,
1.26275372934031));
#13857=CARTESIAN_POINT('Ctrl Pts',(-1.78818068480565,-0.13758988825808,
1.1936958736796));
#13858=CARTESIAN_POINT('Ctrl Pts',(-1.84828770736962,-0.147210304317604,
1.10365433146394));
#13859=CARTESIAN_POINT('Ctrl Pts',(-1.90127508606266,-0.156830727827904,
1.00884599998052));
#13860=CARTESIAN_POINT('Ctrl Pts',(-1.94682567081003,-0.166451181827962,
0.910589167921595));
#13861=CARTESIAN_POINT('Ctrl Pts',(-1.98781746390209,-0.175108801966302,
0.822166071884982));
#13862=CARTESIAN_POINT('Ctrl Pts',(-2.02278698960568,-0.183766446796818,
0.730951298313189));
#13863=CARTESIAN_POINT('Ctrl Pts',(-2.05153803013303,-0.192424133110348,
0.637914699899324));
#13864=CARTESIAN_POINT('Ctrl Pts',(-2.09139068444731,-0.20442480416385,
0.508953962230096));
#13865=CARTESIAN_POINT('Ctrl Pts',(-2.11937975563295,-0.216425431419754,
0.376252287616784));
#13866=CARTESIAN_POINT('Ctrl Pts',(-2.13494174468323,-0.228426037123835,
0.242118082797647));
#13867=CARTESIAN_POINT('Ctrl Pts',(-2.1497621600032,-0.2398547793014,0.114375760295607));
#13868=CARTESIAN_POINT('Ctrl Pts',(-2.1533115885628,-0.251283501932252,
-0.0146671125818596));
#13869=CARTESIAN_POINT('Ctrl Pts',(-2.14505715479067,-0.26271222423113,
-0.14300745196953));
#13870=CARTESIAN_POINT('Ctrl Pts',(-2.14344852391613,-0.264939463076827,
-0.168018523363072));
#13871=CARTESIAN_POINT('Ctrl Pts',(-2.14139145421298,-0.267166701909915,
-0.193002851471323));
#13872=CARTESIAN_POINT('Ctrl Pts',(-2.13888178688306,-0.269393940872609,
-0.217945505641568));
#13873=CARTESIAN_POINT('Ctrl Pts',(-2.13671293946929,-0.271318714489607,
-0.239500876883247));
#13874=CARTESIAN_POINT('Ctrl Pts',(-2.13420663545479,-0.273243486994335,
-0.261019497831176));
#13875=CARTESIAN_POINT('Ctrl Pts',(-2.13136074331412,-0.275168258668881,
-0.28249138372823));
#13876=CARTESIAN_POINT('Ctrl Pts',(-2.1102517111346,-0.289445000445393,
-0.441756284838774));
#13877=CARTESIAN_POINT('Ctrl Pts',(-2.07045749324644,-0.303721696547568,
-0.598446701518509));
#13878=CARTESIAN_POINT('Ctrl Pts',(-2.01401963788178,-0.317998462091363,
-0.748892742727702));
#13879=CARTESIAN_POINT('Ctrl Pts',(-1.97664273626235,-0.327453485811278,
-0.848528117689688));
#13880=CARTESIAN_POINT('Ctrl Pts',(-1.93196655588015,-0.336908539988082,
-0.945425405945982));
#13881=CARTESIAN_POINT('Ctrl Pts',(-1.88058859718454,-0.346363658059302,
-1.03853063984612));
#13882=CARTESIAN_POINT('Ctrl Pts',(-1.81619583542424,-0.358213898528815,
-1.15522081784032));
#13883=CARTESIAN_POINT('Ctrl Pts',(-1.74113749645292,-0.370064035205387,
-1.26619866219996));
#13884=CARTESIAN_POINT('Ctrl Pts',(-1.65650994003969,-0.381914133730994,
-1.369289610165));
#13885=CARTESIAN_POINT('Ctrl Pts',(-1.58311354473584,-0.392191572341276,
-1.45869906838148));
#13886=CARTESIAN_POINT('Ctrl Pts',(-1.50252055125346,-0.402468982254876,
-1.54217545295685));
#13887=CARTESIAN_POINT('Ctrl Pts',(-1.41547635316767,-0.412746406294107,
-1.61830982624727));
#13888=CARTESIAN_POINT('Ctrl Pts',(-1.38558788849214,-0.416275377002174,
-1.64445217205234));
#13889=CARTESIAN_POINT('Ctrl Pts',(-1.35493901623949,-0.419804349375706,
-1.66972899784035));
#13890=CARTESIAN_POINT('Ctrl Pts',(-1.32358958377519,-0.423333325148358,
-1.69411695871237));
#13891=CARTESIAN_POINT('Ctrl Pts',(-1.22901514748013,-0.433979479421723,
-1.76769014554705));
#13892=CARTESIAN_POINT('Ctrl Pts',(-1.12818410298468,-0.444625658136703,
-1.83308698183334));
#13893=CARTESIAN_POINT('Ctrl Pts',(-1.02267279851515,-0.455271851977543,
-1.88978810786402));
#13894=CARTESIAN_POINT('Ctrl Pts',(-0.913233663837565,-0.466314367728904,
-1.94860002568875));
#13895=CARTESIAN_POINT('Ctrl Pts',(-0.798758150774989,-0.477356899753293,
-1.99805751311023));
#13896=CARTESIAN_POINT('Ctrl Pts',(-0.680967747542164,-0.48839943765537,
-2.03754066959344));
#13897=CARTESIAN_POINT('Ctrl Pts',(-0.638642208663121,-0.492367344670458,
-2.05172812314595));
#13898=CARTESIAN_POINT('Ctrl Pts',(-0.595888406433419,-0.496335252444458,
-2.06462729201675));
#13899=CARTESIAN_POINT('Ctrl Pts',(-0.552785559276754,-0.500303160495067,
-2.07620791467739));
#13900=CARTESIAN_POINT('Ctrl Pts',(-0.452393043337931,-0.50954496929639,
-2.10318079284514));
#13901=CARTESIAN_POINT('Ctrl Pts',(-0.349975592528666,-0.518786741799876,
-2.12303119653041));
#13902=CARTESIAN_POINT('Ctrl Pts',(-0.24666352700019,-0.528028493278499,
-2.13530341028129));
#13903=CARTESIAN_POINT('Ctrl Pts',(-0.163571110884956,-0.535461501761749,
-2.14517377621025));
#13904=CARTESIAN_POINT('Ctrl Pts',(-0.0799008481762825,-0.542894496644514,
-2.15014272792901));
#13905=CARTESIAN_POINT('Ctrl Pts',(0.00375245598683078,-0.550327485872929,
-2.14999672542845));
#13906=CARTESIAN_POINT('Ctrl Pts',(0.104835735372361,-0.559309210317197,
-2.14982030189441));
#13907=CARTESIAN_POINT('Ctrl Pts',(0.205893376806318,-0.568290926505382,
-2.14217422367334));
#13908=CARTESIAN_POINT('Ctrl Pts',(0.305879281886703,-0.577272648457315,
-2.12745301769284));
#13909=CARTESIAN_POINT('Ctrl Pts',(0.415433915962271,-0.587113928195907,
-2.11132298083365));
#13910=CARTESIAN_POINT('Ctrl Pts',(0.523701381992398,-0.596955289760699,
-2.08670807798976));
#13911=CARTESIAN_POINT('Ctrl Pts',(0.629506698707356,-0.606796672111442,
-2.05410204499644));
#13912=CARTESIAN_POINT('Ctrl Pts',(0.7362266343023,-0.616723126879929,-2.02121415382905));
#13913=CARTESIAN_POINT('Ctrl Pts',(0.840442973658776,-0.626649602795276,
-1.98019595821689));
#13914=CARTESIAN_POINT('Ctrl Pts',(0.940939887621261,-0.636576037220439,
-1.93150309431318));
#13915=CARTESIAN_POINT('Ctrl Pts',(1.00055963316546,-0.642464889636447,
-1.90261607638105));
#13916=CARTESIAN_POINT('Ctrl Pts',(1.0588700592828,-0.648353727450196,-1.87102705996308));
#13917=CARTESIAN_POINT('Ctrl Pts',(1.11561276575759,-0.654242537583649,
-1.83682373771093));
#13918=CARTESIAN_POINT('Ctrl Pts',(1.20190916640318,-0.663198457210571,
-1.7848060638308));
#13919=CARTESIAN_POINT('Ctrl Pts',(1.28461395722914,-0.672154369918574,
-1.72671438540263));
#13920=CARTESIAN_POINT('Ctrl Pts',(1.36267612235558,-0.681110285090713,
-1.66293744887761));
#13921=CARTESIAN_POINT('Ctrl Pts',(1.38246000075157,-0.683380049661083,
-1.64677398281648));
#13922=CARTESIAN_POINT('Ctrl Pts',(1.40194579851717,-0.685649814389728,
-1.63024558168205));
#13923=CARTESIAN_POINT('Ctrl Pts',(1.42111668508107,-0.687919579429389,
-1.61335903240838));
#13924=CARTESIAN_POINT('Ctrl Pts',(1.49683848269127,-0.696884771956248,
-1.54665998527912));
#13925=CARTESIAN_POINT('Ctrl Pts',(1.56764415040306,-0.705849969335355,
-1.47437066573726));
#13926=CARTESIAN_POINT('Ctrl Pts',(1.63299881687974,-0.714815180979017,
-1.39747640935412));
#13927=CARTESIAN_POINT('Ctrl Pts',(1.67284194765184,-0.7202807753914,-1.35059822791942));
#13928=CARTESIAN_POINT('Ctrl Pts',(1.71065986859473,-0.725746375105432,
-1.30200929725504));
#13929=CARTESIAN_POINT('Ctrl Pts',(1.74633944512399,-0.731211982253794,
-1.25193787618981));
#13930=CARTESIAN_POINT('Ctrl Pts',(1.81383563057361,-0.741551444477461,
-1.1572161824171));
#13931=CARTESIAN_POINT('Ctrl Pts',(1.87376027274665,-0.751890948856925,
-1.05708688572005));
#13932=CARTESIAN_POINT('Ctrl Pts',(1.92543098634018,-0.762230454249894,
-0.952865578606035));
#13933=CARTESIAN_POINT('Ctrl Pts',(1.97615540761795,-0.772380602968229,
-0.850552970157105));
#13934=CARTESIAN_POINT('Ctrl Pts',(2.01892596431358,-0.782530752663265,
-0.744295584274527));
#13935=CARTESIAN_POINT('Ctrl Pts',(2.05305207438863,-0.792680864412052,
-0.635318870181491));
#13936=CARTESIAN_POINT('Ctrl Pts',(2.07042427884942,-0.797847870443853,
-0.57984328991393));
#13937=CARTESIAN_POINT('Ctrl Pts',(2.08555557901215,-0.803014866642226,
-0.523662827821059));
#13938=CARTESIAN_POINT('Ctrl Pts',(2.09834962140627,-0.808181847872517,
-0.466938767683641));
#13939=CARTESIAN_POINT('Ctrl Pts',(2.11264848263973,-0.81395656280091,-0.403542896424378));
#13940=CARTESIAN_POINT('Ctrl Pts',(2.12402111673552,-0.81973127182325,-0.339494498482121));
#13941=CARTESIAN_POINT('Ctrl Pts',(2.13233383734598,-0.825505981234692,
-0.275049825307238));
#13942=CARTESIAN_POINT('Ctrl Pts',(2.14706022967544,-0.835736162226755,
-0.160882925541307));
#13943=CARTESIAN_POINT('Ctrl Pts',(2.15218037387138,-0.845966344439981,
-0.0454727405449347));
#13944=CARTESIAN_POINT('Ctrl Pts',(2.14805857657556,-0.856196562874184,
0.0696147130120628));
#13945=CARTESIAN_POINT('Ctrl Pts',(2.14416991397958,-0.8658481456471,0.178192656999639));
#13946=CARTESIAN_POINT('Ctrl Pts',(2.1320559120424,-0.875499760659425,0.286482292885839));
#13947=CARTESIAN_POINT('Ctrl Pts',(2.11206366829738,-0.885151437301663,
0.393179278001693));
#13948=CARTESIAN_POINT('Ctrl Pts',(2.08441372175388,-0.898500031217214,
0.5407448025337));
#13949=CARTESIAN_POINT('Ctrl Pts',(2.04164123141159,-0.911848529627996,
0.685599334388376));
#13950=CARTESIAN_POINT('Ctrl Pts',(1.98445313399436,-0.925197001463674,
0.824494840372859));
#13951=CARTESIAN_POINT('Ctrl Pts',(1.93172235030964,-0.937505076267311,
0.952564652302691));
#13952=CARTESIAN_POINT('Ctrl Pts',(1.866734999188,-0.949813128477027,1.0755686879077));
#13953=CARTESIAN_POINT('Ctrl Pts',(1.79002412712317,-0.962121212128629,
1.19092743220905));
#13954=CARTESIAN_POINT('Ctrl Pts',(1.78802495584534,-0.962441974579362,
1.19393381034094));
#13955=CARTESIAN_POINT('Ctrl Pts',(1.78601791436486,-0.962762737003993,
1.19693485342922));
#13956=CARTESIAN_POINT('Ctrl Pts',(1.78400301433828,-0.963083499403627,
1.19993051666803));
#13957=CARTESIAN_POINT('Ctrl Pts',(1.69375843327332,-0.977450002949473,
1.33410212341423));
#13958=CARTESIAN_POINT('Ctrl Pts',(1.58775427402266,-0.991816456350905,
1.45748085014487));
#13959=CARTESIAN_POINT('Ctrl Pts',(1.46947880964235,-1.0061829589133,1.56770856745458));
#13960=CARTESIAN_POINT('Ctrl Pts',(1.37917162655664,-1.01715225321286,1.65187103259783));
#13961=CARTESIAN_POINT('Ctrl Pts',(1.28170911994277,-1.0281215761724,1.72836702686252));
#13962=CARTESIAN_POINT('Ctrl Pts',(1.17862389042603,-1.03909097199534,1.79614880908248));
#13963=CARTESIAN_POINT('Ctrl Pts',(1.07927620822019,-1.04966265190832,1.86147303633505));
#13964=CARTESIAN_POINT('Ctrl Pts',(0.974522219696174,-1.0602342542074,1.91881853880723));
#13965=CARTESIAN_POINT('Ctrl Pts',(0.865769157978579,-1.070805820398,1.96712566934777));
#13966=CARTESIAN_POINT('Ctrl Pts',(0.763391600568948,-1.0807576425122,2.0126008582951));
#13967=CARTESIAN_POINT('Ctrl Pts',(0.657471367298694,-1.09070943262743,
2.05006596767214));
#13968=CARTESIAN_POINT('Ctrl Pts',(0.549208379576276,-1.10066122536905,
2.07867028555393));
#13969=CARTESIAN_POINT('Ctrl Pts',(0.493366520354362,-1.10579434261414,
2.09342434255806));
#13970=CARTESIAN_POINT('Ctrl Pts',(0.436901701494061,-1.11092746055799,
2.10582160743021));
#13971=CARTESIAN_POINT('Ctrl Pts',(0.380014619514122,-1.11606058395213,
2.11588073829693));
#13972=CARTESIAN_POINT('Ctrl Pts',(0.266781811981912,-1.12627798222775,
2.13590327398919));
#13973=CARTESIAN_POINT('Ctrl Pts',(0.151977035804607,-1.13649542935549,
2.14664964747342));
#13974=CARTESIAN_POINT('Ctrl Pts',(0.0370366125123074,-1.14671289418464,
2.14832797671703));
#13975=CARTESIAN_POINT('Ctrl Pts',(-0.0810644601923213,-1.15721132043087,
2.15005245691595));
#13976=CARTESIAN_POINT('Ctrl Pts',(-0.199310124060812,-1.16770976536543,
2.14220340823848));
#13977=CARTESIAN_POINT('Ctrl Pts',(-0.316153836373017,-1.17820819519649,
2.12495366561866));
#13978=CARTESIAN_POINT('Ctrl Pts',(-0.371142628313499,-1.18314894863763,
2.11683562067489));
#13979=CARTESIAN_POINT('Ctrl Pts',(-0.425820945600476,-1.18808969873363,
2.10663473889586));
#13980=CARTESIAN_POINT('Ctrl Pts',(-0.480027057582445,-1.19303044196224,
2.09436507407996));
#13981=CARTESIAN_POINT('Ctrl Pts',(-0.578978142735444,-1.20204957072943,
2.07196729265631));
#13982=CARTESIAN_POINT('Ctrl Pts',(-0.676460590337036,-1.2110686753973,
2.04264685296404));
#13983=CARTESIAN_POINT('Ctrl Pts',(-0.771335842863926,-1.2200877665272,
2.00649586702304));
#13984=CARTESIAN_POINT('Ctrl Pts',(-0.83500723907403,-1.22614053697568,
1.98223470631011));
#13985=CARTESIAN_POINT('Ctrl Pts',(-0.897504289009474,-1.23219330132686,
1.95489826292322));
#13986=CARTESIAN_POINT('Ctrl Pts',(-0.958485656028116,-1.23824606277299,
1.92452727892239));
#13987=CARTESIAN_POINT('Ctrl Pts',(-1.04921780185708,-1.2472517650235,1.87933930292163));
#13988=CARTESIAN_POINT('Ctrl Pts',(-1.13659283713798,-1.25625746084299,
1.82743191255314));
#13989=CARTESIAN_POINT('Ctrl Pts',(-1.21983547650336,-1.2652631607459,1.76963483802778));
#13990=CARTESIAN_POINT('Ctrl Pts',(-1.23442987368726,-1.26684207225452,
1.75950164825724));
#13991=CARTESIAN_POINT('Ctrl Pts',(-1.24889732962621,-1.26842098388866,
1.74918751959763));
#13992=CARTESIAN_POINT('Ctrl Pts',(-1.2632337773796,-1.26999989570497,1.73869704406139));
#13993=CARTESIAN_POINT('Ctrl Pts',(-1.35279273421466,-1.27986326616023,
1.67316365239487));
#13994=CARTESIAN_POINT('Ctrl Pts',(-1.43727166003755,-1.28972671774178,
1.60073036213476));
#13995=CARTESIAN_POINT('Ctrl Pts',(-1.51582812240706,-1.29959018732102,
1.52236007107001));
#13996=CARTESIAN_POINT('Ctrl Pts',(-1.59447737559033,-1.30946530762054,
1.44389720909685));
#13997=CARTESIAN_POINT('Ctrl Pts',(-1.66719110375498,-1.31934044596026,
1.35948231302115));
#13998=CARTESIAN_POINT('Ctrl Pts',(-1.73309015729065,-1.32921553898753,
1.27004330919134));
#13999=CARTESIAN_POINT('Ctrl Pts',(-1.7725831932114,-1.33513364224883,1.21644287638613));
#14000=CARTESIAN_POINT('Ctrl Pts',(-1.8096279889798,-1.34105172923591,1.16103734046149));
#14001=CARTESIAN_POINT('Ctrl Pts',(-1.84402738053199,-1.34696978631274,
1.10402210100787));
#14002=CARTESIAN_POINT('Ctrl Pts',(-1.89701562762061,-1.35608586239785,
1.01619678027794));
#14003=CARTESIAN_POINT('Ctrl Pts',(-1.94372842826759,-1.36520193294027,
0.924538465851365));
#14004=CARTESIAN_POINT('Ctrl Pts',(-1.983366316552,-1.37431801089728,0.82990628909204));
#14005=CARTESIAN_POINT('Ctrl Pts',(-1.98557014234611,-1.37482485544961,
0.824644837457733));
#14006=CARTESIAN_POINT('Ctrl Pts',(-1.98775210914776,-1.37533170002485,
0.819374200175097));
#14007=CARTESIAN_POINT('Ctrl Pts',(-1.98991208368564,-1.37583854462525,
0.814094527327367));
#14008=CARTESIAN_POINT('Ctrl Pts',(-2.02884800367239,-1.38497497677321,
0.71892260934876));
#14009=CARTESIAN_POINT('Ctrl Pts',(-2.06063345853673,-1.39411141709258,
0.620813452405457));
#14010=CARTESIAN_POINT('Ctrl Pts',(-2.08522380920602,-1.40324787862765,
0.520945067607857));
#14011=CARTESIAN_POINT('Ctrl Pts',(-2.10378705929605,-1.4101449913486,0.445554446790037));
#14012=CARTESIAN_POINT('Ctrl Pts',(-2.11825105895416,-1.4170421161598,0.369161879812258));
#14013=CARTESIAN_POINT('Ctrl Pts',(-2.12861618621955,-1.42393925867289,
0.292275809346556));
#14014=CARTESIAN_POINT('Ctrl Pts',(-2.14484500772538,-1.43473820902624,
0.171894237376967));
#14015=CARTESIAN_POINT('Ctrl Pts',(-2.15105642268712,-1.4455371714393,0.0501320965044703));
#14016=CARTESIAN_POINT('Ctrl Pts',(-2.14720407173045,-1.45633612521925,
-0.0713091123552385));
#14017=CARTESIAN_POINT('Ctrl Pts',(-2.14346081128115,-1.46682927525492,
-0.189311360632586));
#14018=CARTESIAN_POINT('Ctrl Pts',(-2.13021549798078,-1.47732241713949,
-0.307011950828631));
#14019=CARTESIAN_POINT('Ctrl Pts',(-2.10737820057378,-1.48781553188887,
-0.422842016555831));
#14020=CARTESIAN_POINT('Ctrl Pts',(-2.09787920513487,-1.49218006099089,
-0.47102062746686));
#14021=CARTESIAN_POINT('Ctrl Pts',(-2.08672015986324,-1.49654458539831,
-0.518875413538272));
#14022=CARTESIAN_POINT('Ctrl Pts',(-2.07389218402246,-1.50090910374499,
-0.566292230810799));
#14023=CARTESIAN_POINT('Ctrl Pts',(-2.06163399970687,-1.50507975942804,
-0.611602893459367));
#14024=CARTESIAN_POINT('Ctrl Pts',(-2.04785696534972,-1.50925041078825,
-0.656493928176217));
#14025=CARTESIAN_POINT('Ctrl Pts',(-2.03255932387099,-1.51342106058787,
-0.700858470094616));
#14026=CARTESIAN_POINT('Ctrl Pts',(-1.99129602523472,-1.52467081882205,
-0.820525762898292));
#14027=CARTESIAN_POINT('Ctrl Pts',(-1.9389660390348,-1.53592056570171,-0.936360310291058));
#14028=CARTESIAN_POINT('Ctrl Pts',(-1.87691822783045,-1.547170355437,-1.04674670439718));
#14029=CARTESIAN_POINT('Ctrl Pts',(-1.82046148231699,-1.55740643796493,
-1.14718629185777));
#14030=CARTESIAN_POINT('Ctrl Pts',(-1.75596049599052,-1.56764255597309,
-1.24311491750237));
#14031=CARTESIAN_POINT('Ctrl Pts',(-1.68445696879917,-1.57787875029803,
-1.33334314829979));
#14032=CARTESIAN_POINT('Ctrl Pts',(-1.57816625909843,-1.5930949557381,-1.46746831754962));
#14033=CARTESIAN_POINT('Ctrl Pts',(-1.45611949820129,-1.60831100261461,
-1.58936165575153));
#14034=CARTESIAN_POINT('Ctrl Pts',(-1.32143778516597,-1.6235270254014,-1.69509164555733));
#14035=CARTESIAN_POINT('Ctrl Pts',(-1.2403832402782,-1.63268437701351,-1.75872237917036));
#14036=CARTESIAN_POINT('Ctrl Pts',(-1.1547533596122,-1.64184171990055,-1.81649828441596));
#14037=CARTESIAN_POINT('Ctrl Pts',(-1.06523613713058,-1.6509990833744,-1.86755775604367));
#14038=CARTESIAN_POINT('Ctrl Pts',(-1.05269294999024,-1.65228221661491,
-1.87471222855922));
#14039=CARTESIAN_POINT('Ctrl Pts',(-1.0400734483823,-1.65356535025962,-1.881734827598));
#14040=CARTESIAN_POINT('Ctrl Pts',(-1.02738058384234,-1.65484848438917,
-1.88862502197215));
#14041=CARTESIAN_POINT('Ctrl Pts',(-0.909721814516881,-1.66674272481745,
-1.95249490634092));
#14042=CARTESIAN_POINT('Ctrl Pts',(-0.785960307043669,-1.67863694886956,
-2.00488317907329));
#14043=CARTESIAN_POINT('Ctrl Pts',(-0.658433952223786,-1.6905311913999,
-2.04549523452568));
#14044=CARTESIAN_POINT('Ctrl Pts',(-0.523552452478682,-1.70311144018918,
-2.08844961015169));
#14045=CARTESIAN_POINT('Ctrl Pts',(-0.384458109946442,-1.71569170964966,
-2.11823081535576));
#14046=CARTESIAN_POINT('Ctrl Pts',(-0.243879285742567,-1.72827204102101,
-2.1344480958084));
#14047=CARTESIAN_POINT('Ctrl Pts',(-0.230670163896899,-1.7294541189825,
-2.13597191018598));
#14048=CARTESIAN_POINT('Ctrl Pts',(-0.217447917878059,-1.73063619749059,
-2.13737593637491));
#14049=CARTESIAN_POINT('Ctrl Pts',(-0.204214801524846,-1.7318182765795,
-2.13865982929153));
#14050=CARTESIAN_POINT('Ctrl Pts',(-0.0940559936059023,-1.74165846991149,
-2.14934756976135));
#14051=CARTESIAN_POINT('Ctrl Pts',(0.0170319180460684,-1.75149860472723,
-2.15172318447799));
#14052=CARTESIAN_POINT('Ctrl Pts',(0.127629739073989,-1.76133870871583,
-2.14552092692591));
#14053=CARTESIAN_POINT('Ctrl Pts',(0.229677753696459,-1.77041811974203,
-2.13979813724087));
#14054=CARTESIAN_POINT('Ctrl Pts',(0.331307399421747,-1.77949750452303,
-2.12677281393757));
#14055=CARTESIAN_POINT('Ctrl Pts',(0.431398535636282,-1.78857688481002,
-2.10627522033382));
#14056=CARTESIAN_POINT('Ctrl Pts',(0.505667078849773,-1.79531386845012,
-2.09106581744455));
#14057=CARTESIAN_POINT('Ctrl Pts',(0.579088401370791,-1.80205084961592,
-2.07174320483138));
#14058=CARTESIAN_POINT('Ctrl Pts',(0.651268888525473,-1.80878783719349,
-2.04855194526834));
#14059=CARTESIAN_POINT('Ctrl Pts',(0.758244120422034,-1.81877240278462,
-2.01418129375952));
#14060=CARTESIAN_POINT('Ctrl Pts',(0.862440456081423,-1.82875703527447,
-1.97133727426226));
#14061=CARTESIAN_POINT('Ctrl Pts',(0.962751223328877,-1.83874168737687,
-1.92078030085791));
#14062=CARTESIAN_POINT('Ctrl Pts',(1.06496440405616,-1.84891570037515,-1.86926450448427));
#14063=CARTESIAN_POINT('Ctrl Pts',(1.16314447816446,-1.85908973373697,-1.80973982527943));
#14064=CARTESIAN_POINT('Ctrl Pts',(1.25610430924613,-1.86926373743437,-1.74296009602128));
#14065=CARTESIAN_POINT('Ctrl Pts',(1.3063395294205,-1.87476173920402,-1.70687252611682));
#14066=CARTESIAN_POINT('Ctrl Pts',(1.3550498964473,-1.8802597323108,-1.66866545866889));
#14067=CARTESIAN_POINT('Ctrl Pts',(1.40204415428096,-1.88575770885973,-1.62845284783459));
#14068=CARTESIAN_POINT('Ctrl Pts',(1.47814399737386,-1.89466082111193,-1.56333482031559));
#14069=CARTESIAN_POINT('Ctrl Pts',(1.54980220057176,-1.90356391843453,-1.49290076286398));
#14070=CARTESIAN_POINT('Ctrl Pts',(1.61607511600231,-1.91246700997469,-1.41772349525774));
#14071=CARTESIAN_POINT('Ctrl Pts',(1.65006518927242,-1.91703323030488,-1.3791665551023));
#14072=CARTESIAN_POINT('Ctrl Pts',(1.68263910959245,-1.92159944911403,-1.33936265105279));
#14073=CARTESIAN_POINT('Ctrl Pts',(1.7136730378829,-1.92616566763619,-1.29839312969576));
#14074=CARTESIAN_POINT('Ctrl Pts',(1.7741799371271,-1.93506843113624,-1.21851478888014));
#14075=CARTESIAN_POINT('Ctrl Pts',(1.82882984359509,-1.9439711935454,-1.13420417698836));
#14076=CARTESIAN_POINT('Ctrl Pts',(1.87730680081322,-1.95287396400987,-1.04651803924107));
#14077=CARTESIAN_POINT('Ctrl Pts',(1.89519082923519,-1.95615835744455,-1.01416903324573));
#14078=CARTESIAN_POINT('Ctrl Pts',(1.91223517668191,-1.95944275197557,-0.98136084759658));
#14079=CARTESIAN_POINT('Ctrl Pts',(1.92842564875693,-1.96272714806214,-0.948147166408794));
#14080=CARTESIAN_POINT('Ctrl Pts',(1.97707651191226,-1.97259645291104,-0.848343142729681));
#14081=CARTESIAN_POINT('Ctrl Pts',(2.01805448866746,-1.98246583113485,-0.744813178898148));
#14082=CARTESIAN_POINT('Ctrl Pts',(2.05102784716761,-1.99233522071939,-0.638793681783248));
#14083=CARTESIAN_POINT('Ctrl Pts',(2.08377938217068,-2.0021382154139,-0.533487415491025));
#14084=CARTESIAN_POINT('Ctrl Pts',(2.10863396352524,-2.01194122131676,-0.425723679332623));
#14085=CARTESIAN_POINT('Ctrl Pts',(2.12521884429204,-2.02174417765695,-0.31669842209029));
#14086=CARTESIAN_POINT('Ctrl Pts',(2.13534325322579,-2.0277284919335,-0.250142846325303));
#14087=CARTESIAN_POINT('Ctrl Pts',(2.14238491344303,-2.03371278773996,-0.183116928193918));
#14088=CARTESIAN_POINT('Ctrl Pts',(2.14624939550719,-2.03969705125123,-0.115893013806827));
#14089=CARTESIAN_POINT('Ctrl Pts',(2.15142844512317,-2.0477169610672,-0.0258017720281359));
#14090=CARTESIAN_POINT('Ctrl Pts',(2.1508970855676,-2.05573687209812,0.0646354082577172));
#14091=CARTESIAN_POINT('Ctrl Pts',(2.14443040646274,-2.06375678802137,0.154655204293321));
#14092=CARTESIAN_POINT('Ctrl Pts',(2.13690168346352,-2.07309384101008,0.259459246338326));
#14093=CARTESIAN_POINT('Ctrl Pts',(2.1213267628892,-2.08243090063007,0.363696511439923));
#14094=CARTESIAN_POINT('Ctrl Pts',(2.09820253713493,-2.09176797268451,0.466236306460128));
#14095=CARTESIAN_POINT('Ctrl Pts',(2.07764803655949,-2.10006744419787,0.557381164590559));
#14096=CARTESIAN_POINT('Ctrl Pts',(2.05112990792501,-2.10836692553559,0.647184319962309));
#14097=CARTESIAN_POINT('Ctrl Pts',(2.01902946446485,-2.11666642077307,0.73486384668651));
#14098=CARTESIAN_POINT('',(2.67614644529864,-2.1166752978846,0.974032799954154));
#14099=CARTESIAN_POINT('Ctrl Pts',(2.67638790329494,-2.11666698860102,0.974121792631881));
#14100=CARTESIAN_POINT('Ctrl Pts',(2.67638785912941,-2.08672748700797,0.974106749158961));
#14101=CARTESIAN_POINT('Ctrl Pts',(2.67157529235006,-2.05667767012892,0.972341928041461));
#14102=CARTESIAN_POINT('Ctrl Pts',(2.66268404270861,-2.02740880552684,0.969095274171888));
#14103=CARTESIAN_POINT('Ctrl Pts',(2.65402263405934,-1.99889654828049,0.965932547104144));
#14104=CARTESIAN_POINT('Ctrl Pts',(2.64149062979418,-1.97112535002398,0.961363588377978));
#14105=CARTESIAN_POINT('Ctrl Pts',(2.62579575237343,-1.9449566292807,0.95564659024295));
#14106=CARTESIAN_POINT('Ctrl Pts',(2.61159820845988,-1.92128447486024,0.950475009102186));
#14107=CARTESIAN_POINT('Ctrl Pts',(2.59481275799209,-1.89892397248532,0.944364084064225));
#14108=CARTESIAN_POINT('Ctrl Pts',(2.57598557478357,-1.87854093566211,0.937512918344076));
#14109=CARTESIAN_POINT('Ctrl Pts',(2.55503707155986,-1.85586127573259,0.92988980948147));
#14110=CARTESIAN_POINT('Ctrl Pts',(2.53155658992225,-1.83562899381035,0.921346468856337));
#14111=CARTESIAN_POINT('Ctrl Pts',(2.50636772427429,-1.81881930830857,0.912183426472423));
#14112=CARTESIAN_POINT('Ctrl Pts',(2.47882812394535,-1.80044086972207,0.9021652490532));
#14113=CARTESIAN_POINT('Ctrl Pts',(2.44924741230612,-1.78615580340538,0.891406679152019));
#14114=CARTESIAN_POINT('Ctrl Pts',(2.4187607069639,-1.77723122603903,0.880321667073218));
#14115=CARTESIAN_POINT('Ctrl Pts',(2.39592843838876,-1.77054738319471,0.872019819756467));
#14116=CARTESIAN_POINT('Ctrl Pts',(2.37258948914726,-1.76687025757582,0.863535408372535));
#14117=CARTESIAN_POINT('Ctrl Pts',(2.34923258819565,-1.76671767765912,0.855046590252549));
#14118=CARTESIAN_POINT('Ctrl Pts',(2.34872464986128,-1.76671435953105,0.854861985447934));
#14119=CARTESIAN_POINT('Ctrl Pts',(2.34821668840943,-1.76671270731511,0.854677371654798));
#14120=CARTESIAN_POINT('Ctrl Pts',(2.34770870905014,-1.76671272653744,0.854492750764122));
#14121=CARTESIAN_POINT('Ctrl Pts',(2.32259204314204,-1.76671367697138,0.845364306574461));
#14122=CARTESIAN_POINT('Ctrl Pts',(2.29743124275574,-1.77080593190913,0.836218370574714));
#14123=CARTESIAN_POINT('Ctrl Pts',(2.27285936173094,-1.77837665826544,0.827284778016346));
#14124=CARTESIAN_POINT('Ctrl Pts',(2.24680917535251,-1.78640285831105,0.817813718355116));
#14125=CARTESIAN_POINT('Ctrl Pts',(2.22142265714173,-1.79833745252292,0.808581961916408));
#14126=CARTESIAN_POINT('Ctrl Pts',(2.19744399945536,-1.81339165766342,0.79985981724167));
#14127=CARTESIAN_POINT('Ctrl Pts',(2.17404994367491,-1.82807883988161,0.791350319265811));
#14128=CARTESIAN_POINT('Ctrl Pts',(2.15199742940655,-1.8457334718391,0.783326435636173));
#14129=CARTESIAN_POINT('Ctrl Pts',(2.13194384484284,-1.86559379902691,0.776026983036747));
#14130=CARTESIAN_POINT('Ctrl Pts',(2.12820384737706,-1.86929775395406,0.774665633691115));
#14131=CARTESIAN_POINT('Ctrl Pts',(2.12453324555184,-1.87307838964054,0.773329433815644));
#14132=CARTESIAN_POINT('Ctrl Pts',(2.12093610725898,-1.87693072872798,0.772019861055125));
#14133=CARTESIAN_POINT('Ctrl Pts',(2.09876788439411,-1.90067168737027,0.763949306506105));
#14134=CARTESIAN_POINT('Ctrl Pts',(2.07936467035814,-1.92715926223815,0.756883690562579));
#14135=CARTESIAN_POINT('Ctrl Pts',(2.06360873957658,-1.95534911991786,0.75114346667111));
#14136=CARTESIAN_POINT('Ctrl Pts',(2.04587070830782,-1.98708526955682,0.744681121012945));
#14137=CARTESIAN_POINT('Ctrl Pts',(2.03275442850618,-2.02097909692896,0.739898298179565));
#14138=CARTESIAN_POINT('Ctrl Pts',(2.02549893555319,-2.05560715796329,0.737244850782333));
#14139=CARTESIAN_POINT('Ctrl Pts',(2.02126782786752,-2.07580083138167,0.735697468440612));
#14140=CARTESIAN_POINT('Ctrl Pts',(2.01902953634433,-2.09624540533448,0.734874123352453));
#14141=CARTESIAN_POINT('Ctrl Pts',(2.01902946446485,-2.11666642077307,0.73486384668651));
#14142=CARTESIAN_POINT('Ctrl Pts',(-2.80458233589288,2.11665724005696,-0.494527021640491));
#14143=CARTESIAN_POINT('Ctrl Pts',(-2.78195692265552,2.10782585092188,-0.624275021078974));
#14144=CARTESIAN_POINT('Ctrl Pts',(-2.75048104123089,2.09899509849822,-0.752587818575418));
#14145=CARTESIAN_POINT('Ctrl Pts',(-2.71025331183979,2.09016408935099,-0.878085114837578));
#14146=CARTESIAN_POINT('Ctrl Pts',(-2.67015244924239,2.08136093068979,-1.00318662839371));
#14147=CARTESIAN_POINT('Ctrl Pts',(-2.62135498898967,2.07255751692177,-1.12548915070111));
#14148=CARTESIAN_POINT('Ctrl Pts',(-2.56400948500098,2.06375296303797,-1.243633861005));
#14149=CARTESIAN_POINT('Ctrl Pts',(-2.52310745426962,2.05747306124127,-1.32790129673196));
#14150=CARTESIAN_POINT('Ctrl Pts',(-2.47785791614011,2.05119257942859,-1.41005369783363));
#14151=CARTESIAN_POINT('Ctrl Pts',(-2.42862419207533,2.04491119646754,-1.48974196812404));
#14152=CARTESIAN_POINT('Ctrl Pts',(-2.35656441161157,2.03571759826265,-1.60637582777495));
#14153=CARTESIAN_POINT('Ctrl Pts',(-2.27600690970338,2.02652406927197,-1.71768368532288));
#14154=CARTESIAN_POINT('Ctrl Pts',(-2.18800206838966,2.01733111013869,-1.82275301439088));
#14155=CARTESIAN_POINT('Ctrl Pts',(-2.09783558126732,2.00791234613738,-1.93040314096281));
#14156=CARTESIAN_POINT('Ctrl Pts',(-1.99985064780579,1.99849418033187,-2.03150549829407));
#14157=CARTESIAN_POINT('Ctrl Pts',(-1.89512935512655,1.98907715117062,-2.1250528185535));
#14158=CARTESIAN_POINT('Ctrl Pts',(-1.83610060721461,1.98376900966265,-2.1777830804148));
#14159=CARTESIAN_POINT('Ctrl Pts',(-1.77493073132476,1.97846122929977,-2.22811233864566));
#14160=CARTESIAN_POINT('Ctrl Pts',(-1.71180854829565,1.97315390651591,-2.27585485864977));
#14161=CARTESIAN_POINT('Ctrl Pts',(-1.61043745719953,1.96463060970357,-2.35252697473078));
#14162=CARTESIAN_POINT('Ctrl Pts',(-1.50392997092724,1.95610753076537,-2.42259747247663));
#14163=CARTESIAN_POINT('Ctrl Pts',(-1.39318682599955,1.94758406792774,-2.48516487943052));
#14164=CARTESIAN_POINT('Ctrl Pts',(-1.30044328685753,1.9404459637153,-2.53756291056491));
#14165=CARTESIAN_POINT('Ctrl Pts',(-1.20473011838826,1.93330759025575,-2.58469891486034));
#14166=CARTESIAN_POINT('Ctrl Pts',(-1.10659388581258,1.92616859409453,-2.62606546345969));
#14167=CARTESIAN_POINT('Ctrl Pts',(-0.993148428790342,1.91791591655705,
-2.67388518190738));
#14168=CARTESIAN_POINT('Ctrl Pts',(-0.876465346112244,1.90966240688131,
-2.71399381805545));
#14169=CARTESIAN_POINT('Ctrl Pts',(-0.757696549627284,1.90140751904957,
-2.7463426951939));
#14170=CARTESIAN_POINT('Ctrl Pts',(-0.626181159144015,1.89226669394469,
-2.78216334282587));
#14171=CARTESIAN_POINT('Ctrl Pts',(-0.492130004822071,1.88312627592044,
-2.80847279982899));
#14172=CARTESIAN_POINT('Ctrl Pts',(-0.356898911517837,1.87398652541256,
-2.82527490060671));
#14173=CARTESIAN_POINT('Ctrl Pts',(-0.21960563696361,1.86470739998973,-2.84233322187587));
#14174=CARTESIAN_POINT('Ctrl Pts',(-0.0810949057590346,1.85542896259683,
-2.8495921840046));
#14175=CARTESIAN_POINT('Ctrl Pts',(0.0572283211157545,1.84615148576666,
-2.84700464260265));
#14176=CARTESIAN_POINT('Ctrl Pts',(0.139230104201676,1.84065154436274,-2.84547067745765));
#14177=CARTESIAN_POINT('Ctrl Pts',(0.221166160679518,1.83515194054302,-2.8404752344192));
#14178=CARTESIAN_POINT('Ctrl Pts',(0.30274321958312,1.8296527310885,-2.83199983632318));
#14179=CARTESIAN_POINT('Ctrl Pts',(0.42569985615815,1.82136407362233,-2.81922533258981));
#14180=CARTESIAN_POINT('Ctrl Pts',(0.547929990333508,1.81307516416304,-2.79853030292443));
#14181=CARTESIAN_POINT('Ctrl Pts',(0.668253724755781,1.8047857434996,-2.76984910916053));
#14182=CARTESIAN_POINT('Ctrl Pts',(0.746648213223421,1.79938493961228,-2.75116245914457));
#14183=CARTESIAN_POINT('Ctrl Pts',(0.82423327113268,1.79398391872342,-2.72908680139804));
#14184=CARTESIAN_POINT('Ctrl Pts',(0.900683703946973,1.78858260914337,-2.70361587160169));
#14185=CARTESIAN_POINT('Ctrl Pts',(1.01786233849029,1.78030380602824,-2.66457555928147));
#14186=CARTESIAN_POINT('Ctrl Pts',(1.13237393427125,1.77202432469325,-2.61755666473922));
#14187=CARTESIAN_POINT('Ctrl Pts',(1.24330248133285,1.76374390699457,-2.56329332031478));
#14188=CARTESIAN_POINT('Ctrl Pts',(1.26938375238872,1.76179703376693,-2.55053504454339));
#14189=CARTESIAN_POINT('Ctrl Pts',(1.2952670635135,1.75985010877677,-2.53737649080999));
#14190=CARTESIAN_POINT('Ctrl Pts',(1.3209407377059,1.75790312866889,-2.52382754784158));
#14191=CARTESIAN_POINT('Ctrl Pts',(1.44045818507747,1.74883944378948,-2.46075379119761));
#14192=CARTESIAN_POINT('Ctrl Pts',(1.55546286758081,1.73977653023493,-2.38920902392338));
#14193=CARTESIAN_POINT('Ctrl Pts',(1.66496510134029,1.73071439590768,-2.31005428671678));
#14194=CARTESIAN_POINT('Ctrl Pts',(1.77514668187161,1.72159604052,-2.23040847719732));
#14195=CARTESIAN_POINT('Ctrl Pts',(1.87975834022544,1.7124784740582,-2.14305722122181));
#14196=CARTESIAN_POINT('Ctrl Pts',(1.97776537519384,1.70336170457275,-2.04883305684583));
#14197=CARTESIAN_POINT('Ctrl Pts',(2.0394413901976,1.69762450405697,-1.98953760955835));
#14198=CARTESIAN_POINT('Ctrl Pts',(2.09850125673617,1.69188761916048,-1.92751949672681));
#14199=CARTESIAN_POINT('Ctrl Pts',(2.15467902364597,1.68615105188955,-1.86297929705858));
#14200=CARTESIAN_POINT('Ctrl Pts',(2.23506632755639,1.67794233869256,-1.77062581042926));
#14201=CARTESIAN_POINT('Ctrl Pts',(2.30958423117854,1.66973293664819,-1.67306262287684));
#14202=CARTESIAN_POINT('Ctrl Pts',(2.37733115154558,1.66152289082693,-1.57100557093827));
#14203=CARTESIAN_POINT('Ctrl Pts',(2.40628489938846,1.65801407307995,-1.5273883241113));
#14204=CARTESIAN_POINT('Ctrl Pts',(2.43400232755433,1.6545051377442,-1.48295073002168));
#14205=CARTESIAN_POINT('Ctrl Pts',(2.46041525696606,1.65099608833801,-1.43775059105066));
#14206=CARTESIAN_POINT('Ctrl Pts',(2.52223089679436,1.64278366589703,-1.3319662054088));
#14207=CARTESIAN_POINT('Ctrl Pts',(2.57689806784256,1.63457061866224,-1.22200385757481));
#14208=CARTESIAN_POINT('Ctrl Pts',(2.6242135385369,1.62635699173425,-1.1089945602547));
#14209=CARTESIAN_POINT('Ctrl Pts',(2.64717459106986,1.62237111741847,-1.05415388395152));
#14210=CARTESIAN_POINT('Ctrl Pts',(2.66840510749953,1.61838510658923,-0.998595985561653));
#14211=CARTESIAN_POINT('Ctrl Pts',(2.68788611968169,1.61439896440059,-0.942451252524915));
#14212=CARTESIAN_POINT('Ctrl Pts',(2.73243195458445,1.6052841386321,-0.814069113797786));
#14213=CARTESIAN_POINT('Ctrl Pts',(2.76786121198766,1.59617037125586,-0.682546337603376));
#14214=CARTESIAN_POINT('Ctrl Pts',(2.79398463412037,1.58705744696499,-0.549200789547298));
#14215=CARTESIAN_POINT('Ctrl Pts',(2.82004885042824,1.57796517610141,-0.41615745431471));
#14216=CARTESIAN_POINT('Ctrl Pts',(2.83684955611659,1.56887374450604,-0.281298348456388));
#14217=CARTESIAN_POINT('Ctrl Pts',(2.84414931768941,1.5597829383326,-0.145920560005815));
#14218=CARTESIAN_POINT('Ctrl Pts',(2.84873544117182,1.55407157923543,-0.060868569140493));
#14219=CARTESIAN_POINT('Ctrl Pts',(2.84957048782428,1.54836046699627,0.0243883193675018));
#14220=CARTESIAN_POINT('Ctrl Pts',(2.84658502904739,1.54264954858617,0.109527498678143));
#14221=CARTESIAN_POINT('Ctrl Pts',(2.84224367557131,1.5343449236209,0.23333402212198));
#14222=CARTESIAN_POINT('Ctrl Pts',(2.82981710043464,1.52603917879535,0.356908951255374));
#14223=CARTESIAN_POINT('Ctrl Pts',(2.80910367996215,1.5177326713053,0.479083523772095));
#14224=CARTESIAN_POINT('Ctrl Pts',(2.80551079386501,1.51629185010841,0.500275548701168));
#14225=CARTESIAN_POINT('Ctrl Pts',(2.80166870570173,1.51485100596501,0.521425439142127));
#14226=CARTESIAN_POINT('Ctrl Pts',(2.79757652440072,1.51341014073923,0.54252710241733));
#14227=CARTESIAN_POINT('Ctrl Pts',(2.77394067383935,1.50508791045412,0.664407274159863));
#14228=CARTESIAN_POINT('Ctrl Pts',(2.74195745366128,1.49676497685038,0.784677265492543));
#14229=CARTESIAN_POINT('Ctrl Pts',(2.70223914758,1.48844169912296,0.902317170192954));
#14230=CARTESIAN_POINT('Ctrl Pts',(2.67432890489442,1.48259289225702,0.98498329102345));
#14231=CARTESIAN_POINT('Ctrl Pts',(2.64260028236357,1.47674391546488,1.06635087545059));
#14232=CARTESIAN_POINT('Ctrl Pts',(2.60727944653752,1.4708948933841,1.14607297111354));
#14233=CARTESIAN_POINT('Ctrl Pts',(2.55107174904667,1.46158707107342,1.2729384693828));
#14234=CARTESIAN_POINT('Ctrl Pts',(2.48572431206794,1.45228057614097,1.39575090488485));
#14235=CARTESIAN_POINT('Ctrl Pts',(2.41200087454017,1.44297495438738,1.51331153309315));
#14236=CARTESIAN_POINT('Ctrl Pts',(2.33912082498289,1.43377578791732,1.62952728071858));
#14237=CARTESIAN_POINT('Ctrl Pts',(2.2580545758542,1.42457747476227,1.74061172045069));
#14238=CARTESIAN_POINT('Ctrl Pts',(2.16949824700251,1.41537957613314,1.84537958337022));
#14239=CARTESIAN_POINT('Ctrl Pts',(2.11740532649016,1.40996894757185,1.90700887656795));
#14240=CARTESIAN_POINT('Ctrl Pts',(2.06271985469377,1.40455846245042,1.96645183280968));
#14241=CARTESIAN_POINT('Ctrl Pts',(2.00557821089282,1.39914803145207,2.02346054546564));
#14242=CARTESIAN_POINT('Ctrl Pts',(1.92348429671894,1.39137500588827,2.10536348091922));
#14243=CARTESIAN_POINT('Ctrl Pts',(1.83633357380992,1.38360069944669,2.18222360846758));
#14244=CARTESIAN_POINT('Ctrl Pts',(1.74463343531627,1.37582563843094,2.25322530463692));
#14245=CARTESIAN_POINT('Ctrl Pts',(1.64304360701143,1.36721205150921,2.33188440201326));
#14246=CARTESIAN_POINT('Ctrl Pts',(1.53587039232361,1.3585975384778,2.40335199327399));
#14247=CARTESIAN_POINT('Ctrl Pts',(1.42435621965327,1.34998281494774,2.46723143747144));
#14248=CARTESIAN_POINT('Ctrl Pts',(1.32687558837224,1.34245221441587,2.52307194991157));
#14249=CARTESIAN_POINT('Ctrl Pts',(1.22607884688904,1.33492145303225,2.57311451942267));
#14250=CARTESIAN_POINT('Ctrl Pts',(1.12280743727165,1.32739100881219,2.61712470493613));
#14251=CARTESIAN_POINT('Ctrl Pts',(0.990207240359367,1.31772193980155,2.67363365825489));
#14252=CARTESIAN_POINT('Ctrl Pts',(0.853379606627105,1.30805447587311,2.72026934000668));
#14253=CARTESIAN_POINT('Ctrl Pts',(0.713861018160752,1.29838786904702,2.75656592271339));
#14254=CARTESIAN_POINT('Ctrl Pts',(0.577367304017838,1.28893084197014,2.79207556654503));
#14255=CARTESIAN_POINT('Ctrl Pts',(0.438296805635782,1.27947463523317,2.81768977284684));
#14256=CARTESIAN_POINT('Ctrl Pts',(0.298080367904077,1.27001854845938,2.83292424809103));
#14257=CARTESIAN_POINT('Ctrl Pts',(0.227042875518054,1.26522783559389,2.84064245101125));
#14258=CARTESIAN_POINT('Ctrl Pts',(0.155711241883743,1.2604371535195,2.84569568310527));
#14259=CARTESIAN_POINT('Ctrl Pts',(0.0842722593669868,1.25564641116154,
2.84801583840595));
#14260=CARTESIAN_POINT('Ctrl Pts',(-0.00222290094123247,1.24984599220751,
2.85082497982428));
#14261=CARTESIAN_POINT('Ctrl Pts',(-0.0888424845338625,1.24404474795043,
2.84962541460311));
#14262=CARTESIAN_POINT('Ctrl Pts',(-0.17521088761524,1.23824297558038,2.84430505124541));
#14263=CARTESIAN_POINT('Ctrl Pts',(-0.311666308540717,1.22907662234674,
2.8358992871517));
#14264=CARTESIAN_POINT('Ctrl Pts',(-0.447493850899554,1.21990895086045,
2.81720476888644));
#14265=CARTESIAN_POINT('Ctrl Pts',(-0.581278969526878,1.21074113316035,
2.78884600173747));
#14266=CARTESIAN_POINT('Ctrl Pts',(-0.711907039215729,1.20178965678008,
2.76115644217036));
#14267=CARTESIAN_POINT('Ctrl Pts',(-0.840586922470479,1.19283804100528,
2.72425404482427));
#14268=CARTESIAN_POINT('Ctrl Pts',(-0.966020705809652,1.18388737684435,
2.67876424010694));
#14269=CARTESIAN_POINT('Ctrl Pts',(-1.11059363914152,1.17357098728354,2.62633343295434));
#14270=CARTESIAN_POINT('Ctrl Pts',(-1.25105662977625,1.16325655063408,2.56243126293453));
#14271=CARTESIAN_POINT('Ctrl Pts',(-1.3856020394883,1.15294287837623,2.48785423186171));
#14272=CARTESIAN_POINT('Ctrl Pts',(-1.5155161453378,1.14298422194736,2.41584428124748));
#14273=CARTESIAN_POINT('Ctrl Pts',(-1.63991404568272,1.13302627819219,2.33388097949739));
#14274=CARTESIAN_POINT('Ctrl Pts',(-1.75713727350267,1.12306797714789,2.24264513907806));
#14275=CARTESIAN_POINT('Ctrl Pts',(-1.799997721801,1.11942691338445,2.20928648572948));
#14276=CARTESIAN_POINT('Ctrl Pts',(-1.84189863558586,1.11578580185645,2.17468791758819));
#14277=CARTESIAN_POINT('Ctrl Pts',(-1.8827574653352,1.11214459026435,2.13888172789186));
#14278=CARTESIAN_POINT('Ctrl Pts',(-1.92570430221763,1.10831730198274,2.10124573592381));
#14279=CARTESIAN_POINT('Ctrl Pts',(-1.96748293849158,1.10448963806102,2.06229011400923));
#14280=CARTESIAN_POINT('Ctrl Pts',(-2.00799362759083,1.10066169833689,2.02206122998739));
#14281=CARTESIAN_POINT('Ctrl Pts',(-2.1158473025442,1.09047037905974,1.91495781907288));
#14282=CARTESIAN_POINT('Ctrl Pts',(-2.21471041744568,1.08027710486391,1.79882743654177));
#14283=CARTESIAN_POINT('Ctrl Pts',(-2.30372169493775,1.07008375979099,1.67556698066195));
#14284=CARTESIAN_POINT('Ctrl Pts',(-2.39017505429039,1.06018334099661,1.55584866196802));
#14285=CARTESIAN_POINT('Ctrl Pts',(-2.4673343500471,1.05028285534021,1.42940544772771));
#14286=CARTESIAN_POINT('Ctrl Pts',(-2.53445489838778,1.04038402906109,1.29799088753696));
#14287=CARTESIAN_POINT('Ctrl Pts',(-2.61554686873761,1.02842472081692,1.13922183868422));
#14288=CARTESIAN_POINT('Ctrl Pts',(-2.68213302783367,1.01646812482486,0.972930314429998));
#14289=CARTESIAN_POINT('Ctrl Pts',(-2.7328636458305,1.0045119563375,0.801945004864593));
#14290=CARTESIAN_POINT('Ctrl Pts',(-2.77931928941865,0.993563311833254,
0.64536830791847));
#14291=CARTESIAN_POINT('Ctrl Pts',(-2.81247886793264,0.982615025819403,
0.484854447140363));
#14292=CARTESIAN_POINT('Ctrl Pts',(-2.83125821150622,0.97166534383724,0.322581819316084));
#14293=CARTESIAN_POINT('Ctrl Pts',(-2.83298633767105,0.970657724382605,
0.307649051678014));
#14294=CARTESIAN_POINT('Ctrl Pts',(-2.83459265425157,0.96965009310666,0.292701401630804));
#14295=CARTESIAN_POINT('Ctrl Pts',(-2.83607629458685,0.968642448642216,
0.277740574396832));
#14296=CARTESIAN_POINT('Ctrl Pts',(-2.83880587230564,0.966788600500464,
0.250215884146019));
#14297=CARTESIAN_POINT('Ctrl Pts',(-2.84111956607568,0.96493467000898,0.222653121347949));
#14298=CARTESIAN_POINT('Ctrl Pts',(-2.84301252487888,0.96308066892502,0.195063450417379));
#14299=CARTESIAN_POINT('Ctrl Pts',(-2.85561123541669,0.950741244023576,
0.0114385995752131));
#14300=CARTESIAN_POINT('Ctrl Pts',(-2.84956951455601,0.938398692119184,
-0.173376147093211));
#14301=CARTESIAN_POINT('Ctrl Pts',(-2.82597651771739,0.926056479468952,
-0.355930500791568));
#14302=CARTESIAN_POINT('Ctrl Pts',(-2.80738470726687,0.916330539195121,
-0.499787424271555));
#14303=CARTESIAN_POINT('Ctrl Pts',(-2.7778948576424,0.906604809591102,-0.642240748807444));
#14304=CARTESIAN_POINT('Ctrl Pts',(-2.73805633784352,0.896880986854682,
-0.781618227284983));
#14305=CARTESIAN_POINT('Ctrl Pts',(-2.68219190584366,0.883245544655029,
-0.977063331872888));
#14306=CARTESIAN_POINT('Ctrl Pts',(-2.60587050090985,0.869613649916618,
-1.16685079029084));
#14307=CARTESIAN_POINT('Ctrl Pts',(-2.510357866132,0.855981266040079,-1.3463984534859));
#14308=CARTESIAN_POINT('Ctrl Pts',(-2.43917350435211,0.845821222313435,
-1.48021306181849));
#14309=CARTESIAN_POINT('Ctrl Pts',(-2.35732930885754,0.835660906893434,
-1.60833903565359));
#14310=CARTESIAN_POINT('Ctrl Pts',(-2.26535011224914,0.825498648739708,
-1.72886054990566));
#14311=CARTESIAN_POINT('Ctrl Pts',(-2.26426761998683,0.82537905032806,-1.73027895332111));
#14312=CARTESIAN_POINT('Ctrl Pts',(-2.26318372397246,0.825259451647331,
-1.73169630326915));
#14313=CARTESIAN_POINT('Ctrl Pts',(-2.26209842687303,0.825139852694796,
-1.73311259799423));
#14314=CARTESIAN_POINT('Ctrl Pts',(-2.14142969266093,0.811842245778572,
-1.89058329596036));
#14315=CARTESIAN_POINT('Ctrl Pts',(-2.00366546403506,0.798541291076087,
-2.03472132532182));
#14316=CARTESIAN_POINT('Ctrl Pts',(-1.85262348342731,0.785240915843383,
-2.16327288912423));
#14317=CARTESIAN_POINT('Ctrl Pts',(-1.73199858567728,0.774618992084,-2.26593652725237));
#14318=CARTESIAN_POINT('Ctrl Pts',(-1.60290395110196,0.763997437905361,
-2.3586595711926));
#14319=CARTESIAN_POINT('Ctrl Pts',(-1.46726066438,0.75337825366249,-2.44029700691361));
#14320=CARTESIAN_POINT('Ctrl Pts',(-1.31445136477984,0.741415183866013,
-2.53226587374926));
#14321=CARTESIAN_POINT('Ctrl Pts',(-1.15306195631937,0.729454649678202,
-2.61032190563498));
#14322=CARTESIAN_POINT('Ctrl Pts',(-0.985839578997115,0.717493702838762,
-2.67265181028179));
#14323=CARTESIAN_POINT('Ctrl Pts',(-0.848015707358323,0.707635548515908,
-2.72402381512266));
#14324=CARTESIAN_POINT('Ctrl Pts',(-0.706230953840882,0.697777113879811,
-2.76471322800078));
#14325=CARTESIAN_POINT('Ctrl Pts',(-0.562044485381816,0.687916748276768,
-2.79372079692265));
#14326=CARTESIAN_POINT('Ctrl Pts',(-0.531435194482997,0.685823494989287,
-2.79987880276665));
#14327=CARTESIAN_POINT('Ctrl Pts',(-0.500717716471415,0.683730154679143,
-2.80551040642833));
#14328=CARTESIAN_POINT('Ctrl Pts',(-0.469909449984022,0.681636711554149,
-2.81061812312463));
#14329=CARTESIAN_POINT('Ctrl Pts',(-0.311384277657102,0.670864815891595,
-2.83690008448744));
#14330=CARTESIAN_POINT('Ctrl Pts',(-0.150671980668343,0.660091482015627,
-2.84927975948678));
#14331=CARTESIAN_POINT('Ctrl Pts',(0.0099591028400281,0.64931841187939,
-2.84821053083917));
#14332=CARTESIAN_POINT('Ctrl Pts',(0.17896284199308,0.637983811530465,-2.84708557024308));
#14333=CARTESIAN_POINT('Ctrl Pts',(0.34787789599397,0.626649503131862,-2.83107334950554));
#14334=CARTESIAN_POINT('Ctrl Pts',(0.51408428978591,0.615317468884971,-2.80064983867025));
#14335=CARTESIAN_POINT('Ctrl Pts',(0.540689324805138,0.613503524420505,
-2.79577987817887));
#14336=CARTESIAN_POINT('Ctrl Pts',(0.567224975267696,0.61168963822693,-2.79054054879862));
#14337=CARTESIAN_POINT('Ctrl Pts',(0.59368050928722,0.609875818434349,-2.78493368240782));
#14338=CARTESIAN_POINT('Ctrl Pts',(0.739823533721816,0.599856095904029,
-2.75396078988004));
#14339=CARTESIAN_POINT('Ctrl Pts',(0.883727347479231,0.589837817515454,
-2.71172418574845));
#14340=CARTESIAN_POINT('Ctrl Pts',(1.02342699697088,0.579819329519902,-2.65849030561885));
#14341=CARTESIAN_POINT('Ctrl Pts',(1.16046079679312,0.569992021552417,-2.60627227286081));
#14342=CARTESIAN_POINT('Ctrl Pts',(1.29344805073623,0.560164511901412,-2.54347303709899));
#14343=CARTESIAN_POINT('Ctrl Pts',(1.42053874146158,0.550335239697112,-2.47039258642219));
#14344=CARTESIAN_POINT('Ctrl Pts',(1.47312477640536,0.546268203404703,-2.44015424944357));
#14345=CARTESIAN_POINT('Ctrl Pts',(1.52470146343064,0.54220086535649,-2.40815628242956));
#14346=CARTESIAN_POINT('Ctrl Pts',(1.57518338415778,0.538133114982619,-2.37449979056686));
#14347=CARTESIAN_POINT('Ctrl Pts',(1.69729820182146,0.528293303262863,-2.29308536916979));
#14348=CARTESIAN_POINT('Ctrl Pts',(1.81289131980392,0.518452892961791,-2.20204937750933));
#14349=CARTESIAN_POINT('Ctrl Pts',(1.92091735073199,0.508612868932424,-2.10277545645514));
#14350=CARTESIAN_POINT('Ctrl Pts',(2.03287349302946,0.498414853500606,-1.99988983586455));
#14351=CARTESIAN_POINT('Ctrl Pts',(2.13670294434962,0.488217252957753,-1.88815519413113));
#14352=CARTESIAN_POINT('Ctrl Pts',(2.23121668812399,0.478021163605228,-1.76906264376533));
#14353=CARTESIAN_POINT('Ctrl Pts',(2.26720817603854,0.474138422195861,-1.72371137615037));
#14354=CARTESIAN_POINT('Ctrl Pts',(2.30184842051047,0.470255899930118,-1.67729267913346));
#14355=CARTESIAN_POINT('Ctrl Pts',(2.33507036011353,0.466373657348281,-1.62988750356013));
#14356=CARTESIAN_POINT('Ctrl Pts',(2.41273176910905,0.457298316396783,-1.51907059242573));
#14357=CARTESIAN_POINT('Ctrl Pts',(2.48273157246174,0.448223760354261,-1.40272772949553));
#14358=CARTESIAN_POINT('Ctrl Pts',(2.54408129257416,0.4391489482232,-1.28199626892511));
#14359=CARTESIAN_POINT('Ctrl Pts',(2.60356074674044,0.430350784658185,-1.16494534575437));
#14360=CARTESIAN_POINT('Ctrl Pts',(2.65490892647938,0.421552380380548,-1.04377036445469));
#14361=CARTESIAN_POINT('Ctrl Pts',(2.69726206377657,0.412752786725291,-0.919536395873714));
#14362=CARTESIAN_POINT('Ctrl Pts',(2.72633564009712,0.406712250556015,-0.83425521016603));
#14363=CARTESIAN_POINT('Ctrl Pts',(2.75117138033395,0.400671153925594,-0.747533168042571));
#14364=CARTESIAN_POINT('Ctrl Pts',(2.7717797395978,0.394629189966113,-0.659813786973422));
#14365=CARTESIAN_POINT('Ctrl Pts',(2.80375197296895,0.385255562533699,-0.523724130984334));
#14366=CARTESIAN_POINT('Ctrl Pts',(2.82553726556799,0.375881893634451,-0.385313547487032));
#14367=CARTESIAN_POINT('Ctrl Pts',(2.83724652168304,0.366508758774783,-0.246056202140706));
#14368=CARTESIAN_POINT('Ctrl Pts',(2.84925229116111,0.356898268124789,-0.103272444579225));
#14369=CARTESIAN_POINT('Ctrl Pts',(2.85066541482192,0.347288338903776,0.0404027634423335));
#14370=CARTESIAN_POINT('Ctrl Pts',(2.84155340634652,0.337679591455343,0.18339543013698));
#14371=CARTESIAN_POINT('Ctrl Pts',(2.83687230357611,0.332743299481687,0.256854906170083));
#14372=CARTESIAN_POINT('Ctrl Pts',(2.82941258685957,0.32780731939845,0.330134368779524));
#14373=CARTESIAN_POINT('Ctrl Pts',(2.81917806754171,0.322871735313071,0.403020188466609));
#14374=CARTESIAN_POINT('Ctrl Pts',(2.80142248463043,0.314309127757034,0.529467769864187));
#14375=CARTESIAN_POINT('Ctrl Pts',(2.77529267449128,0.305746785348526,0.654854651051419));
#14376=CARTESIAN_POINT('Ctrl Pts',(2.74079858797234,0.297184076994133,0.777892924300791));
#14377=CARTESIAN_POINT('Ctrl Pts',(2.71123783404779,0.289846004294255,0.883334305298909));
#14378=CARTESIAN_POINT('Ctrl Pts',(2.675535086332,0.282507662838135,0.987050215039095));
#14379=CARTESIAN_POINT('Ctrl Pts',(2.63372688779794,0.275168655428478,1.08823367223257));
#14380=CARTESIAN_POINT('Ctrl Pts',(2.58807592749233,0.267155089963133,1.19871731299886));
#14381=CARTESIAN_POINT('Ctrl Pts',(2.53514542312535,0.259140730497123,1.30618070531776));
#14382=CARTESIAN_POINT('Ctrl Pts',(2.47565204537744,0.251125059933902,1.40985110762689));
#14383=CARTESIAN_POINT('Ctrl Pts',(2.40780838796007,0.241984338256172,1.52807232021941));
#14384=CARTESIAN_POINT('Ctrl Pts',(2.33145002966693,0.232843999637142,1.64134427148275));
#14385=CARTESIAN_POINT('Ctrl Pts',(2.24754333145362,0.223704325212609,1.74871557175885));
#14386=CARTESIAN_POINT('Ctrl Pts',(2.16228962806164,0.214417926044483,1.85781056871938));
#14387=CARTESIAN_POINT('Ctrl Pts',(2.06924251621642,0.205132212567469,1.96081494828424));
#14388=CARTESIAN_POINT('Ctrl Pts',(1.96936951706988,0.195847479675699,2.0567044677364));
#14389=CARTESIAN_POINT('Ctrl Pts',(1.91028458189457,0.190354625293452,2.11343277357719));
#14390=CARTESIAN_POINT('Ctrl Pts',(1.84880982925535,0.184862114107581,2.16767036869738));
#14391=CARTESIAN_POINT('Ctrl Pts',(1.78513987983399,0.179370007177408,2.21919873359685));
#14392=CARTESIAN_POINT('Ctrl Pts',(1.68894916907077,0.171072691504912,2.29704629102687));
#14393=CARTESIAN_POINT('Ctrl Pts',(1.58767192555512,0.162775177956397,2.3687647574989));
#14394=CARTESIAN_POINT('Ctrl Pts',(1.48210122139711,0.154477168518722,2.43347386498712));
#14395=CARTESIAN_POINT('Ctrl Pts',(1.41045945317825,0.148846022325721,2.47738637762303));
#14396=CARTESIAN_POINT('Ctrl Pts',(1.33684137980812,0.143214647767288,2.51807155841732));
#14397=CARTESIAN_POINT('Ctrl Pts',(1.26150357893371,0.137582951710285,2.55526488394704));
#14398=CARTESIAN_POINT('Ctrl Pts',(1.15066666393052,0.129297604780205,2.60998367600861));
#14399=CARTESIAN_POINT('Ctrl Pts',(1.03610718865871,0.121011561989863,2.6571422134355));
#14400=CARTESIAN_POINT('Ctrl Pts',(0.918995430112488,0.112724526775131,
2.696618264617));
#14401=CARTESIAN_POINT('Ctrl Pts',(0.894954400175827,0.111023340966322,
2.7047220190138));
#14402=CARTESIAN_POINT('Ctrl Pts',(0.870805859448953,0.109322113335728,
2.71250219525392));
#14403=CARTESIAN_POINT('Ctrl Pts',(0.846559984942935,0.107620841317824,
2.71995800043706));
#14404=CARTESIAN_POINT('Ctrl Pts',(0.717441227963609,0.0985609029691008,
2.75966307674962));
#14405=CARTESIAN_POINT('Ctrl Pts',(0.585538508374012,0.0895016936606722,
2.79018113528876));
#14406=CARTESIAN_POINT('Ctrl Pts',(0.452160387528534,0.0804432509080095,
2.81142975491808));
#14407=CARTESIAN_POINT('Ctrl Pts',(0.317796625702479,0.0713178678480413,
2.83283539812933));
#14408=CARTESIAN_POINT('Ctrl Pts',(0.181934324020822,0.0621932627151443,
2.84483427845823));
#14409=CARTESIAN_POINT('Ctrl Pts',(0.0458981191767985,0.0530694738626992,
2.84729178064325));
#14410=CARTESIAN_POINT('Ctrl Pts',(-0.0395963040053689,0.0473354630817454,
2.8488362425166));
#14411=CARTESIAN_POINT('Ctrl Pts',(-0.125159610904366,0.0416017747088944,
2.84661111327967));
#14412=CARTESIAN_POINT('Ctrl Pts',(-0.210462215375585,0.0358684182644795,
2.84057242424866));
#14413=CARTESIAN_POINT('Ctrl Pts',(-0.332628311613721,0.0276573937653124,
2.83192411778853));
#14414=CARTESIAN_POINT('Ctrl Pts',(-0.454318949508754,0.0194457328714482,
2.81544408284231));
#14415=CARTESIAN_POINT('Ctrl Pts',(-0.574388741029553,0.0112334439036321,
2.79100586565238));
#14416=CARTESIAN_POINT('Ctrl Pts',(-0.62915108024243,0.007487921000048,
2.77985989860636));
#14417=CARTESIAN_POINT('Ctrl Pts',(-0.68357621353279,0.00374226744711259,
2.7670592115551));
#14418=CARTESIAN_POINT('Ctrl Pts',(-0.737555719985232,-3.51596576807223E-6,
2.75259542039799));
#14419=CARTESIAN_POINT('Ctrl Pts',(-0.855910739555236,-0.00821648970844346,
2.72088223148684));
#14420=CARTESIAN_POINT('Ctrl Pts',(-0.972121952743627,-0.016430087747433,
2.68117054902539));
#14421=CARTESIAN_POINT('Ctrl Pts',(-1.08524943432292,-0.0246443017617273,
2.63412173290116));
#14422=CARTESIAN_POINT('Ctrl Pts',(-1.13684304884904,-0.0283905266893244,
2.61266436065937));
#14423=CARTESIAN_POINT('Ctrl Pts',(-1.1877955424641,-0.0321368797375203,
2.58968156208569));
#14424=CARTESIAN_POINT('Ctrl Pts',(-1.23801956154725,-0.0358833601169834,
2.56523916887831));
#14425=CARTESIAN_POINT('Ctrl Pts',(-1.36006367903396,-0.0449872888733795,
2.50584427450875));
#14426=CARTESIAN_POINT('Ctrl Pts',(-1.47787419080016,-0.0540901924371456,
2.43780365338667));
#14427=CARTESIAN_POINT('Ctrl Pts',(-1.59039424635548,-0.0631922589418942,
2.36191920832476));
#14428=CARTESIAN_POINT('Ctrl Pts',(-1.70277447939221,-0.0722830148064472,
2.28612906071213));
#14429=CARTESIAN_POINT('Ctrl Pts',(-1.80987841761559,-0.0813729356910015,
2.20251382274258));
#14430=CARTESIAN_POINT('Ctrl Pts',(-1.91062667852844,-0.0904622090286987,
2.11182884014686));
#14431=CARTESIAN_POINT('Ctrl Pts',(-1.9740717901352,-0.0961860791591553,
2.05472096761674));
#14432=CARTESIAN_POINT('Ctrl Pts',(-2.03499584355038,-0.10190969249116,
1.99480860783181));
#14433=CARTESIAN_POINT('Ctrl Pts',(-2.09312110392871,-0.107633095833601,
1.93227353006217));
#14434=CARTESIAN_POINT('Ctrl Pts',(-2.17725469900751,-0.115917454409398,
1.84175693061733));
#14435=CARTESIAN_POINT('Ctrl Pts',(-2.25553549330611,-0.124202880489431,
1.74572510198876));
#14436=CARTESIAN_POINT('Ctrl Pts',(-2.32700347370338,-0.13248905593599,
1.64486162842615));
#14437=CARTESIAN_POINT('Ctrl Pts',(-2.34166723806075,-0.134189209256356,
1.6241665115309));
#14438=CARTESIAN_POINT('Ctrl Pts',(-2.35604431386819,-0.135889394124023,
1.60326811487315));
#14439=CARTESIAN_POINT('Ctrl Pts',(-2.37012661068211,-0.137589607790991,
1.58217252837426));
#14440=CARTESIAN_POINT('Ctrl Pts',(-2.43887420373001,-0.145889787713038,
1.47918714077051));
#14441=CARTESIAN_POINT('Ctrl Pts',(-2.50059269511661,-0.154190653991916,
1.37150029709983));
#14442=CARTESIAN_POINT('Ctrl Pts',(-2.55500200152593,-0.162491886908244,
1.26025962660104));
#14443=CARTESIAN_POINT('Ctrl Pts',(-2.59191434546933,-0.168123606641198,
1.18479176713129));
#14444=CARTESIAN_POINT('Ctrl Pts',(-2.62546356838125,-0.173755495120222,
1.10768889203951));
#14445=CARTESIAN_POINT('Ctrl Pts',(-2.65557518457384,-0.17938745251458,
1.02931353467584));
#14446=CARTESIAN_POINT('Ctrl Pts',(-2.70517097227751,-0.188663652154619,
0.900224230397167));
#14447=CARTESIAN_POINT('Ctrl Pts',(-2.74548922999383,-0.197938556591528,
0.76757664521583));
#14448=CARTESIAN_POINT('Ctrl Pts',(-2.77623467558263,-0.207212589244025,
0.632745539129348));
#14449=CARTESIAN_POINT('Ctrl Pts',(-2.80666391168401,-0.216391240708993,
0.499301138427257));
#14450=CARTESIAN_POINT('Ctrl Pts',(-2.82771643357988,-0.225569038229503,
0.363716648488724));
#14451=CARTESIAN_POINT('Ctrl Pts',(-2.83905719972122,-0.234746392293966,
0.227314229871604));
#14452=CARTESIAN_POINT('Ctrl Pts',(-2.84580784954219,-0.240209259863949,
0.146119983262331));
#14453=CARTESIAN_POINT('Ctrl Pts',(-2.84911640035801,-0.24567197030472,
0.064635807190785));
#14454=CARTESIAN_POINT('Ctrl Pts',(-2.84890338395658,-0.251134610194849,
-0.0168585082596733));
#14455=CARTESIAN_POINT('Ctrl Pts',(-2.84859095134652,-0.259146701410729,
-0.136386777026674));
#14456=CARTESIAN_POINT('Ctrl Pts',(-2.84069830829409,-0.267160119774128,
-0.25591825162007));
#14457=CARTESIAN_POINT('Ctrl Pts',(-2.82499127124688,-0.275174317819118,
-0.374425444279389));
#14458=CARTESIAN_POINT('Ctrl Pts',(-2.80820184658356,-0.283740782258516,
-0.501099085987492));
#14459=CARTESIAN_POINT('Ctrl Pts',(-2.78248344796085,-0.292308137539294,
-0.62660131446913));
#14460=CARTESIAN_POINT('Ctrl Pts',(-2.74843102357668,-0.300875715037838,
-0.749793091323411));
#14461=CARTESIAN_POINT('Ctrl Pts',(-2.7192635507982,-0.308214240502195,
-0.85531253268221));
#14462=CARTESIAN_POINT('Ctrl Pts',(-2.68398275963749,-0.315552929001334,
-0.959136584134086));
#14463=CARTESIAN_POINT('Ctrl Pts',(-2.64299019944675,-0.322891360356581,
-1.06056200859463));
#14464=CARTESIAN_POINT('Ctrl Pts',(-2.58928984766141,-0.332504722964227,
-1.19342955695376));
#14465=CARTESIAN_POINT('Ctrl Pts',(-2.52573563654052,-0.34211651623184,
-1.32233107103795));
#14466=CARTESIAN_POINT('Ctrl Pts',(-2.45307990206561,-0.35172744735852,
-1.44588164571447));
#14467=CARTESIAN_POINT('Ctrl Pts',(-2.38190226984351,-0.361142854497278,
-1.56691871771862));
#14468=CARTESIAN_POINT('Ctrl Pts',(-2.30198893075688,-0.370557434216932,
-1.6828213822311));
#14469=CARTESIAN_POINT('Ctrl Pts',(-2.21400728279147,-0.379971851427205,
-1.79225939560688));
#14470=CARTESIAN_POINT('Ctrl Pts',(-2.1683256449433,-0.384859984435583,
-1.84908156033628));
#14471=CARTESIAN_POINT('Ctrl Pts',(-2.12046830077378,-0.389748073633526,
-1.90416037877037));
#14472=CARTESIAN_POINT('Ctrl Pts',(-2.07052526111232,-0.394636212091378,
-1.95730518181801));
#14473=CARTESIAN_POINT('Ctrl Pts',(-2.00881800212756,-0.400675764906277,
-2.02296838829451));
#14474=CARTESIAN_POINT('Ctrl Pts',(-1.94394844543176,-0.406716201619121,
-2.08565406472235));
#14475=CARTESIAN_POINT('Ctrl Pts',(-1.8761293000041,-0.412757196014427,
-2.14497294477118));
#14476=CARTESIAN_POINT('Ctrl Pts',(-1.77418651530985,-0.421837755598251,
-2.23413850088353));
#14477=CARTESIAN_POINT('Ctrl Pts',(-1.66557812957501,-0.430919575254045,
-2.31569450072344));
#14478=CARTESIAN_POINT('Ctrl Pts',(-1.55171138002138,-0.440001547039586,
-2.38910295251116));
#14479=CARTESIAN_POINT('Ctrl Pts',(-1.44140473304468,-0.448799566299178,
-2.46021625124145));
#14480=CARTESIAN_POINT('Ctrl Pts',(-1.3261645781001,-0.457597728324383,
-2.52368334697871));
#14481=CARTESIAN_POINT('Ctrl Pts',(-1.20728772228421,-0.466395025878857,
-2.57905840053748));
#14482=CARTESIAN_POINT('Ctrl Pts',(-1.06924625101902,-0.476610571110452,
-2.64336068891968));
#14483=CARTESIAN_POINT('Ctrl Pts',(-0.926118773149324,-0.486824213024927,
-2.69684664251162));
#14484=CARTESIAN_POINT('Ctrl Pts',(-0.77969440642078,-0.497037072922188,
-2.73883496415487));
#14485=CARTESIAN_POINT('Ctrl Pts',(-0.638052790054798,-0.506916343810545,
-2.7794517950753));
#14486=CARTESIAN_POINT('Ctrl Pts',(-0.49332491118727,-0.516794882934398,
-2.80931002663451));
#14487=CARTESIAN_POINT('Ctrl Pts',(-0.347125828863604,-0.526673705266467,
-2.82774527917647));
#14488=CARTESIAN_POINT('Ctrl Pts',(-0.290572441659506,-0.530495075794835,
-2.83487648655917));
#14489=CARTESIAN_POINT('Ctrl Pts',(-0.23379896130483,-0.53431648870055,
-2.84029790415576));
#14490=CARTESIAN_POINT('Ctrl Pts',(-0.176899268891918,-0.538138002732039,
-2.84396897512448));
#14491=CARTESIAN_POINT('Ctrl Pts',(-0.116352231391689,-0.542204480836932,
-2.84787536656851));
#14492=CARTESIAN_POINT('Ctrl Pts',(-0.0556864187648436,-0.546271383042092,
-2.84979803401917));
#14493=CARTESIAN_POINT('Ctrl Pts',(0.00497365610244438,-0.550338591071923,
-2.8496921406586));
#14494=CARTESIAN_POINT('Ctrl Pts',(0.154530000355481,-0.560366220704572,
-2.84943106244659));
#14495=CARTESIAN_POINT('Ctrl Pts',(0.304050612630736,-0.570395709324061,
-2.83683559990313));
#14496=CARTESIAN_POINT('Ctrl Pts',(0.451675731743237,-0.5804252843707,-2.81261256222691));
#14497=CARTESIAN_POINT('Ctrl Pts',(0.596287470173571,-0.590250131875864,
-2.78888397450767));
#14498=CARTESIAN_POINT('Ctrl Pts',(0.739079140294107,-0.600075062315811,
-2.75399829388592));
#14499=CARTESIAN_POINT('Ctrl Pts',(0.878322966205294,-0.609898409476766,
-2.70866393343392));
#14500=CARTESIAN_POINT('Ctrl Pts',(1.04784464245577,-0.621857792711305,
-2.65347185058733));
#14501=CARTESIAN_POINT('Ctrl Pts',(1.21239860104531,-0.633814470368098,
-2.58270958152775));
#14502=CARTESIAN_POINT('Ctrl Pts',(1.36904374063119,-0.645770674535305,
-2.49743826863348));
#14503=CARTESIAN_POINT('Ctrl Pts',(1.51022988132689,-0.656546944569603,
-2.42058221289232));
#14504=CARTESIAN_POINT('Ctrl Pts',(1.64499180429864,-0.667322829958374,
-2.33193849640115));
#14505=CARTESIAN_POINT('Ctrl Pts',(1.7711385373037,-0.678099965020317,-2.23225318102518));
#14506=CARTESIAN_POINT('Ctrl Pts',(1.78495081516552,-0.67927999386834,-2.22133826280323));
#14507=CARTESIAN_POINT('Ctrl Pts',(1.79865976111333,-0.680460037698545,
-2.21029094308228));
#14508=CARTESIAN_POINT('Ctrl Pts',(1.81226246383145,-0.681640098656313,
-2.19911218332638));
#14509=CARTESIAN_POINT('Ctrl Pts',(1.83638940132602,-0.683733157481302,
-2.17928456204503));
#14510=CARTESIAN_POINT('Ctrl Pts',(1.86017575754718,-0.685826322908651,
-2.15904864358979));
#14511=CARTESIAN_POINT('Ctrl Pts',(1.88360520990837,-0.687919577979938,
-2.13841094879892));
#14512=CARTESIAN_POINT('Ctrl Pts',(2.01767668833799,-0.699897911822797,
-2.0203148785478));
#14513=CARTESIAN_POINT('Ctrl Pts',(2.14005752488522,-0.711879181080226,
-1.8890612688117));
#14514=CARTESIAN_POINT('Ctrl Pts',(2.24922740729515,-0.7238602080859,-1.74760001821103));
#14515=CARTESIAN_POINT('Ctrl Pts',(2.33895996050149,-0.733708053659428,
-1.63132546596324));
#14516=CARTESIAN_POINT('Ctrl Pts',(2.41976767616667,-0.743555735565897,
-1.50815535967203));
#14517=CARTESIAN_POINT('Ctrl Pts',(2.49083272407377,-0.753401489190834,
-1.37973020927764));
#14518=CARTESIAN_POINT('Ctrl Pts',(2.58692232024631,-0.766714285251585,
-1.20608196441995));
#14519=CARTESIAN_POINT('Ctrl Pts',(2.66539065768445,-0.780023697310082,
-1.02249109650153));
#14520=CARTESIAN_POINT('Ctrl Pts',(2.72408373297952,-0.793333409033395,
-0.832806588169003));
#14521=CARTESIAN_POINT('Ctrl Pts',(2.77083752169619,-0.803935672531488,
-0.681707512497436));
#14522=CARTESIAN_POINT('Ctrl Pts',(2.80504246184954,-0.81453812617926,-0.526742078154303));
#14523=CARTESIAN_POINT('Ctrl Pts',(2.8255909834669,-0.825142631936016,-0.369870509681839));
#14524=CARTESIAN_POINT('Ctrl Pts',(2.82582273756608,-0.825262233614654,
-0.368101252033223));
#14525=CARTESIAN_POINT('Ctrl Pts',(2.82605275056068,-0.825381835575542,
-0.366331781103057));
#14526=CARTESIAN_POINT('Ctrl Pts',(2.82628102101889,-0.825501437815763,
-0.364562099745109));
#14527=CARTESIAN_POINT('Ctrl Pts',(2.85228039059975,-0.839123799949733,
-0.163000320674225));
#14528=CARTESIAN_POINT('Ctrl Pts',(2.85567668810618,-0.852749785743964,
0.0412871256586262));
#14529=CARTESIAN_POINT('Ctrl Pts',(2.83767946395795,-0.866375084534093,
0.243678475560316));
#14530=CARTESIAN_POINT('Ctrl Pts',(2.82423649436951,-0.876552458320218,
0.39485405348747));
#14531=CARTESIAN_POINT('Ctrl Pts',(2.79885689994874,-0.886729448806458,
0.544972862464313));
#14532=CARTESIAN_POINT('Ctrl Pts',(2.76203586844939,-0.896904259550461,
0.692125424989613));
#14533=CARTESIAN_POINT('Ctrl Pts',(2.71744107462166,-0.909227205673603,
0.870345260768906));
#14534=CARTESIAN_POINT('Ctrl Pts',(2.65597926441388,-0.921547418985483,
1.04453367619778));
#14535=CARTESIAN_POINT('Ctrl Pts',(2.57838960400743,-0.933868114421141,
1.21118089962741));
#14536=CARTESIAN_POINT('Ctrl Pts',(2.51706685619316,-0.943605737902665,
1.34289001657406));
#14537=CARTESIAN_POINT('Ctrl Pts',(2.44567101895833,-0.95334366254192,1.46988763932027));
#14538=CARTESIAN_POINT('Ctrl Pts',(2.36458933503997,-0.963083475516264,
1.59043615941138));
#14539=CARTESIAN_POINT('Ctrl Pts',(2.34915516664531,-0.964937481332544,
1.61338297142735));
#14540=CARTESIAN_POINT('Ctrl Pts',(2.33337009128119,-0.966791555571495,
1.63609610498031));
#14541=CARTESIAN_POINT('Ctrl Pts',(2.31724389399609,-0.968645709180412,
1.65856831625786));
#14542=CARTESIAN_POINT('Ctrl Pts',(2.22206520595145,-0.979589138980383,
1.79120191542856));
#14543=CARTESIAN_POINT('Ctrl Pts',(2.11514122746783,-0.990534146427008,
1.91525839371467));
#14544=CARTESIAN_POINT('Ctrl Pts',(1.99849993464102,-1.0014788962736,2.02939768246979));
#14545=CARTESIAN_POINT('Ctrl Pts',(1.87549830855913,-1.0130204524032,2.14976087269569));
#14546=CARTESIAN_POINT('Ctrl Pts',(1.74169002021321,-1.02456172207351,2.25909682066194));
#14547=CARTESIAN_POINT('Ctrl Pts',(1.59940027188827,-1.03610055314691,2.3558139759935));
#14548=CARTESIAN_POINT('Ctrl Pts',(1.58169941761635,-1.03753598450934,2.36784559662867));
#14549=CARTESIAN_POINT('Ctrl Pts',(1.56386725431272,-1.03897137813357,2.3796819008649));
#14550=CARTESIAN_POINT('Ctrl Pts',(1.54590821413885,-1.04040672987643,2.39131979215231));
#14551=CARTESIAN_POINT('Ctrl Pts',(1.41850062270793,-1.05058960750483,2.47388298505734));
#14552=CARTESIAN_POINT('Ctrl Pts',(1.2845210901381,-1.06077094234822,2.54657562083443));
#14553=CARTESIAN_POINT('Ctrl Pts',(1.14562765742176,-1.07095249073693,2.60814967754909));
#14554=CARTESIAN_POINT('Ctrl Pts',(1.01052845018237,-1.08085590437486,2.66804168313909));
#14555=CARTESIAN_POINT('Ctrl Pts',(0.870781356165271,-1.09075952005037,
2.71741367426934));
#14556=CARTESIAN_POINT('Ctrl Pts',(0.727942869331522,-1.10066495405409,
2.75515317742913));
#14557=CARTESIAN_POINT('Ctrl Pts',(0.672745192890889,-1.10449275252256,
2.76973701215477));
#14558=CARTESIAN_POINT('Ctrl Pts',(0.617086111586118,-1.10832082252452,
2.78258418807595));
#14559=CARTESIAN_POINT('Ctrl Pts',(0.561075206954555,-1.11214925733085,
2.79370443055281));
#14560=CARTESIAN_POINT('Ctrl Pts',(0.415939980854654,-1.12206948188143,
2.82251915719901));
#14561=CARTESIAN_POINT('Ctrl Pts',(0.268591246834638,-1.1319903866323,2.83971425995812));
#14562=CARTESIAN_POINT('Ctrl Pts',(0.12079118009236,-1.14191092298971,2.84554363412139));
#14563=CARTESIAN_POINT('Ctrl Pts',(-0.032618438032068,-1.15220797987016,
2.85159425428688));
#14564=CARTESIAN_POINT('Ctrl Pts',(-0.186515561471283,-1.16250463986278,
2.84540020170277));
#14565=CARTESIAN_POINT('Ctrl Pts',(-0.338946955042084,-1.17279973039116,
2.82719276804528));
#14566=CARTESIAN_POINT('Ctrl Pts',(-0.393778617605422,-1.17650301563108,
2.82064330447963));
#14567=CARTESIAN_POINT('Ctrl Pts',(-0.448420685577804,-1.18020609779181,
2.81253889014373));
#14568=CARTESIAN_POINT('Ctrl Pts',(-0.502782257634685,-1.18390892229605,
2.80288865320055));
#14569=CARTESIAN_POINT('Ctrl Pts',(-0.637274623859498,-1.19306983524332,
2.77901364090767));
#14570=CARTESIAN_POINT('Ctrl Pts',(-0.770213396999383,-1.20222989352261,
2.74564308769741));
#14571=CARTESIAN_POINT('Ctrl Pts',(-0.900056879936483,-1.21139019744609,
2.70289282289534));
#14572=CARTESIAN_POINT('Ctrl Pts',(-1.02694447851203,-1.22034196722906,
2.66111576703933));
#14573=CARTESIAN_POINT('Ctrl Pts',(-1.15087493148394,-1.22929397159932,
2.61038149471995));
#14574=CARTESIAN_POINT('Ctrl Pts',(-1.27041542598044,-1.23824723742104,
2.55084583424531));
#14575=CARTESIAN_POINT('Ctrl Pts',(-1.34787274881595,-1.24404858535845,
2.51226917540653));
#14576=CARTESIAN_POINT('Ctrl Pts',(-1.42348713502069,-1.24985046291713,
2.46999825131315));
#14577=CARTESIAN_POINT('Ctrl Pts',(-1.49698933741267,-1.25565314945133,
2.42431798977058));
#14578=CARTESIAN_POINT('Ctrl Pts',(-1.61624974890631,-1.26506825214644,
2.35019984621277));
#14579=CARTESIAN_POINT('Ctrl Pts',(-1.72987865084394,-1.27448345518868,
2.26715757146334));
#14580=CARTESIAN_POINT('Ctrl Pts',(-1.8369037071566,-1.28389814149844,2.17633379704892));
#14581=CARTESIAN_POINT('Ctrl Pts',(-1.94676850078249,-1.29356263133018,
2.0831001602152));
#14582=CARTESIAN_POINT('Ctrl Pts',(-2.04967536339833,-1.30322657664433,
1.98166583179054));
#14583=CARTESIAN_POINT('Ctrl Pts',(-2.14454649169789,-1.31288930992677,
1.87321917481648));
#14584=CARTESIAN_POINT('Ctrl Pts',(-2.19207519461938,-1.31773016285876,
1.81888937991962));
#14585=CARTESIAN_POINT('Ctrl Pts',(-2.2375865690511,-1.32257071159175,1.76279894915519));
#14586=CARTESIAN_POINT('Ctrl Pts',(-2.2809414956653,-1.32741087219403,1.70509395756389));
#14587=CARTESIAN_POINT('Ctrl Pts',(-2.35806048512942,-1.33602046569683,
1.60244932208436));
#14588=CARTESIAN_POINT('Ctrl Pts',(-2.42843033480345,-1.34462973490771,
1.4945890168124));
#14589=CARTESIAN_POINT('Ctrl Pts',(-2.49113853055435,-1.35323935515332,
1.38244863236214));
#14590=CARTESIAN_POINT('Ctrl Pts',(-2.54598462287356,-1.3607695355575,1.28436796197092));
#14591=CARTESIAN_POINT('Ctrl Pts',(-2.5949698842659,-1.36829998449169,1.18301421805579));
#14592=CARTESIAN_POINT('Ctrl Pts',(-2.63750948583029,-1.37583115378905,
1.07903361952129));
#14593=CARTESIAN_POINT('Ctrl Pts',(-2.68142316890915,-1.38360558912872,
0.971694319610797));
#14594=CARTESIAN_POINT('Ctrl Pts',(-2.71846769641451,-1.39138079212042,
0.861556290119179));
#14595=CARTESIAN_POINT('Ctrl Pts',(-2.74861153842052,-1.39915725981108,
0.749579659818414));
#14596=CARTESIAN_POINT('Ctrl Pts',(-2.78412055464879,-1.40831782790891,
0.617672785381378));
#14597=CARTESIAN_POINT('Ctrl Pts',(-2.81005394236977,-1.41747805955768,
0.483246619510076));
#14598=CARTESIAN_POINT('Ctrl Pts',(-2.82643013810069,-1.42663764140704,
0.347667528530173));
#14599=CARTESIAN_POINT('Ctrl Pts',(-2.84308692979975,-1.43595416701665,
0.209765373823006));
#14600=CARTESIAN_POINT('Ctrl Pts',(-2.84985638294299,-1.44527002036825,
0.0706691911022305));
#14601=CARTESIAN_POINT('Ctrl Pts',(-2.84670661998034,-1.45458487172665,
-0.0681974790284871));
#14602=CARTESIAN_POINT('Ctrl Pts',(-2.84486611926434,-1.46002781800478,
-0.149341428219176));
#14603=CARTESIAN_POINT('Ctrl Pts',(-2.83963781638863,-1.46547042216091,
-0.230407182515753));
#14604=CARTESIAN_POINT('Ctrl Pts',(-2.8310071078325,-1.47091261840812,-0.311110263182307));
#14605=CARTESIAN_POINT('Ctrl Pts',(-2.81781371033578,-1.47923187260117,
-0.434477633951345));
#14606=CARTESIAN_POINT('Ctrl Pts',(-2.79665378128776,-1.48755127053128,
-0.557093791266127));
#14607=CARTESIAN_POINT('Ctrl Pts',(-2.76747059455719,-1.49587114828328,
-0.677766985411362));
#14608=CARTESIAN_POINT('Ctrl Pts',(-2.74695702916998,-1.50171939089827,
-0.762591082294128));
#14609=CARTESIAN_POINT('Ctrl Pts',(-2.72248022415427,-1.50756787059436,
-0.846454899621325));
#14610=CARTESIAN_POINT('Ctrl Pts',(-2.69403586235103,-1.51341670409936,
-0.928945999604021));
#14611=CARTESIAN_POINT('Ctrl Pts',(-2.65364415779899,-1.52172219383198,
-1.04608542293585));
#14612=CARTESIAN_POINT('Ctrl Pts',(-2.60525022569129,-1.53002839701002,
-1.16045536951902));
#14613=CARTESIAN_POINT('Ctrl Pts',(-2.54960516799807,-1.53833564787641,
-1.27114014825599));
#14614=CARTESIAN_POINT('Ctrl Pts',(-2.53994671480788,-1.53977755838847,
-1.29035198482539));
#14615=CARTESIAN_POINT('Ctrl Pts',(-2.53006991307008,-1.54121950046469,
-1.30945286158362));
#14616=CARTESIAN_POINT('Ctrl Pts',(-2.51997882226938,-1.5426614758529,-1.32843807863483));
#14617=CARTESIAN_POINT('Ctrl Pts',(-2.45657270677688,-1.55172194907707,
-1.44772933156009));
#14618=CARTESIAN_POINT('Ctrl Pts',(-2.38470081591898,-1.56078173197691,
-1.56247422468651));
#14619=CARTESIAN_POINT('Ctrl Pts',(-2.3052368403023,-1.56984075937861,-1.67169370439398));
#14620=CARTESIAN_POINT('Ctrl Pts',(-2.22510581752997,-1.57897583128243,
-1.78183000889803));
#14621=CARTESIAN_POINT('Ctrl Pts',(-2.13725395829225,-1.58811013495105,
-1.88634876066361));
#14622=CARTESIAN_POINT('Ctrl Pts',(-2.04253202532631,-1.59724360355553,
-1.98421985142671));
#14623=CARTESIAN_POINT('Ctrl Pts',(-1.98317053855799,-1.60296747614488,
-2.0455548904976));
#14624=CARTESIAN_POINT('Ctrl Pts',(-1.92111002239413,-1.60869102076865,
-2.10427853314291));
#14625=CARTESIAN_POINT('Ctrl Pts',(-1.85655299640856,-1.61441422097834,
-2.16012933435915));
#14626=CARTESIAN_POINT('Ctrl Pts',(-1.76394106594421,-1.62262458401413,
-2.2402515277169));
#14627=CARTESIAN_POINT('Ctrl Pts',(-1.66613907414915,-1.63083553082874,
-2.31449904720288));
#14628=CARTESIAN_POINT('Ctrl Pts',(-1.56387127587846,-1.63904709023554,
-2.38197566886126));
#14629=CARTESIAN_POINT('Ctrl Pts',(-1.51423913488985,-1.64303228675983,
-2.41472311484342));
#14630=CARTESIAN_POINT('Ctrl Pts',(-1.46355574560736,-1.64701762756862,
-2.44587630950781));
#14631=CARTESIAN_POINT('Ctrl Pts',(-1.41190681906569,-1.65100311595549,
-2.47533616148238));
#14632=CARTESIAN_POINT('Ctrl Pts',(-1.30550422906709,-1.65921366969139,
-2.53602676554636));
#14633=CARTESIAN_POINT('Ctrl Pts',(-1.1950027195626,-1.66742484975796,-2.58952751654282));
#14634=CARTESIAN_POINT('Ctrl Pts',(-1.08153463719784,-1.67563668495174,
-2.63564802546423));
#14635=CARTESIAN_POINT('Ctrl Pts',(-1.03304098215896,-1.67914623490468,
-2.65535887280774));
#14636=CARTESIAN_POINT('Ctrl Pts',(-0.984005717021573,-1.68265590451736,
-2.67372232411164));
#14637=CARTESIAN_POINT('Ctrl Pts',(-0.934517956492218,-1.68616569603766,
-2.69072631614391));
#14638=CARTESIAN_POINT('Ctrl Pts',(-0.806271691038139,-1.69526123097774,
-2.73479172651251));
#14639=CARTESIAN_POINT('Ctrl Pts',(-0.674924695864088,-1.7043557744404,
-2.7697542564575));
#14640=CARTESIAN_POINT('Ctrl Pts',(-0.541788878943015,-1.71344948581134,
-2.79544280040553));
#14641=CARTESIAN_POINT('Ctrl Pts',(-0.408659211874132,-1.72254277712265,
-2.82113015774013));
#14642=CARTESIAN_POINT('Ctrl Pts',(-0.273739637134264,-1.73163523641909,
-2.83754458164282));
#14643=CARTESIAN_POINT('Ctrl Pts',(-0.138329457050682,-1.74072702306423,
-2.84446539794242));
#14644=CARTESIAN_POINT('Ctrl Pts',(-0.0529910806746092,-1.74645686043817,
-2.84882704361663));
#14645=CARTESIAN_POINT('Ctrl Pts',(0.0325423380463692,-1.75218643064925,
-2.8494170305828));
#14646=CARTESIAN_POINT('Ctrl Pts',(0.117944702086942,-1.75791577358787,
-2.84616945617145));
#14647=CARTESIAN_POINT('Ctrl Pts',(0.241332803706742,-1.76619344548451,
-2.84147740758488));
#14648=CARTESIAN_POINT('Ctrl Pts',(0.364474224217159,-1.77447212945813,
-2.82876802081294));
#14649=CARTESIAN_POINT('Ctrl Pts',(0.486208475639264,-1.78275154654318,
-2.80785133344645));
#14650=CARTESIAN_POINT('Ctrl Pts',(0.514819391444495,-1.78469743853635,
-2.8029353334368));
#14651=CARTESIAN_POINT('Ctrl Pts',(0.543352572900193,-1.78664337102512,
-2.79756620469295));
#14652=CARTESIAN_POINT('Ctrl Pts',(0.571792972249852,-1.78858934038785,
-2.79174190249468));
#14653=CARTESIAN_POINT('Ctrl Pts',(0.692971647225559,-1.7968807144301,-2.76692575225826));
#14654=CARTESIAN_POINT('Ctrl Pts',(0.812464588866411,-1.80517275789546,
-2.73384222121513));
#14655=CARTESIAN_POINT('Ctrl Pts',(0.929267711739225,-1.8134651906415,-2.69310782065252));
#14656=CARTESIAN_POINT('Ctrl Pts',(1.00534859807176,-1.81886654993442,-2.66657506003102));
#14657=CARTESIAN_POINT('Ctrl Pts',(1.08028852426493,-1.8242680743874,-2.63679735865193));
#14658=CARTESIAN_POINT('Ctrl Pts',(1.15381545442221,-1.82966968658238,-2.603955633288));
#14659=CARTESIAN_POINT('Ctrl Pts',(1.27996989407616,-1.83893754746313,-2.54760717087168));
#14660=CARTESIAN_POINT('Ctrl Pts',(1.40206986362378,-1.84820414389981,-2.48219900974871));
#14661=CARTESIAN_POINT('Ctrl Pts',(1.51894129549226,-1.85746987740176,-2.40849865032819));
#14662=CARTESIAN_POINT('Ctrl Pts',(1.63470780780595,-1.8666480113084,-2.33549506484991));
#14663=CARTESIAN_POINT('Ctrl Pts',(1.74534520783587,-1.87582529851979,-2.25435458956647));
#14664=CARTESIAN_POINT('Ctrl Pts',(1.84968554364318,-1.88500212926488,-2.16578098172825));
#14665=CARTESIAN_POINT('Ctrl Pts',(1.91189974797703,-1.89047392709545,-2.11296788223038));
#14666=CARTESIAN_POINT('Ctrl Pts',(1.97187457949454,-1.89594556263917,-2.05751133736491));
#14667=CARTESIAN_POINT('Ctrl Pts',(2.02935554639636,-1.90141711862002,-1.99955491386437));
#14668=CARTESIAN_POINT('Ctrl Pts',(2.11603817247803,-1.90966835144954,-1.91215528824726));
#14669=CARTESIAN_POINT('Ctrl Pts',(2.19703442575146,-1.91792098236696,-1.81907843166739));
#14670=CARTESIAN_POINT('Ctrl Pts',(2.27137118380573,-1.92617442917523,-1.7209424871885));
#14671=CARTESIAN_POINT('Ctrl Pts',(2.34817371186233,-1.93470164500556,-1.61955134737449));
#14672=CARTESIAN_POINT('Ctrl Pts',(2.41786670209158,-1.94322973175108,-1.51276058838507));
#14673=CARTESIAN_POINT('Ctrl Pts',(2.48007992947221,-1.95175804733692,-1.40178648915373));
#14674=CARTESIAN_POINT('Ctrl Pts',(2.53215578122658,-1.95889671087941,-1.3088951381748));
#14675=CARTESIAN_POINT('Ctrl Pts',(2.57899153730472,-1.96603553476112,-1.21307363921052));
#14676=CARTESIAN_POINT('Ctrl Pts',(2.62039639755441,-1.97317414241128,-1.11504501496294));
#14677=CARTESIAN_POINT('Ctrl Pts',(2.67503572119203,-1.98259450251797,-0.985682961964462));
#14678=CARTESIAN_POINT('Ctrl Pts',(2.72028312241804,-1.99201334903906,-0.85234232372255));
#14679=CARTESIAN_POINT('Ctrl Pts',(2.75573316399703,-2.00143131453587,-0.716444766366111));
#14680=CARTESIAN_POINT('Ctrl Pts',(2.79050233332678,-2.01066839360589,-0.583157329376883));
#14681=CARTESIAN_POINT('Ctrl Pts',(2.81584707486254,-2.01990462516945,-0.447409014739265));
#14682=CARTESIAN_POINT('Ctrl Pts',(2.8313366954026,-2.02914060603565,-0.310532368306937));
#14683=CARTESIAN_POINT('Ctrl Pts',(2.84015746635835,-2.03440015849283,-0.232586136877494));
#14684=CARTESIAN_POINT('Ctrl Pts',(2.84578143549661,-2.03965962965174,-0.154273939294073));
#14685=CARTESIAN_POINT('Ctrl Pts',(2.84812148408046,-2.04491912972532,-0.0758428334344391));
#14686=CARTESIAN_POINT('Ctrl Pts',(2.85091497943733,-2.05119779809844,0.0177863892939412));
#14687=CARTESIAN_POINT('Ctrl Pts',(2.84902594284215,-2.05747737660946,0.111557393492299));
#14688=CARTESIAN_POINT('Ctrl Pts',(2.8423143279138,-2.06375753276342,0.204986229314948));
#14689=CARTESIAN_POINT('Ctrl Pts',(2.83287159820045,-2.07259323292689,0.336433467204058));
#14690=CARTESIAN_POINT('Ctrl Pts',(2.813880666638,-2.08143007649653,0.467202554864027));
#14691=CARTESIAN_POINT('Ctrl Pts',(2.78589826341793,-2.09026713750293,0.596029432374906));
#14692=CARTESIAN_POINT('Ctrl Pts',(2.75802274342066,-2.09907044395463,0.72436423521504));
#14693=CARTESIAN_POINT('Ctrl Pts',(2.72122485788936,-2.10787396618517,0.850770535434859));
#14694=CARTESIAN_POINT('Ctrl Pts',(2.67610312119081,-2.11667678879524,0.974016832256147));
#14695=CARTESIAN_POINT('Ctrl Pts',(-2.097235989958,2.319248086811,0.5776750355837));
#14696=CARTESIAN_POINT('Ctrl Pts',(-2.235952065827,2.2733869757,0.07406949825217));
#14697=CARTESIAN_POINT('Ctrl Pts',(-2.133884893527,2.181664753478,-1.034686203893));
#14698=CARTESIAN_POINT('Ctrl Pts',(-0.9210292495221,2.044081420145,-2.185735282405));
#14699=CARTESIAN_POINT('Ctrl Pts',(0.7496331376127,1.906498086811,-2.25015296747));
#14700=CARTESIAN_POINT('Ctrl Pts',(2.047765400978,1.768914753478,-1.196625791736));
#14701=CARTESIAN_POINT('Ctrl Pts',(2.328382246189,1.631331420145,0.4515392303455));
#14702=CARTESIAN_POINT('Ctrl Pts',(1.452032556261,1.493748086811,1.875325701807));
#14703=CARTESIAN_POINT('Ctrl Pts',(-0.1458254019403,1.356164753478,2.367273318177));
#14704=CARTESIAN_POINT('Ctrl Pts',(-1.671223522139,1.218581420145,1.682931733308));
#14705=CARTESIAN_POINT('Ctrl Pts',(-2.366197443666,1.080998086811,0.1623484463472));
#14706=CARTESIAN_POINT('Ctrl Pts',(-1.885417534126,0.9434147534781,-1.43890517495));
#14707=CARTESIAN_POINT('Ctrl Pts',(-0.4677813480371,0.8058314201447,-2.325172676827));
#14708=CARTESIAN_POINT('Ctrl Pts',(1.182293478365,0.6682480868114,-2.056071375655));
#14709=CARTESIAN_POINT('Ctrl Pts',(2.244891504223,0.5306647534781,-0.7653166040083));
#14710=CARTESIAN_POINT('Ctrl Pts',(2.192012109843,0.3930814201447,0.9057208622855));
#14711=CARTESIAN_POINT('Ctrl Pts',(1.049930850427,0.2554980868114,2.12670933121));
#14712=CARTESIAN_POINT('Ctrl Pts',(-0.6138567605814,0.1179147534781,2.290944619059));
#14713=CARTESIAN_POINT('Ctrl Pts',(-1.972621454292,-0.01966857985527,1.31681888208));
#14714=CARTESIAN_POINT('Ctrl Pts',(-2.35119860367,-0.1572519131886,-0.3116287794445));
#14715=CARTESIAN_POINT('Ctrl Pts',(-1.561474769393,-0.2948352465219,-1.785229373121));
#14716=CARTESIAN_POINT('Ctrl Pts',(0.004139500834496,-0.4324185798553,-2.371756782494));
#14717=CARTESIAN_POINT('Ctrl Pts',(1.56769686923,-0.5700019131886,-1.779767932299));
#14718=CARTESIAN_POINT('Ctrl Pts',(2.352272068769,-0.7075852465219,-0.3034196680806));
#14719=CARTESIAN_POINT('Ctrl Pts',(1.968012873411,-0.8451685798553,1.323696600635));
#14720=CARTESIAN_POINT('Ctrl Pts',(0.6058561589209,-0.9827519131886,2.293073394949));
#14721=CARTESIAN_POINT('Ctrl Pts',(-1.057348156491,-1.120335246522,2.123031532212));
#14722=CARTESIAN_POINT('Ctrl Pts',(-2.195159931747,-1.257918579855,0.8980634200042));
#14723=CARTESIAN_POINT('Ctrl Pts',(-2.242207790093,-1.395501913189,-0.7731466788102));
#14724=CARTESIAN_POINT('Ctrl Pts',(-1.175103962369,-1.533085246522,-2.060191034956));
#14725=CARTESIAN_POINT('Ctrl Pts',(0.4758751430437,-1.670668579855,-2.323506201036));
#14726=CARTESIAN_POINT('Ctrl Pts',(1.890502368917,-1.808251913189,-1.43238765575));
#14727=CARTESIAN_POINT('Ctrl Pts',(2.365341628493,-1.945835246522,0.1708779092467));
#14728=CARTESIAN_POINT('Ctrl Pts',(1.899356541525,-2.037557468744,1.182122100046));
#14729=CARTESIAN_POINT('Ctrl Pts',(1.527422127243,-2.083418579855,1.548899250927));
#14730=CARTESIAN_POINT('Ctrl Pts',(-2.081620410866,2.281336533461,0.5733737884892));
#14731=CARTESIAN_POINT('Ctrl Pts',(-2.219303635942,2.23547542235,0.07351799231108));
#14732=CARTESIAN_POINT('Ctrl Pts',(-2.117996434389,2.143753200128,-1.02698214754));
#14733=CARTESIAN_POINT('Ctrl Pts',(-0.9141714590009,2.006169866795,-2.169460756152));
#14734=CARTESIAN_POINT('Ctrl Pts',(0.7440515265746,1.868586533461,-2.233398800651));
#14735=CARTESIAN_POINT('Ctrl Pts',(2.03251816951,1.731003200128,-1.187715967194));
#14736=CARTESIAN_POINT('Ctrl Pts',(2.311045600577,1.593419866795,0.4481771639882));
#14737=CARTESIAN_POINT('Ctrl Pts',(1.441221026544,1.455836533461,1.861362420153));
#14738=CARTESIAN_POINT('Ctrl Pts',(-0.1447396165978,1.318253200128,2.349647097803));
#14739=CARTESIAN_POINT('Ctrl Pts',(-1.658779942486,1.180669866795,1.670400976771));
#14740=CARTESIAN_POINT('Ctrl Pts',(-2.348579234028,1.043086533461,0.1611396338832));
#14741=CARTESIAN_POINT('Ctrl Pts',(-1.871379110807,0.905503200128,-1.42819138896));
#14742=CARTESIAN_POINT('Ctrl Pts',(-0.4642983462798,0.7679198667947,-2.307859928994));
#14743=CARTESIAN_POINT('Ctrl Pts',(1.17349036922,0.6303365334613,-2.040762299642));
#14744=CARTESIAN_POINT('Ctrl Pts',(2.228176513155,0.492753200128,-0.7596182171705));
#14745=CARTESIAN_POINT('Ctrl Pts',(2.175690847649,0.3551698667947,0.8989770548032));
#14746=CARTESIAN_POINT('Ctrl Pts',(1.042113285635,0.2175865334613,2.110874299803));
#14747=CARTESIAN_POINT('Ctrl Pts',(-0.609286111955,0.080003200128,2.273886726162));
#14748=CARTESIAN_POINT('Ctrl Pts',(-1.957933728882,-0.05758013320533,1.307014125008));
#14749=CARTESIAN_POINT('Ctrl Pts',(-2.333692072247,-0.1951634665387,-0.3093084569456));
#14750=CARTESIAN_POINT('Ctrl Pts',(-1.549848355923,-0.332746799872,-1.771936929824));
#14751=CARTESIAN_POINT('Ctrl Pts',(0.004108678979924,-0.4703301332053,-2.354097179186));
#14752=CARTESIAN_POINT('Ctrl Pts',(1.556024127311,-0.6079134665387,-1.766516153745));
#14753=CARTESIAN_POINT('Ctrl Pts',(2.33475754455,-0.745496799872,-0.3011604689023));
#14754=CARTESIAN_POINT('Ctrl Pts',(1.953359462527,-0.8830801332053,1.313840633513));
#14755=CARTESIAN_POINT('Ctrl Pts',(0.6013450810956,-1.020663466539,2.275999651633));
#14756=CARTESIAN_POINT('Ctrl Pts',(-1.049475363994,-1.158246799872,2.107223884925));
#14757=CARTESIAN_POINT('Ctrl Pts',(-2.178815231532,-1.295830133205,0.8913766282303));
#14758=CARTESIAN_POINT('Ctrl Pts',(-2.225512781398,-1.433413466539,-0.7673899908785));
#14759=CARTESIAN_POINT('Ctrl Pts',(-1.166354384852,-1.570996799872,-2.044851284825));
#14760=CARTESIAN_POINT('Ctrl Pts',(0.4723318765873,-1.708580133205,-2.306205861433));
#14761=CARTESIAN_POINT('Ctrl Pts',(1.876426084985,-1.846163466539,-1.42172239784));
#14762=CARTESIAN_POINT('Ctrl Pts',(2.347729791075,-1.983746799872,0.1696055881918));
#14763=CARTESIAN_POINT('Ctrl Pts',(1.885214331281,-2.075469022094,1.173320266948));
#14764=CARTESIAN_POINT('Ctrl Pts',(1.516049262601,-2.121330133205,1.537366472129));
#14765=CARTESIAN_POINT('Ctrl Pts',(-2.053521584663,2.153834933397,0.5656340822739));
#14766=CARTESIAN_POINT('Ctrl Pts',(-2.189346287892,2.107973822286,0.07252560711062));
#14767=CARTESIAN_POINT('Ctrl Pts',(-2.089406585155,2.016251600064,-1.013119392963));
#14768=CARTESIAN_POINT('Ctrl Pts',(-0.9018314834646,1.878668266731,-2.140176213964));
#14769=CARTESIAN_POINT('Ctrl Pts',(0.7340079209191,1.741084933397,-2.203251188525));
#14770=CARTESIAN_POINT('Ctrl Pts',(2.005082151636,1.603501600064,-1.171683541509));
#14771=CARTESIAN_POINT('Ctrl Pts',(2.279849870396,1.465918266731,0.4421274288044));
#14772=CARTESIAN_POINT('Ctrl Pts',(1.421766653915,1.328334933397,1.836236754172));
#14773=CARTESIAN_POINT('Ctrl Pts',(-0.1427858438013,1.190751600064,2.317930303956));
#14774=CARTESIAN_POINT('Ctrl Pts',(-1.636388843192,1.053168266731,1.647853010538));
#14775=CARTESIAN_POINT('Ctrl Pts',(-2.316876854778,0.9155849333973,0.1589644848776));
#14776=CARTESIAN_POINT('Ctrl Pts',(-1.846118234175,0.778001600064,-1.408912897352));
#14777=CARTESIAN_POINT('Ctrl Pts',(-0.4580309987508,0.6404182667307,-2.276707200713));
#14778=CARTESIAN_POINT('Ctrl Pts',(1.15764996827,0.5028349333973,-2.013214998089));
#14779=CARTESIAN_POINT('Ctrl Pts',(2.19809939426,0.365251600064,-0.7493644839955));
#14780=CARTESIAN_POINT('Ctrl Pts',(2.146322208353,0.2276682667307,0.8868421814655));
#14781=CARTESIAN_POINT('Ctrl Pts',(1.02804628286,0.09008493339734,2.082380588953));
#14782=CARTESIAN_POINT('Ctrl Pts',(-0.6010616419805,-0.047498399936,2.243192586352));
#14783=CARTESIAN_POINT('Ctrl Pts',(-1.931504491699,-0.1850817332693,1.289371348951));
#14784=CARTESIAN_POINT('Ctrl Pts',(-2.302190647873,-0.3226650666027,-0.3051332458796));
#14785=CARTESIAN_POINT('Ctrl Pts',(-1.528927673474,-0.460248399936,-1.748018376964));
#14786=CARTESIAN_POINT('Ctrl Pts',(0.004053217832441,-0.5978317332693,-2.32232031576));
#14787=CARTESIAN_POINT('Ctrl Pts',(1.535020080995,-0.7354150666027,-1.742670773421));
#14788=CARTESIAN_POINT('Ctrl Pts',(2.303241737861,-0.872998399936,-0.297095243739));
#14789=CARTESIAN_POINT('Ctrl Pts',(1.926991971239,-1.010581733269,1.296105709592));
#14790=CARTESIAN_POINT('Ctrl Pts',(0.593227803405,-1.148165066603,2.245276990425));
#14791=CARTESIAN_POINT('Ctrl Pts',(-1.035308983945,-1.285748399936,2.078779449328));
#14792=CARTESIAN_POINT('Ctrl Pts',(-2.14940441763,-1.423331733269,0.8793443495176));
#14793=CARTESIAN_POINT('Ctrl Pts',(-2.195471618979,-1.560915066603,-0.7570313501432));
#14794=CARTESIAN_POINT('Ctrl Pts',(-1.150610309237,-1.698498399936,-2.017248787961));
#14795=CARTESIAN_POINT('Ctrl Pts',(0.4659560881674,-1.836081733269,-2.27507546064));
#14796=CARTESIAN_POINT('Ctrl Pts',(1.851097081595,-1.973665066603,-1.402531228136));
#14797=CARTESIAN_POINT('Ctrl Pts',(2.316038878061,-2.111248399936,0.1673161612047));
#14798=CARTESIAN_POINT('Ctrl Pts',(1.85976669944,-2.202970622158,1.157482162128));
#14799=CARTESIAN_POINT('Ctrl Pts',(1.495584818401,-2.248831733269,1.516614276827));
#14800=CARTESIAN_POINT('Ctrl Pts',(-2.157170361559,1.938833333333,0.5941837119619));
#14801=CARTESIAN_POINT('Ctrl Pts',(-2.299850636439,1.892972222222,0.07618624088569));
#14802=CARTESIAN_POINT('Ctrl Pts',(-2.19486660983,1.80125,-1.064255249881));
#14803=CARTESIAN_POINT('Ctrl Pts',(-0.9473502308328,1.663666666667,-2.24819876828));
#14804=CARTESIAN_POINT('Ctrl Pts',(0.7710559966752,1.526083333333,-2.31445736848));
#14805=CARTESIAN_POINT('Ctrl Pts',(2.10628601243,1.3885,-1.230822713405));
#14806=CARTESIAN_POINT('Ctrl Pts',(2.394922267169,1.250916666667,0.4644432240559));
#14807=CARTESIAN_POINT('Ctrl Pts',(1.493528439041,1.113333333333,1.928918367593));
#14808=CARTESIAN_POINT('Ctrl Pts',(-0.1499927697857,0.97575,2.434924760079));
#14809=CARTESIAN_POINT('Ctrl Pts',(-1.718983398511,0.8381666666667,1.73102620449));
#14810=CARTESIAN_POINT('Ctrl Pts',(-2.433818139452,0.7005833333333,0.1669880063007));
#14811=CARTESIAN_POINT('Ctrl Pts',(-1.939298602186,0.563,-1.480025906173));
#14812=CARTESIAN_POINT('Ctrl Pts',(-0.4811495055907,0.4254166666667,-2.391620975404));
#14813=CARTESIAN_POINT('Ctrl Pts',(1.216080814179,0.2878333333333,-2.114829353515));
#14814=CARTESIAN_POINT('Ctrl Pts',(2.309045544236,0.15025,-0.7871876618941));
#14815=CARTESIAN_POINT('Ctrl Pts',(2.25465497358,0.01266666666667,0.9316043637066));
#14816=CARTESIAN_POINT('Ctrl Pts',(1.079935554736,-0.1249166666667,2.187485985794));
#14817=CARTESIAN_POINT('Ctrl Pts',(-0.6313994307312,-0.2625,2.356414755359));
#14818=CARTESIAN_POINT('Ctrl Pts',(-2.028994617748,-0.4000833333333,1.354450656752));
#14819=CARTESIAN_POINT('Ctrl Pts',(-2.418390665742,-0.5376666666667,-0.3205344415436));
#14820=CARTESIAN_POINT('Ctrl Pts',(-1.606098268856,-0.67525,-1.836247284864));
#14821=CARTESIAN_POINT('Ctrl Pts',(0.004257798623803,-0.8128333333333,-2.439536351903));
#14822=CARTESIAN_POINT('Ctrl Pts',(1.612498182562,-0.9504166666667,-1.830629768129));
#14823=CARTESIAN_POINT('Ctrl Pts',(2.419494808103,-1.088,-0.3120907319116));
#14824=CARTESIAN_POINT('Ctrl Pts',(2.024254333806,-1.225583333333,1.36152492531));
#14825=CARTESIAN_POINT('Ctrl Pts',(0.6231701895493,-1.363166666667,2.358604366961));
#14826=CARTESIAN_POINT('Ctrl Pts',(-1.087564831021,-1.50075,2.183703083425));
#14827=CARTESIAN_POINT('Ctrl Pts',(-2.25789275328,-1.638333333333,0.9237280886409));
#14828=CARTESIAN_POINT('Ctrl Pts',(-2.306285135485,-1.775916666667,-0.7952415029365));
#14829=CARTESIAN_POINT('Ctrl Pts',(-1.208685837698,-1.9135,-2.119066743579));
#14830=CARTESIAN_POINT('Ctrl Pts',(0.4894746033787,-2.051083333333,-2.389906875417));
#14831=CARTESIAN_POINT('Ctrl Pts',(1.944528750322,-2.188666666667,-1.473322130671));
#14832=CARTESIAN_POINT('Ctrl Pts',(2.432937866972,-2.32625,0.1757612224075));
#14833=CARTESIAN_POINT('Ctrl Pts',(1.953635955623,-2.417972222222,1.215904538245));
#14834=CARTESIAN_POINT('Ctrl Pts',(1.57107247742,-2.463833333333,1.593163369853));
#14835=CARTESIAN_POINT('Ctrl Pts',(-2.37767976724,1.824458133325,0.6549221216513));
#14836=CARTESIAN_POINT('Ctrl Pts',(-2.534945048097,1.778597022214,0.08397412032173));
#14837=CARTESIAN_POINT('Ctrl Pts',(-2.419229386322,1.686874799992,-1.173045124258));
#14838=CARTESIAN_POINT('Ctrl Pts',(-1.044189887123,1.549291466659,-2.478013243336));
#14839=CARTESIAN_POINT('Ctrl Pts',(0.8498745742914,1.411708133325,-2.551044903657));
#14840=CARTESIAN_POINT('Ctrl Pts',(2.321593938533,1.274124799992,-1.3566393804));
#14841=CARTESIAN_POINT('Ctrl Pts',(2.639735053028,1.136541466659,0.5119193534958));
#14842=CARTESIAN_POINT('Ctrl Pts',(1.646199305622,0.9989581333253,2.126095489263));
#14843=CARTESIAN_POINT('Ctrl Pts',(-0.1653252706912,0.861374799992,2.683826664765));
#14844=CARTESIAN_POINT('Ctrl Pts',(-1.894700631761,0.7237914666587,1.907974472635));
#14845=CARTESIAN_POINT('Ctrl Pts',(-2.682606923607,0.5862081333253,0.184057787474));
#14846=CARTESIAN_POINT('Ctrl Pts',(-2.137536808044,0.448624799992,-1.63131652224));
#14847=CARTESIAN_POINT('Ctrl Pts',(-0.530333377858,0.3110414666587,-2.636096297938));
#14848=CARTESIAN_POINT('Ctrl Pts',(1.340390540649,0.1734581333253,-2.331010593612));
#14849=CARTESIAN_POINT('Ctrl Pts',(2.54507987408,0.035874799992,-0.8676552441385));
#14850=CARTESIAN_POINT('Ctrl Pts',(2.485129412271,-0.1017085333413,1.026834452267));
#14851=CARTESIAN_POINT('Ctrl Pts',(1.190328294963,-0.2392918666747,2.411094303088));
#14852=CARTESIAN_POINT('Ctrl Pts',(-0.6959420907358,-0.376875200008,2.597291241752));
#14853=CARTESIAN_POINT('Ctrl Pts',(-2.236401693825,-0.5144585333413,1.492904769912));
#14854=CARTESIAN_POINT('Ctrl Pts',(-2.665602428852,-0.6520418666747,-0.3532999849911));
#14855=CARTESIAN_POINT('Ctrl Pts',(-1.770276203545,-0.789625200008,-2.023951420191));
#14856=CARTESIAN_POINT('Ctrl Pts',(0.004693037611301,-0.9272085333413,-2.688909660883));
#14857=CARTESIAN_POINT('Ctrl Pts',(1.777330326669,-1.064791866675,-2.017759671907));
#14858=CARTESIAN_POINT('Ctrl Pts',(2.666819438411,-1.202375200008,-0.3439931458512));
#14859=CARTESIAN_POINT('Ctrl Pts',(2.231176850475,-1.339958533341,1.50070218152));
#14860=CARTESIAN_POINT('Ctrl Pts',(0.6868716433541,-1.477541866675,2.599704678955));
#14861=CARTESIAN_POINT('Ctrl Pts',(-1.198737448077,-1.615125200008,2.406924706386));
#14862=CARTESIAN_POINT('Ctrl Pts',(-2.488698162992,-1.752708533341,1.018153051763));
#14863=CARTESIAN_POINT('Ctrl Pts',(-2.542037291931,-1.890291866675,-0.8765323616979));
#14864=CARTESIAN_POINT('Ctrl Pts',(-1.332239637841,-2.027875200008,-2.335681136467));
#14865=CARTESIAN_POINT('Ctrl Pts',(0.5395094804615,-2.165458533341,-2.634206979907));
#14866=CARTESIAN_POINT('Ctrl Pts',(2.143301590291,-2.303041866675,-1.623927476082));
#14867=CARTESIAN_POINT('Ctrl Pts',(2.681636668265,-2.440625200008,0.1937278157678));
#14868=CARTESIAN_POINT('Ctrl Pts',(2.153339748689,-2.53234742223,1.340196245508));
#14869=CARTESIAN_POINT('Ctrl Pts',(1.731670019669,-2.578208533341,1.756019078471));
#14870=CARTESIAN_POINT('Ctrl Pts',(-2.565745420624,1.884351681926,0.7067240330865));
#14871=CARTESIAN_POINT('Ctrl Pts',(-2.735449802072,1.838490570815,0.09061616187131));
#14872=CARTESIAN_POINT('Ctrl Pts',(-2.610581460513,1.746768348593,-1.26582864405));
#14873=CARTESIAN_POINT('Ctrl Pts',(-1.12678143544,1.60918501526,-2.674014902652));
#14874=CARTESIAN_POINT('Ctrl Pts',(0.9170965018656,1.471601681926,-2.75282309651));
#14875=CARTESIAN_POINT('Ctrl Pts',(2.505223410826,1.334018348593,-1.463944525103));
#14876=CARTESIAN_POINT('Ctrl Pts',(2.848528307842,1.19643501526,0.5524102762102));
#14877=CARTESIAN_POINT('Ctrl Pts',(1.77640756675,1.058851681926,2.294261759109));
#14878=CARTESIAN_POINT('Ctrl Pts',(-0.1784018865929,0.9212683485929,2.89610740258));
#14879=CARTESIAN_POINT('Ctrl Pts',(-2.044564426368,0.7836850152596,2.058888178837));
#14880=CARTESIAN_POINT('Ctrl Pts',(-2.894791184419,0.6461016819263,0.1986160759949));
#14881=CARTESIAN_POINT('Ctrl Pts',(-2.306608043782,0.5085183485929,-1.760347610387));
#14882=CARTESIAN_POINT('Ctrl Pts',(-0.5722807816221,0.3709350152596,-2.844601740716));
#14883=CARTESIAN_POINT('Ctrl Pts',(1.446410462377,0.2333516819263,-2.515384888406));
#14884=CARTESIAN_POINT('Ctrl Pts',(2.746386255211,0.09576834859292,-0.9362835567687));
#14885=CARTESIAN_POINT('Ctrl Pts',(2.681693934163,-0.04181498474041,1.108053250039));
#14886=CARTESIAN_POINT('Ctrl Pts',(1.284478849473,-0.1793983180737,2.601802922359));
#14887=CARTESIAN_POINT('Ctrl Pts',(-0.7509885296274,-0.3169816514071,2.802727348471));
#14888=CARTESIAN_POINT('Ctrl Pts',(-2.413292775447,-0.4545649847404,1.610988001667));
#14889=CARTESIAN_POINT('Ctrl Pts',(-2.87644169718,-0.5921483180737,-0.3812447038019));
#14890=CARTESIAN_POINT('Ctrl Pts',(-1.910298487233,-0.7297316514071,-2.184038472913));
#14891=CARTESIAN_POINT('Ctrl Pts',(0.005064239485027,-0.8673149847404,-2.901592444844));
#14892=CARTESIAN_POINT('Ctrl Pts',(1.91791056534,-1.004898318074,-2.177356980299));
#14893=CARTESIAN_POINT('Ctrl Pts',(2.877754967682,-1.142481651407,-0.3712017281949));
#14894=CARTESIAN_POINT('Ctrl Pts',(2.407654666361,-1.28006498474,1.619402159621));
#14895=CARTESIAN_POINT('Ctrl Pts',(0.7412006434902,-1.417648318074,2.805331679608));
#14896=CARTESIAN_POINT('Ctrl Pts',(-1.293553135418,-1.555231651407,2.597303526019));
#14897=CARTESIAN_POINT('Ctrl Pts',(-2.685544959835,-1.69281498474,1.098685182945));
#14898=CARTESIAN_POINT('Ctrl Pts',(-2.743103016096,-1.830398318074,-0.9458628214115));
#14899=CARTESIAN_POINT('Ctrl Pts',(-1.43761485338,-1.967981651407,-2.520424853883));
#14900=CARTESIAN_POINT('Ctrl Pts',(0.5821826799174,-2.10556498474,-2.842562984635));
#14901=CARTESIAN_POINT('Ctrl Pts',(2.31282879893,-2.243148318074,-1.752374118075));
#14902=CARTESIAN_POINT('Ctrl Pts',(2.893744185478,-2.380731651407,0.2090509676711));
#14903=CARTESIAN_POINT('Ctrl Pts',(2.323660938436,-2.472453873629,1.44620079921));
#14904=CARTESIAN_POINT('Ctrl Pts',(1.868638697361,-2.51831498474,1.89491367643));
#14905=CARTESIAN_POINT('Ctrl Pts',(-2.691657648987,2.002509974399,0.7414060389974));
#14906=CARTESIAN_POINT('Ctrl Pts',(-2.869690158652,1.956648863288,0.09506308898078));
#14907=CARTESIAN_POINT('Ctrl Pts',(-2.738693987334,1.864926641066,-1.32794833216));
#14908=CARTESIAN_POINT('Ctrl Pts',(-1.182077475443,1.727343307732,-2.805240382922));
#14909=CARTESIAN_POINT('Ctrl Pts',(0.9621023949859,1.589759974399,-2.887916035812));
#14910=CARTESIAN_POINT('Ctrl Pts',(2.628165562323,1.452176641066,-1.535786616635));
#14911=CARTESIAN_POINT('Ctrl Pts',(2.988317915928,1.314593307732,0.5795194384402));
#14912=CARTESIAN_POINT('Ctrl Pts',(1.863583571592,1.177009974399,2.406851109641));
#14913=CARTESIAN_POINT('Ctrl Pts',(-0.1871568390151,1.039426641066,3.038231922694));
#14914=CARTESIAN_POINT('Ctrl Pts',(-2.144900048479,0.9018433077322,2.159926729453));
#14915=CARTESIAN_POINT('Ctrl Pts',(-3.036851112013,0.7642599743989,0.2083630261468));
#14916=CARTESIAN_POINT('Ctrl Pts',(-2.419803279919,0.6266766410655,-1.846735483687));
#14917=CARTESIAN_POINT('Ctrl Pts',(-0.6003650755214,0.4890933077322,-2.984198655165));
#14918=CARTESIAN_POINT('Ctrl Pts',(1.517392081591,0.3515099743989,-2.638825707572));
#14919=CARTESIAN_POINT('Ctrl Pts',(2.881163310862,0.2139266410655,-0.9822310416849));
#14920=CARTESIAN_POINT('Ctrl Pts',(2.813296257732,0.07634330773221,1.162430216957));
#14921=CARTESIAN_POINT('Ctrl Pts',(1.347513783853,-0.06124002560112,2.729484648334));
#14922=CARTESIAN_POINT('Ctrl Pts',(-0.7878427858918,-0.1988233589345,2.940269305325));
#14923=CARTESIAN_POINT('Ctrl Pts',(-2.531723492933,-0.3364066922678,1.69004615277));
#14924=CARTESIAN_POINT('Ctrl Pts',(-3.017601136046,-0.4739900256011,-0.3999540308542));
#14925=CARTESIAN_POINT('Ctrl Pts',(-2.004045098816,-0.6115733589345,-2.291218689916));
#14926=CARTESIAN_POINT('Ctrl Pts',(0.005312763626742,-0.7491566922678,-3.043986139712));
#14927=CARTESIAN_POINT('Ctrl Pts',(2.012030734529,-0.8867400256011,-2.284209307552));
#14928=CARTESIAN_POINT('Ctrl Pts',(3.018978854414,-1.024323358934,-0.3894182029838));
#14929=CARTESIAN_POINT('Ctrl Pts',(2.525808697441,-1.161906692268,1.698873229859));
#14930=CARTESIAN_POINT('Ctrl Pts',(0.777574565835,-1.299490025601,2.943001442258));
#14931=CARTESIAN_POINT('Ctrl Pts',(-1.357033384268,-1.437073358934,2.724764447149));
#14932=CARTESIAN_POINT('Ctrl Pts',(-2.817336269894,-1.574656692268,1.15260241828));
#14933=CARTESIAN_POINT('Ctrl Pts',(-2.877718948998,-1.712240025601,-0.992280402288));
#14934=CARTESIAN_POINT('Ctrl Pts',(-1.508164834006,-1.849823358934,-2.64411300596));
#14935=CARTESIAN_POINT('Ctrl Pts',(0.6107529028062,-1.987406692268,-2.982059848502));
#14936=CARTESIAN_POINT('Ctrl Pts',(2.426329314435,-2.124990025601,-1.838370697611));
#14937=CARTESIAN_POINT('Ctrl Pts',(3.035752732303,-2.262573358934,0.2193100031036));
#14938=CARTESIAN_POINT('Ctrl Pts',(2.437693033892,-2.354295581157,1.517172129345));
#14939=CARTESIAN_POINT('Ctrl Pts',(1.960340882815,-2.400156692268,1.987905288785));
#14940=CARTESIAN_POINT('Ctrl Pts',(-2.759938298802,2.158874760259,0.7602136634136));
#14941=CARTESIAN_POINT('Ctrl Pts',(-2.942487049769,2.113013649148,0.0974746027524));
#14942=CARTESIAN_POINT('Ctrl Pts',(-2.808167831889,2.021291426926,-1.361635073516));
#14943=CARTESIAN_POINT('Ctrl Pts',(-1.212063836518,1.883708093593,-2.876402343769));
#14944=CARTESIAN_POINT('Ctrl Pts',(0.9865085362136,1.746124760259,-2.961175272033));
#14945=CARTESIAN_POINT('Ctrl Pts',(2.694835576054,1.608541426926,-1.574745697557));
#14946=CARTESIAN_POINT('Ctrl Pts',(3.064124097754,1.470958093593,0.594220403049));
#14947=CARTESIAN_POINT('Ctrl Pts',(1.91085804474,1.333374760259,2.467906926987));
#14948=CARTESIAN_POINT('Ctrl Pts',(-0.1919045418257,1.195791426926,3.115304298539));
#14949=CARTESIAN_POINT('Ctrl Pts',(-2.199310819906,1.058208093593,2.214718690345));
#14950=CARTESIAN_POINT('Ctrl Pts',(-3.11388846013,0.9206247602593,0.2136486771017));
#14951=CARTESIAN_POINT('Ctrl Pts',(-2.481187661562,0.7830414269259,-1.893582562813));
#14952=CARTESIAN_POINT('Ctrl Pts',(-0.6155948420179,0.6454580935926,-3.059900341606));
#14953=CARTESIAN_POINT('Ctrl Pts',(1.555884538978,0.5078747602593,-2.705766142633));
#14954=CARTESIAN_POINT('Ctrl Pts',(2.954251247272,0.3702914269259,-1.00714779654));
#14955=CARTESIAN_POINT('Ctrl Pts',(2.884662576057,0.2327080935926,1.191918176025));
#14956=CARTESIAN_POINT('Ctrl Pts',(1.381696851982,0.09512476025927,2.798724874897));
#14957=CARTESIAN_POINT('Ctrl Pts',(-0.8078283949059,-0.04245857307406,3.014856613586));
#14958=CARTESIAN_POINT('Ctrl Pts',(-2.595947011594,-0.1800419064074,1.732918413874));
#14959=CARTESIAN_POINT('Ctrl Pts',(-3.094150160224,-0.3176252397407,-0.4100998683581));
#14960=CARTESIAN_POINT('Ctrl Pts',(-2.05488273103,-0.4552085730741,-2.349341200806));
#14961=CARTESIAN_POINT('Ctrl Pts',(0.00544753520622,-0.5927919064074,-3.121204485709));
#14962=CARTESIAN_POINT('Ctrl Pts',(2.063070942429,-0.7303752397407,-2.342154007871));
#14963=CARTESIAN_POINT('Ctrl Pts',(3.095562827875,-0.8679585730741,-0.3992967727786));
#14964=CARTESIAN_POINT('Ctrl Pts',(2.589882172473,-1.005541906407,1.74196941192));
#14965=CARTESIAN_POINT('Ctrl Pts',(0.7972996956837,-1.143125239741,3.017658058028));
#14966=CARTESIAN_POINT('Ctrl Pts',(-1.391457940947,-1.280708573074,2.793884933966));
#14967=CARTESIAN_POINT('Ctrl Pts',(-2.888805073264,-1.418291906407,1.181841070576));
#14968=CARTESIAN_POINT('Ctrl Pts',(-2.950719510528,-1.555875239741,-1.01745208439));
#14969=CARTESIAN_POINT('Ctrl Pts',(-1.546423219107,-1.693458573074,-2.711187566611));
#14970=CARTESIAN_POINT('Ctrl Pts',(0.6262461826055,-1.831041906407,-3.057707278746));
#14971=CARTESIAN_POINT('Ctrl Pts',(2.487879245318,-1.968625239741,-1.88500558295));
#14972=CARTESIAN_POINT('Ctrl Pts',(3.112762217264,-2.106208573074,0.2248733515957));
#14973=CARTESIAN_POINT('Ctrl Pts',(2.499531234031,-2.197930795296,1.555659007092));
#14974=CARTESIAN_POINT('Ctrl Pts',(2.010069847933,-2.243791906407,2.038333494221));
#14975=CARTESIAN_POINT('Ctrl Pts',(-2.744223782437,2.268306095628,0.755885164454));
#14976=CARTESIAN_POINT('Ctrl Pts',(-2.925733138669,2.222444984517,0.09691960257691));
#14977=CARTESIAN_POINT('Ctrl Pts',(-2.792178706563,2.130722762294,-1.353882205759));
#14978=CARTESIAN_POINT('Ctrl Pts',(-1.20516259637,1.993139428961,-2.860024705282));
#14979=CARTESIAN_POINT('Ctrl Pts',(0.9808915611733,1.855556095628,-2.944314954071));
#14980=CARTESIAN_POINT('Ctrl Pts',(2.679491741092,1.717972762294,-1.565779422098));
#14981=CARTESIAN_POINT('Ctrl Pts',(3.046677610526,1.580389428961,0.5908370352931));
#14982=CARTESIAN_POINT('Ctrl Pts',(1.899978015274,1.442806095628,2.453855176696));
#14983=CARTESIAN_POINT('Ctrl Pts',(-0.1908118771584,1.305222762294,3.09756640186));
#14984=CARTESIAN_POINT('Ctrl Pts',(-2.186788400152,1.167639428961,2.202108541372));
#14985=CARTESIAN_POINT('Ctrl Pts',(-3.096158624942,1.030056095628,0.212432205837));
#14986=CARTESIAN_POINT('Ctrl Pts',(-2.467060293522,0.8924727622944,-1.882800896359));
#14987=CARTESIAN_POINT('Ctrl Pts',(-0.6120897726388,0.754889428961,-3.04247790357));
#14988=CARTESIAN_POINT('Ctrl Pts',(1.547025655045,0.6173060956277,-2.690360071292));
#14989=CARTESIAN_POINT('Ctrl Pts',(2.937430353272,0.4797227622944,-1.001413305832));
#14990=CARTESIAN_POINT('Ctrl Pts',(2.86823790552,0.342139428961,1.18513164109));
#14991=CARTESIAN_POINT('Ctrl Pts',(1.373829756619,0.2045560956277,2.78278951581));
#14992=CARTESIAN_POINT('Ctrl Pts',(-0.8032287875387,0.06697276229438,2.997690645196));
#14993=CARTESIAN_POINT('Ctrl Pts',(-2.581166227612,-0.07061057103895,1.723051535767));
#14994=CARTESIAN_POINT('Ctrl Pts',(-3.076532710823,-0.2081939043723,-0.407764844747));
#14995=CARTESIAN_POINT('Ctrl Pts',(-2.043182654865,-0.3457772377056,-2.335964539174));
#14996=CARTESIAN_POINT('Ctrl Pts',(0.005416518070365,-0.483360571039,-3.103432994589));
#14997=CARTESIAN_POINT('Ctrl Pts',(2.051324244287,-0.6209439043723,-2.328818268625));
#14998=CARTESIAN_POINT('Ctrl Pts',(3.077937335037,-0.7585272377056,-0.3970232597536));
#14999=CARTESIAN_POINT('Ctrl Pts',(2.575135920428,-0.896110571039,1.732050999308));
#15000=CARTESIAN_POINT('Ctrl Pts',(0.7927600365466,-1.033693904372,3.000476138795));
#15001=CARTESIAN_POINT('Ctrl Pts',(-1.383535267967,-1.171277237706,2.777977132499));
#15002=CARTESIAN_POINT('Ctrl Pts',(-2.872356816207,-1.308860571039,1.17511191259));
#15003=CARTESIAN_POINT('Ctrl Pts',(-2.933918725503,-1.446443904372,-1.011658923203));
#15004=CARTESIAN_POINT('Ctrl Pts',(-1.537618205967,-1.584027237706,-2.695750626806));
#15005=CARTESIAN_POINT('Ctrl Pts',(0.6226804667018,-1.721610571039,-3.040297327555));
#15006=CARTESIAN_POINT('Ctrl Pts',(2.473713776788,-1.859193904372,-1.87427275204));
#15007=CARTESIAN_POINT('Ctrl Pts',(3.095038794669,-1.996777237706,0.2235929693621));
#15008=CARTESIAN_POINT('Ctrl Pts',(2.485299421493,-2.088499459928,1.546801407291));
#15009=CARTESIAN_POINT('Ctrl Pts',(1.998624927033,-2.134360571039,2.026727645979));
#15010=CARTESIAN_POINT('Ctrl Pts',(-2.723241031212,2.319248086811,0.7501055518504));
#15011=CARTESIAN_POINT('Ctrl Pts',(-2.90336253938,2.2733869757,0.09617854059695));
#15012=CARTESIAN_POINT('Ctrl Pts',(-2.770829284715,2.181664753478,-1.343530217087));
#15013=CARTESIAN_POINT('Ctrl Pts',(-1.195947740385,2.044081420145,-2.838156522639));
#15014=CARTESIAN_POINT('Ctrl Pts',(0.9733915155363,1.906498086811,-2.921802275403));
#15015=CARTESIAN_POINT('Ctrl Pts',(2.659003940873,1.768914753478,-1.553807235173));
#15016=CARTESIAN_POINT('Ctrl Pts',(3.023382251462,1.631331420145,0.586319405716));
#15017=CARTESIAN_POINT('Ctrl Pts',(1.885450495222,1.493748086811,2.435092627868));
#15018=CARTESIAN_POINT('Ctrl Pts',(-0.1893529006074,1.356164753478,3.07388193938));
#15019=CARTESIAN_POINT('Ctrl Pts',(-2.1700678844,1.218581420145,2.185270885497));
#15020=CARTESIAN_POINT('Ctrl Pts',(-3.072484926538,1.080998086811,0.2108079169741));
#15021=CARTESIAN_POINT('Ctrl Pts',(-2.448196776368,0.9434147534781,-1.868404715163));
#15022=CARTESIAN_POINT('Ctrl Pts',(-0.6074096414087,0.8058314201447,-3.019214656103));
#15023=CARTESIAN_POINT('Ctrl Pts',(1.535196862268,0.6682480868114,-2.669789170172));
#15024=CARTESIAN_POINT('Ctrl Pts',(2.914970315305,0.5306647534781,-0.9937563478226));
#15025=CARTESIAN_POINT('Ctrl Pts',(2.846306923502,0.3930814201447,1.176069944827));
#15026=CARTESIAN_POINT('Ctrl Pts',(1.363325245947,0.2554980868114,2.761511885139));
#15027=CARTESIAN_POINT('Ctrl Pts',(-0.797087178413,0.1179147534781,2.974769847899));
#15028=CARTESIAN_POINT('Ctrl Pts',(-2.561430239181,-0.01966857985526,1.70987682241));
#15029=CARTESIAN_POINT('Ctrl Pts',(-3.053009075134,-0.1572519131886,-0.4046470129032));
#15030=CARTESIAN_POINT('Ctrl Pts',(-2.02756017042,-0.2948352465219,-2.318103400039));
#15031=CARTESIAN_POINT('Ctrl Pts',(0.005375102551739,-0.4324185798553,-3.079703675251));
#15032=CARTESIAN_POINT('Ctrl Pts',(2.035639508015,-0.5700019131886,-2.311011770959));
#15033=CARTESIAN_POINT('Ctrl Pts',(3.054402959379,-0.7075852465219,-0.3939875596977));
#15034=CARTESIAN_POINT('Ctrl Pts',(2.55544604064,-0.8451685798553,1.718807474687));
#15035=CARTESIAN_POINT('Ctrl Pts',(0.7866984730786,-0.9827519131886,2.977534043191));
#15036=CARTESIAN_POINT('Ctrl Pts',(-1.372956547484,-1.120335246522,2.756736298041));
#15037=CARTESIAN_POINT('Ctrl Pts',(-2.850394340374,-1.257918579855,1.166126828691));
#15038=CARTESIAN_POINT('Ctrl Pts',(-2.911485537975,-1.395501913189,-1.003923625649));
#15039=CARTESIAN_POINT('Ctrl Pts',(-1.525861343972,-1.533085246522,-2.67513850868));
#15040=CARTESIAN_POINT('Ctrl Pts',(0.6179193574188,-1.670668579855,-3.017050753102));
#15041=CARTESIAN_POINT('Ctrl Pts',(2.454799386092,-1.808251913189,-1.859941778329));
#15042=CARTESIAN_POINT('Ctrl Pts',(3.071373658657,-1.945835246522,0.2218833436086));
#15043=CARTESIAN_POINT('Ctrl Pts',(2.466296445201,-2.037557468744,1.534974329146));
#15044=CARTESIAN_POINT('Ctrl Pts',(1.983343137733,-2.083418579855,2.011230979028));
#15045=CARTESIAN_POINT('Ctrl Pts',(2.01902946445913,-2.11666666786796,0.734863845645197));
#15046=CARTESIAN_POINT('Ctrl Pts',(2.01902946451889,-2.11668202258293,0.734863837959268));
#15047=CARTESIAN_POINT('Ctrl Pts',(2.01902946584361,-2.1166973773117,0.734863830734622));
#15048=CARTESIAN_POINT('Ctrl Pts',(2.0190294684334,-2.11671273205414,0.734863823971304));
#15049=CARTESIAN_POINT('Ctrl Pts',(2.01903548208762,-2.15236732805478,0.734848119158269));
#15050=CARTESIAN_POINT('Ctrl Pts',(2.02586252056251,-2.18809959722609,0.737319747367766));
#15051=CARTESIAN_POINT('Ctrl Pts',(2.03820710077089,-2.22243716863227,0.741802872331295));
#15052=CARTESIAN_POINT('Ctrl Pts',(2.04907580053001,-2.25266944447893,0.745750008514841));
#15053=CARTESIAN_POINT('Ctrl Pts',(2.06422244902162,-2.28182080703269,0.75125674949461));
#15054=CARTESIAN_POINT('Ctrl Pts',(2.08275044399805,-2.3088469914139,0.757996028301507));
#15055=CARTESIAN_POINT('Ctrl Pts',(2.09424913019561,-2.32561975142987,0.762178502028261));
#15056=CARTESIAN_POINT('Ctrl Pts',(2.1070499859288,-2.34157319175473,0.766835634157785));
#15057=CARTESIAN_POINT('Ctrl Pts',(2.12093514751278,-2.35644804570745,0.771887967645838));
#15058=CARTESIAN_POINT('Ctrl Pts',(2.12121072935012,-2.35674327018558,0.771988242413044));
#15059=CARTESIAN_POINT('Ctrl Pts',(2.12148674218689,-2.35703807399843,0.77208867472817));
#15060=CARTESIAN_POINT('Ctrl Pts',(2.12176318420811,-2.35733245490323,0.772189263929199));
#15061=CARTESIAN_POINT('Ctrl Pts',(2.14134918971209,-2.37818943603857,0.779316040952179));
#15062=CARTESIAN_POINT('Ctrl Pts',(2.16309415443761,-2.3969226989842,0.787232005697749));
#15063=CARTESIAN_POINT('Ctrl Pts',(2.18632484782624,-2.41273811410247,0.795691621595359));
#15064=CARTESIAN_POINT('Ctrl Pts',(2.21101485867412,-2.42954702997516,0.804682657927619));
#15065=CARTESIAN_POINT('Ctrl Pts',(2.23738150094186,-2.44305736749398,0.814287210804268));
#15066=CARTESIAN_POINT('Ctrl Pts',(2.2645681620712,-2.45234913529765,0.82419282825343));
#15067=CARTESIAN_POINT('Ctrl Pts',(2.28827459351538,-2.46045144162298,0.832830403859112));
#15068=CARTESIAN_POINT('Ctrl Pts',(2.31260281779126,-2.4653456070908,0.841696272796586));
#15069=CARTESIAN_POINT('Ctrl Pts',(2.33697436671365,-2.46646509645855,0.850579343032716));
#15070=CARTESIAN_POINT('Ctrl Pts',(2.34055223916708,-2.46662944342654,0.851883424788085));
#15071=CARTESIAN_POINT('Ctrl Pts',(2.34413104789601,-2.46671253148602,0.8531878779859));
#15072=CARTESIAN_POINT('Ctrl Pts',(2.34770897025998,-2.46671266849111,0.854492037291276));
#15073=CARTESIAN_POINT('Ctrl Pts',(2.3482169537651,-2.46671268794271,0.854677198216468));
#15074=CARTESIAN_POINT('Ctrl Pts',(2.34872491941112,-2.46671103535315,0.85486235322026));
#15075=CARTESIAN_POINT('Ctrl Pts',(2.34923286192811,-2.46670771626141,0.8550475003789));
#15076=CARTESIAN_POINT('Ctrl Pts',(2.3791440767032,-2.46651226488167,0.865950262486324));
#15077=CARTESIAN_POINT('Ctrl Pts',(2.40903830687,-2.4605323337516,0.876843657964342));
#15078=CARTESIAN_POINT('Ctrl Pts',(2.43787213578489,-2.44985748919329,0.887348258852877));
#15079=CARTESIAN_POINT('Ctrl Pts',(2.45728477633215,-2.44267055190099,0.894420578028505));
#15080=CARTESIAN_POINT('Ctrl Pts',(2.47621682134733,-2.43335694704768,0.901316688346371));
#15081=CARTESIAN_POINT('Ctrl Pts',(2.49435736808247,-2.42225965114417,0.907923562114362));
#15082=CARTESIAN_POINT('Ctrl Pts',(2.51927659281981,-2.40701556756533,0.916999262788638));
#15083=CARTESIAN_POINT('Ctrl Pts',(2.5426999565375,-2.38840626533803,0.925528330549401));
#15084=CARTESIAN_POINT('Ctrl Pts',(2.56389875562379,-2.36732903978015,0.933245972984017));
#15085=CARTESIAN_POINT('Ctrl Pts',(2.56800440129363,-2.36324693968138,0.934740675826101));
#15086=CARTESIAN_POINT('Ctrl Pts',(2.57202675117484,-2.35907226476846,0.936204996181314));
#15087=CARTESIAN_POINT('Ctrl Pts',(2.57596073679862,-2.35481151043351,0.937637092926701));
#15088=CARTESIAN_POINT('Ctrl Pts',(2.58917727405375,-2.34049716773172,0.942448335721781));
#15089=CARTESIAN_POINT('Ctrl Pts',(2.60140094411319,-2.32520667963406,0.946896870192865));
#15090=CARTESIAN_POINT('Ctrl Pts',(2.61244940192908,-2.30917261084363,0.950916358239321));
#15091=CARTESIAN_POINT('Ctrl Pts',(2.62939488883081,-2.28458048158927,0.957081217007656));
#15092=CARTESIAN_POINT('Ctrl Pts',(2.64357382956465,-2.25824081065372,0.962236059039643));
#15093=CARTESIAN_POINT('Ctrl Pts',(2.65420089843072,-2.23096428845327,0.966095278883079));
#15094=CARTESIAN_POINT('Ctrl Pts',(2.66348159972914,-2.207143490998,0.969465565371594));
#15095=CARTESIAN_POINT('Ctrl Pts',(2.67005398496024,-2.18260765891923,0.971847936252335));
#15096=CARTESIAN_POINT('Ctrl Pts',(2.67341809597679,-2.15787551631565,0.973060682827448));
#15097=CARTESIAN_POINT('Ctrl Pts',(2.67528171007863,-2.14417466949522,0.973732507154356));
#15098=CARTESIAN_POINT('Ctrl Pts',(2.67616137518176,-2.13041322894896,0.974045620035525));
#15099=CARTESIAN_POINT('Ctrl Pts',(2.67610312119081,-2.11667678879524,0.974016832256147));
#15100=CARTESIAN_POINT('Ctrl Pts',(2.16568648002,-1.914085246522,-0.2047176459706));
#15101=CARTESIAN_POINT('Ctrl Pts',(2.214844963183,-1.959946357633,0.3153247854411));
#15102=CARTESIAN_POINT('Ctrl Pts',(1.921795013418,-2.051668579855,1.389512218641));
#15103=CARTESIAN_POINT('Ctrl Pts',(0.5274877970284,-2.189251913189,2.312464102902));
#15104=CARTESIAN_POINT('Ctrl Pts',(-1.128979488109,-2.326835246522,2.085795659563));
#15105=CARTESIAN_POINT('Ctrl Pts',(-2.224447131318,-2.464418579855,0.8228556269872));
#15106=CARTESIAN_POINT('Ctrl Pts',(-2.214599923529,-2.602001913189,-0.8489986687962));
#15107=CARTESIAN_POINT('Ctrl Pts',(-1.104326028381,-2.739585246522,-2.09897809787));
#15108=CARTESIAN_POINT('Ctrl Pts',(0.5546826841579,-2.877168579855,-2.305986801935));
#15109=CARTESIAN_POINT('Ctrl Pts',(1.938071910246,-3.014751913189,-1.367159299658));
#15110=CARTESIAN_POINT('Ctrl Pts',(2.358441099535,-3.152335246522,0.2510038654405));
#15111=CARTESIAN_POINT('Ctrl Pts',(1.606910543807,-3.289918579855,1.744444291083));
#15112=CARTESIAN_POINT('Ctrl Pts',(0.05691270016944,-3.427501913189,2.371077457865));
#15113=CARTESIAN_POINT('Ctrl Pts',(-1.521364831366,-3.565085246522,1.819531923506));
#15114=CARTESIAN_POINT('Ctrl Pts',(-2.343682391654,-3.702668579855,0.3638684063681));
#15115=CARTESIAN_POINT('Ctrl Pts',(-2.001433743259,-3.840251913189,-1.272599835542));
#15116=CARTESIAN_POINT('Ctrl Pts',(-0.6646808418357,-3.977835246522,-2.276718416632));
#15117=CARTESIAN_POINT('Ctrl Pts',(1.002349255295,-4.115418579855,-2.149544914748));
#15118=CARTESIAN_POINT('Ctrl Pts',(2.171316101136,-4.253001913189,-0.9542713236204));
#15119=CARTESIAN_POINT('Ctrl Pts',(2.261364844106,-4.390585246522,0.715175790919));
#15120=CARTESIAN_POINT('Ctrl Pts',(1.227750631671,-4.528168579855,2.029254975732));
#15121=CARTESIAN_POINT('Ctrl Pts',(-0.4159278556647,-4.665751913189,2.335005650883));
#15122=CARTESIAN_POINT('Ctrl Pts',(-1.852933489305,-4.803335246522,1.480501553815));
#15123=CARTESIAN_POINT('Ctrl Pts',(-2.369224042948,-4.940918579855,-0.1096577165763));
#15124=CARTESIAN_POINT('Ctrl Pts',(-1.708256833279,-5.078501913189,-1.645328524034));
#15125=CARTESIAN_POINT('Ctrl Pts',(-0.198463826226,-5.216085246522,-2.363442275497));
#15126=CARTESIAN_POINT('Ctrl Pts',(1.409945218843,-5.353668579855,-1.907171332278));
#15127=CARTESIAN_POINT('Ctrl Pts',(2.317757596199,-5.491251913189,-0.5032342968815));
#15128=CARTESIAN_POINT('Ctrl Pts',(2.073888103704,-5.628835246522,1.150756140208));
#15129=CARTESIAN_POINT('Ctrl Pts',(0.7995030738709,-5.766418579855,2.232946765546));
#15130=CARTESIAN_POINT('Ctrl Pts',(-0.872118147943,-5.904001913189,2.205572069566));
#15131=CARTESIAN_POINT('Ctrl Pts',(-2.110512896131,-6.041585246522,1.082344177464));
#15132=CARTESIAN_POINT('Ctrl Pts',(-2.299734136718,-6.179168579855,-0.5790191531922));
#15133=CARTESIAN_POINT('Ctrl Pts',(-1.665227699375,-6.270890802077,-1.493982811308));
#15134=CARTESIAN_POINT('Ctrl Pts',(-1.235253620718,-6.316751913189,-1.790602059871));
#15135=CARTESIAN_POINT('Ctrl Pts',(2.149561232942,-1.951996799872,-0.2031933613371));
#15136=CARTESIAN_POINT('Ctrl Pts',(2.198353692354,-1.997857910983,0.3129769432571));
#15137=CARTESIAN_POINT('Ctrl Pts',(1.907485731021,-2.089580133205,1.379166202239));
#15138=CARTESIAN_POINT('Ctrl Pts',(0.5235602335809,-2.227163466539,2.295245980444));
#15139=CARTESIAN_POINT('Ctrl Pts',(-1.120573343748,-2.364746799872,2.070265262769));
#15140=CARTESIAN_POINT('Ctrl Pts',(-2.20788436476,-2.502330133205,0.8167288166584));
#15141=CARTESIAN_POINT('Ctrl Pts',(-2.198110477214,-2.639913466539,-0.842677202864));
#15142=CARTESIAN_POINT('Ctrl Pts',(-1.096103448508,-2.777496799872,-2.083349547407));
#15143=CARTESIAN_POINT('Ctrl Pts',(0.5505526332874,-2.915080133205,-2.2888169081));
#15144=CARTESIAN_POINT('Ctrl Pts',(1.923641433491,-3.052663466539,-1.3569797184));
#15145=CARTESIAN_POINT('Ctrl Pts',(2.340880642008,-3.190246799872,0.2491349433296));
#15146=CARTESIAN_POINT('Ctrl Pts',(1.594945825095,-3.327830133205,1.731455524949));
#15147=CARTESIAN_POINT('Ctrl Pts',(0.05648894014665,-3.465413466539,2.353422912665));
#15148=CARTESIAN_POINT('Ctrl Pts',(-1.510037068078,-3.602996799872,1.805984070618));
#15149=CARTESIAN_POINT('Ctrl Pts',(-2.326231824369,-3.740580133205,0.3611591185692));
#15150=CARTESIAN_POINT('Ctrl Pts',(-1.986531487591,-3.878163466539,-1.263124324211));
#15151=CARTESIAN_POINT('Ctrl Pts',(-0.6597317677654,-4.015746799872,-2.259766449053));
#15152=CARTESIAN_POINT('Ctrl Pts',(0.9948859730751,-4.153330133205,-2.133539854377));
#15153=CARTESIAN_POINT('Ctrl Pts',(2.15514893708,-4.290913466539,-0.9471660195909));
#15154=CARTESIAN_POINT('Ctrl Pts',(2.244527196006,-4.428496799872,0.7098507420537));
#15155=CARTESIAN_POINT('Ctrl Pts',(1.218609058101,-4.566080133205,2.014145569006));
#15156=CARTESIAN_POINT('Ctrl Pts',(-0.4128309441306,-4.703663466539,2.317619688789));
#15157=CARTESIAN_POINT('Ctrl Pts',(-1.839136935367,-4.841246799872,1.469478049916));
#15158=CARTESIAN_POINT('Ctrl Pts',(-2.351583297887,-4.978830133205,-0.1088412282295));
#15159=CARTESIAN_POINT('Ctrl Pts',(-1.695537511362,-5.116413466539,-1.633077753103));
#15160=CARTESIAN_POINT('Ctrl Pts',(-0.196986106222,-5.253996799872,-2.345844580263));
#15161=CARTESIAN_POINT('Ctrl Pts',(1.39944706261,-5.391580133205,-1.892970934742));
#15162=CARTESIAN_POINT('Ctrl Pts',(2.300500059501,-5.529163466539,-0.4994873199066));
#15163=CARTESIAN_POINT('Ctrl Pts',(2.058446368072,-5.666746799872,1.142187851465));
#15164=CARTESIAN_POINT('Ctrl Pts',(0.7935501417522,-5.804330133205,2.216320712496));
#15165=CARTESIAN_POINT('Ctrl Pts',(-0.8656245392205,-5.941913466539,2.189149842758));
#15166=CARTESIAN_POINT('Ctrl Pts',(-2.094798459981,-6.079496799872,1.07428526984));
#15167=CARTESIAN_POINT('Ctrl Pts',(-2.282610798917,-6.217080133205,-0.5747078980801));
#15168=CARTESIAN_POINT('Ctrl Pts',(-1.652828763361,-6.308802355428,-1.482858928795));
#15169=CARTESIAN_POINT('Ctrl Pts',(-1.226056181467,-6.354663466539,-1.777269612677));
#15170=CARTESIAN_POINT('Ctrl Pts',(2.10063415235,-2.166998399936,-0.1985683905227));
#15171=CARTESIAN_POINT('Ctrl Pts',(2.14831602577,-2.212859511047,0.3058531414823));
#15172=CARTESIAN_POINT('Ctrl Pts',(1.864068634239,-2.304581733269,1.347774411722));
#15173=CARTESIAN_POINT('Ctrl Pts',(0.5116432556643,-2.442165066603,2.24300290714));
#15174=CARTESIAN_POINT('Ctrl Pts',(-1.095067495643,-2.579748399936,2.023143071595));
#15175=CARTESIAN_POINT('Ctrl Pts',(-2.157629766474,-2.717331733269,0.7981389035067));
#15176=CARTESIAN_POINT('Ctrl Pts',(-2.148078346554,-2.854915066603,-0.8234966674198));
#15177=CARTESIAN_POINT('Ctrl Pts',(-1.071154570131,-2.992498399936,-2.035929539246));
#15178=CARTESIAN_POINT('Ctrl Pts',(0.5380212698415,-3.130081733269,-2.236720169656));
#15179=CARTESIAN_POINT('Ctrl Pts',(1.87985660987,-3.267665066603,-1.326092923911));
#15180=CARTESIAN_POINT('Ctrl Pts',(2.287598858697,-3.405248399936,0.2434642765611));
#15181=CARTESIAN_POINT('Ctrl Pts',(1.558642582494,-3.542831733269,1.692045126811));
#15182=CARTESIAN_POINT('Ctrl Pts',(0.05520317127216,-3.680415066603,2.299855649378));
#15183=CARTESIAN_POINT('Ctrl Pts',(-1.475666469932,-3.817998399936,1.764877296446));
#15184=CARTESIAN_POINT('Ctrl Pts',(-2.273283469047,-3.955581733269,0.3529386217393));
#15185=CARTESIAN_POINT('Ctrl Pts',(-1.941315196609,-4.093165066603,-1.234373812404));
#15186=CARTESIAN_POINT('Ctrl Pts',(-0.6447153314452,-4.230748399936,-2.208330940504));
#15187=CARTESIAN_POINT('Ctrl Pts',(0.972240948854,-4.368331733269,-2.08497744322));
#15188=CARTESIAN_POINT('Ctrl Pts',(2.106094672369,-4.505915066603,-0.9256071695965));
#15189=CARTESIAN_POINT('Ctrl Pts',(2.1934385546,-4.643498399936,0.6936935263705));
#15190=CARTESIAN_POINT('Ctrl Pts',(1.190871777263,-4.781081733269,1.968300742132));
#15191=CARTESIAN_POINT('Ctrl Pts',(-0.4034343228272,-4.918665066603,2.264867357961));
#15192=CARTESIAN_POINT('Ctrl Pts',(-1.797275554691,-5.056248399936,1.436030632892));
#15193=CARTESIAN_POINT('Ctrl Pts',(-2.298057906858,-5.193831733269,-0.1063638465836));
#15194=CARTESIAN_POINT('Ctrl Pts',(-1.656944658461,-5.331415066603,-1.595906573415));
#15195=CARTESIAN_POINT('Ctrl Pts',(-0.1925024213904,-5.468998399936,-2.292449810634));
#15196=CARTESIAN_POINT('Ctrl Pts',(1.367593650775,-5.606581733269,-1.849884215432));
#15197=CARTESIAN_POINT('Ctrl Pts',(2.248137395861,-5.744165066603,-0.4881182758517));
#15198=CARTESIAN_POINT('Ctrl Pts',(2.011593191805,-5.881748399936,1.116190026326));
#15199=CARTESIAN_POINT('Ctrl Pts',(0.775487808312,-6.019331733269,2.165874090898));
#15200=CARTESIAN_POINT('Ctrl Pts',(-0.8459216896603,-6.156915066603,2.139321668922));
#15201=CARTESIAN_POINT('Ctrl Pts',(-2.047117858235,-6.294498399936,1.04983300434));
#15202=CARTESIAN_POINT('Ctrl Pts',(-2.230655320372,-6.432081733269,-0.5616267263435));
#15203=CARTESIAN_POINT('Ctrl Pts',(-1.615208022499,-6.523803955492,-1.449106943876));
#15204=CARTESIAN_POINT('Ctrl Pts',(-1.198149393476,-6.569665066603,-1.736816420537));
#15205=CARTESIAN_POINT('Ctrl Pts',(2.488904911508,-2.557,-0.2352707832963));
#15206=CARTESIAN_POINT('Ctrl Pts',(2.545400065037,-2.602861111111,0.3623855135288));
#15207=CARTESIAN_POINT('Ctrl Pts',(2.208613800721,-2.694583333333,1.596890324375));
#15208=CARTESIAN_POINT('Ctrl Pts',(0.6062128479337,-2.832166666667,2.657588398181));
#15209=CARTESIAN_POINT('Ctrl Pts',(-1.297474319976,-2.96975,2.397090765159));
#15210=CARTESIAN_POINT('Ctrl Pts',(-2.556435311206,-3.107333333333,0.9456629250653));
#15211=CARTESIAN_POINT('Ctrl Pts',(-2.545118454378,-3.244916666667,-0.9757076918219));
#15212=CARTESIAN_POINT('Ctrl Pts',(-1.269141448358,-3.3825,-2.412240619837));
#15213=CARTESIAN_POINT('Ctrl Pts',(0.6374664429341,-3.520083333333,-2.650144390777));
#15214=CARTESIAN_POINT('Ctrl Pts',(2.22731994717,-3.657666666667,-1.571201338294));
#15215=CARTESIAN_POINT('Ctrl Pts',(2.710427243412,-3.79525,0.2884650014053));
#15216=CARTESIAN_POINT('Ctrl Pts',(1.846734318071,-3.932833333333,2.004794324563));
#15217=CARTESIAN_POINT('Ctrl Pts',(0.06540665063283,-4.070416666667,2.724949518265));
#15218=CARTESIAN_POINT('Ctrl Pts',(-1.748421313941,-4.208,2.091088429853));
#15219=CARTESIAN_POINT('Ctrl Pts',(-2.693465868406,-4.345583333333,0.4181740395515));
#15220=CARTESIAN_POINT('Ctrl Pts',(-2.300138233124,-4.483166666667,-1.46252932282));
#15221=CARTESIAN_POINT('Ctrl Pts',(-0.7638813037308,-4.62075,-2.616507837839));
#15222=CARTESIAN_POINT('Ctrl Pts',(1.151945125744,-4.758333333333,-2.470354294206));
#15223=CARTESIAN_POINT('Ctrl Pts',(2.495374726863,-4.895916666667,-1.096691790885));
#15224=CARTESIAN_POINT('Ctrl Pts',(2.598862817463,-5.0335,0.8219123843785));
#15225=CARTESIAN_POINT('Ctrl Pts',(1.41098658807,-5.171083333333,2.332111652539));
#15226=CARTESIAN_POINT('Ctrl Pts',(-0.4780031146462,-5.308666666667,2.683494165244));
#15227=CARTESIAN_POINT('Ctrl Pts',(-2.129475020865,-5.44625,1.701459386102));
#15228=CARTESIAN_POINT('Ctrl Pts',(-2.722819489967,-5.583833333333,-0.1260236104762));
#15229=CARTESIAN_POINT('Ctrl Pts',(-1.963206060383,-5.721416666667,-1.890885999562));
#15230=CARTESIAN_POINT('Ctrl Pts',(-0.2280836106277,-5.859,-2.716174821156));
#15231=CARTESIAN_POINT('Ctrl Pts',(1.620372852909,-5.996583333333,-2.191807604556));
#15232=CARTESIAN_POINT('Ctrl Pts',(2.663671920236,-6.134166666667,-0.5783396279667));
#15233=CARTESIAN_POINT('Ctrl Pts',(2.383406063087,-6.27175,1.322501034076));
#15234=CARTESIAN_POINT('Ctrl Pts',(0.9188251141986,-6.409333333333,2.566203475515));
#15235=CARTESIAN_POINT('Ctrl Pts',(-1.002277643535,-6.546916666667,2.534743236046));
#15236=CARTESIAN_POINT('Ctrl Pts',(-2.425496932009,-6.6845,1.243878910491));
#15237=CARTESIAN_POINT('Ctrl Pts',(-2.642958544944,-6.822083333333,-0.6654350145011));
#15238=CARTESIAN_POINT('Ctrl Pts',(-1.913755032407,-6.913805555556,-1.71695265731));
#15239=CARTESIAN_POINT('Ctrl Pts',(-1.419609362633,-6.959666666667,-2.057840921336));
#15240=CARTESIAN_POINT('Ctrl Pts',(2.877175670666,-2.166998399936,-0.2719731760698));
#15241=CARTESIAN_POINT('Ctrl Pts',(2.942484104304,-2.212859511047,0.4189178855753));
#15242=CARTESIAN_POINT('Ctrl Pts',(2.553158967202,-2.304581733269,1.846006237029));
#15243=CARTESIAN_POINT('Ctrl Pts',(0.700782440203,-2.442165066603,3.072173889222));
#15244=CARTESIAN_POINT('Ctrl Pts',(-1.499881144309,-2.579748399936,2.771038458724));
#15245=CARTESIAN_POINT('Ctrl Pts',(-2.955240855938,-2.717331733269,1.093186946624));
#15246=CARTESIAN_POINT('Ctrl Pts',(-2.942158562201,-2.854915066603,-1.127918716224));
#15247=CARTESIAN_POINT('Ctrl Pts',(-1.467128326585,-2.992498399936,-2.788551700427));
#15248=CARTESIAN_POINT('Ctrl Pts',(0.7369116160266,-3.130081733269,-3.063568611899));
#15249=CARTESIAN_POINT('Ctrl Pts',(2.574783284471,-3.267665066603,-1.816309752677));
#15250=CARTESIAN_POINT('Ctrl Pts',(3.133255628127,-3.405248399936,0.3334657262495));
#15251=CARTESIAN_POINT('Ctrl Pts',(2.134826053647,-3.542831733269,2.317543522314));
#15252=CARTESIAN_POINT('Ctrl Pts',(0.07561012999347,-3.680415066603,3.150043387152));
#15253=CARTESIAN_POINT('Ctrl Pts',(-2.02117615795,-3.817998399936,2.41729956326));
#15254=CARTESIAN_POINT('Ctrl Pts',(-3.113648267764,-3.955581733269,0.4834094573636));
#15255=CARTESIAN_POINT('Ctrl Pts',(-2.658961269639,-4.093165066603,-1.690684833236));
#15256=CARTESIAN_POINT('Ctrl Pts',(-0.8830472760164,-4.230748399936,-3.024684735174));
#15257=CARTESIAN_POINT('Ctrl Pts',(1.331649302635,-4.368331733269,-2.855731145192));
#15258=CARTESIAN_POINT('Ctrl Pts',(2.884654781358,-4.505915066603,-1.267776412174));
#15259=CARTESIAN_POINT('Ctrl Pts',(3.004287080326,-4.643498399936,0.9501312423865));
#15260=CARTESIAN_POINT('Ctrl Pts',(1.631101398876,-4.781081733269,2.695922562946));
#15261=CARTESIAN_POINT('Ctrl Pts',(-0.5525719064653,-4.918665066603,3.102120972527));
#15262=CARTESIAN_POINT('Ctrl Pts',(-2.461674487038,-5.056248399936,1.966888139311));
#15263=CARTESIAN_POINT('Ctrl Pts',(-3.147581073076,-5.193831733269,-0.1456833743688));
#15264=CARTESIAN_POINT('Ctrl Pts',(-2.269467462304,-5.331415066603,-2.185865425709));
#15265=CARTESIAN_POINT('Ctrl Pts',(-0.263664799865,-5.468998399936,-3.139899831678));
#15266=CARTESIAN_POINT('Ctrl Pts',(1.873152055043,-5.606581733269,-2.53373099368));
#15267=CARTESIAN_POINT('Ctrl Pts',(3.079206444611,-5.744165066603,-0.6685609800817));
#15268=CARTESIAN_POINT('Ctrl Pts',(2.755218934369,-5.881748399936,1.528812041827));
#15269=CARTESIAN_POINT('Ctrl Pts',(1.062162420085,-6.019331733269,2.966532860131));
#15270=CARTESIAN_POINT('Ctrl Pts',(-1.15863359741,-6.156915066603,2.930164803169));
#15271=CARTESIAN_POINT('Ctrl Pts',(-2.803876005782,-6.294498399936,1.437924816642));
#15272=CARTESIAN_POINT('Ctrl Pts',(-3.055261769517,-6.432081733269,-0.7692433026587));
#15273=CARTESIAN_POINT('Ctrl Pts',(-2.212302042314,-6.523803955492,-1.984798370744));
#15274=CARTESIAN_POINT('Ctrl Pts',(-1.64106933179,-6.569665066603,-2.378865422135));
#15275=CARTESIAN_POINT('Ctrl Pts',(2.828248590073,-1.951996799872,-0.2673482052555));
#15276=CARTESIAN_POINT('Ctrl Pts',(2.89244643772,-1.997857910983,0.4117940838004));
#15277=CARTESIAN_POINT('Ctrl Pts',(2.50974187042,-2.089580133205,1.814614446512));
#15278=CARTESIAN_POINT('Ctrl Pts',(0.6888654622864,-2.227163466539,3.019930815918));
#15279=CARTESIAN_POINT('Ctrl Pts',(-1.474375296204,-2.364746799872,2.72391626755));
#15280=CARTESIAN_POINT('Ctrl Pts',(-2.904986257652,-2.502330133205,1.074597033472));
#15281=CARTESIAN_POINT('Ctrl Pts',(-2.892126431541,-2.639913466539,-1.10873818078));
#15282=CARTESIAN_POINT('Ctrl Pts',(-1.442179448209,-2.777496799872,-2.741131692266));
#15283=CARTESIAN_POINT('Ctrl Pts',(0.7243802525807,-2.915080133205,-3.011471873454));
#15284=CARTESIAN_POINT('Ctrl Pts',(2.53099846085,-3.052663466539,-1.785422958187));
#15285=CARTESIAN_POINT('Ctrl Pts',(3.079973844815,-3.190246799872,0.3277950594809));
#15286=CARTESIAN_POINT('Ctrl Pts',(2.098522811046,-3.327830133205,2.278133124177));
#15287=CARTESIAN_POINT('Ctrl Pts',(0.07432436111898,-3.465413466539,3.096476123865));
#15288=CARTESIAN_POINT('Ctrl Pts',(-1.986805559805,-3.602996799872,2.376192789088));
#15289=CARTESIAN_POINT('Ctrl Pts',(-3.060699912442,-3.740580133205,0.4751889605338));
#15290=CARTESIAN_POINT('Ctrl Pts',(-2.613744978657,-3.878163466539,-1.661934321428));
#15291=CARTESIAN_POINT('Ctrl Pts',(-0.8680308396962,-4.015746799872,-2.973249226626));
#15292=CARTESIAN_POINT('Ctrl Pts',(1.309004278414,-4.153330133205,-2.807168734035));
#15293=CARTESIAN_POINT('Ctrl Pts',(2.835600516647,-4.290913466539,-1.24621756218));
#15294=CARTESIAN_POINT('Ctrl Pts',(2.95319843892,-4.428496799872,0.9339740267032));
#15295=CARTESIAN_POINT('Ctrl Pts',(1.603364118038,-4.566080133205,2.650077736072));
#15296=CARTESIAN_POINT('Ctrl Pts',(-0.5431752851618,-4.703663466539,3.049368641699));
#15297=CARTESIAN_POINT('Ctrl Pts',(-2.419813106363,-4.841246799872,1.933440722287));
#15298=CARTESIAN_POINT('Ctrl Pts',(-3.094055682046,-4.978830133205,-0.1432059927228));
#15299=CARTESIAN_POINT('Ctrl Pts',(-2.230874609403,-5.116413466539,-2.148694246022));
#15300=CARTESIAN_POINT('Ctrl Pts',(-0.2591811150334,-5.253996799872,-3.086505062049));
#15301=CARTESIAN_POINT('Ctrl Pts',(1.841298643208,-5.391580133205,-2.49064427437));
#15302=CARTESIAN_POINT('Ctrl Pts',(3.026843780971,-5.529163466539,-0.6571919360268));
#15303=CARTESIAN_POINT('Ctrl Pts',(2.708365758102,-5.666746799872,1.502814216688));
#15304=CARTESIAN_POINT('Ctrl Pts',(1.044100086645,-5.804330133205,2.916086238533));
#15305=CARTESIAN_POINT('Ctrl Pts',(-1.13893074785,-5.941913466539,2.880336629334));
#15306=CARTESIAN_POINT('Ctrl Pts',(-2.756195404036,-6.079496799872,1.413472551141));
#15307=CARTESIAN_POINT('Ctrl Pts',(-3.003306290972,-6.217080133205,-0.7561621309221));
#15308=CARTESIAN_POINT('Ctrl Pts',(-2.174681301453,-6.308802355428,-1.951046385826));
#15309=CARTESIAN_POINT('Ctrl Pts',(-1.613162543799,-6.354663466539,-2.338412229995));
#15310=CARTESIAN_POINT('Ctrl Pts',(2.812123342995,-1.914085246522,-0.265823920622));
#15311=CARTESIAN_POINT('Ctrl Pts',(2.875955166892,-1.959946357633,0.4094462416164));
#15312=CARTESIAN_POINT('Ctrl Pts',(2.495432588024,-2.051668579855,1.80426843011));
#15313=CARTESIAN_POINT('Ctrl Pts',(0.6849378988389,-2.189251913189,3.00271269346));
#15314=CARTESIAN_POINT('Ctrl Pts',(-1.465969151843,-2.326835246522,2.708385870756));
#15315=CARTESIAN_POINT('Ctrl Pts',(-2.888423491095,-2.464418579855,1.068470223143));
#15316=CARTESIAN_POINT('Ctrl Pts',(-2.875636985226,-2.602001913189,-1.102416714848));
#15317=CARTESIAN_POINT('Ctrl Pts',(-1.433956868336,-2.739585246522,-2.725503141803));
#15318=CARTESIAN_POINT('Ctrl Pts',(0.7202502017102,-2.877168579855,-2.994301979619));
#15319=CARTESIAN_POINT('Ctrl Pts',(2.516567984095,-3.014751913189,-1.775243376929));
#15320=CARTESIAN_POINT('Ctrl Pts',(3.062413387288,-3.152335246522,0.32592613737));
#15321=CARTESIAN_POINT('Ctrl Pts',(2.086558092334,-3.289918579855,2.265144358043));
#15322=CARTESIAN_POINT('Ctrl Pts',(0.07390060109619,-3.427501913189,3.078821578666));
#15323=CARTESIAN_POINT('Ctrl Pts',(-1.975477796517,-3.565085246522,2.3626449362));
#15324=CARTESIAN_POINT('Ctrl Pts',(-3.043249345157,-3.702668579855,0.4724796727348));
#15325=CARTESIAN_POINT('Ctrl Pts',(-2.598842722989,-3.840251913189,-1.652458810098));
#15326=CARTESIAN_POINT('Ctrl Pts',(-0.8630817656259,-3.977835246522,-2.956297259047));
#15327=CARTESIAN_POINT('Ctrl Pts',(1.301540996194,-4.115418579855,-2.791163673665));
#15328=CARTESIAN_POINT('Ctrl Pts',(2.819433352591,-4.253001913189,-1.239112258151));
#15329=CARTESIAN_POINT('Ctrl Pts',(2.93636079082,-4.390585246522,0.928648977838));
#15330=CARTESIAN_POINT('Ctrl Pts',(1.594222544469,-4.528168579855,2.634968329346));
#15331=CARTESIAN_POINT('Ctrl Pts',(-0.5400783736277,-4.665751913189,3.031982679605));
#15332=CARTESIAN_POINT('Ctrl Pts',(-2.406016552425,-4.803335246522,1.922417218389));
#15333=CARTESIAN_POINT('Ctrl Pts',(-3.076414936985,-4.940918579855,-0.142389504376));
#15334=CARTESIAN_POINT('Ctrl Pts',(-2.218155287486,-5.078501913189,-2.136443475091));
#15335=CARTESIAN_POINT('Ctrl Pts',(-0.2577033950294,-5.216085246522,-3.068907366815));
#15336=CARTESIAN_POINT('Ctrl Pts',(1.830800486974,-5.353668579855,-2.476443876835));
#15337=CARTESIAN_POINT('Ctrl Pts',(3.009586244273,-5.491251913189,-0.653444959052));
#15338=CARTESIAN_POINT('Ctrl Pts',(2.69292402247,-5.628835246522,1.494245927945));
#15339=CARTESIAN_POINT('Ctrl Pts',(1.038147154526,-5.766418579855,2.899460185483));
#15340=CARTESIAN_POINT('Ctrl Pts',(-1.132437139127,-5.904001913189,2.863914402526));
#15341=CARTESIAN_POINT('Ctrl Pts',(-2.740480967886,-6.041585246522,1.405413643517));
#15342=CARTESIAN_POINT('Ctrl Pts',(-2.98618295317,-6.179168579855,-0.75185087581));
#15343=CARTESIAN_POINT('Ctrl Pts',(-2.162282365438,-6.270890802077,-1.939922503313));
#15344=CARTESIAN_POINT('Ctrl Pts',(-1.603965104547,-6.316751913189,-2.325079782801));
#15345=CARTESIAN_POINT('',(-2.46657190792704,-6.35000032196109,-1.42407460247911));
#15346=CARTESIAN_POINT('Ctrl Pts',(2.67638549957928,-2.11666634473297,0.974128396786123));
#15347=CARTESIAN_POINT('Ctrl Pts',(2.63158429467461,-2.1254957760933,1.09794595690002));
#15348=CARTESIAN_POINT('Ctrl Pts',(2.57832130571527,-2.13432523104768,1.21881530794275));
#15349=CARTESIAN_POINT('Ctrl Pts',(2.51693294178586,-2.14315470006068,1.33539535663631));
#15350=CARTESIAN_POINT('Ctrl Pts',(2.45569542878568,-2.15196247223212,1.45168893070262));
#15351=CARTESIAN_POINT('Ctrl Pts',(2.38637276527163,-2.16077025839314,1.56371307377647));
#15352=CARTESIAN_POINT('Ctrl Pts',(2.30934763707904,-2.16957804907858,1.67015373268866));
#15353=CARTESIAN_POINT('Ctrl Pts',(2.2544280617514,-2.17585807918525,1.74604683306021));
#15354=CARTESIAN_POINT('Ctrl Pts',(2.19559382630051,-2.18213811159205,1.81910178374938));
#15355=CARTESIAN_POINT('Ctrl Pts',(2.1332634233653,-2.18841814286804,1.88903780308403));
#15356=CARTESIAN_POINT('Ctrl Pts',(2.04207818376161,-2.19760541151469,1.99134955432665));
#15357=CARTESIAN_POINT('Ctrl Pts',(1.94345554311775,-2.20679260757273,2.08694592181752));
#15358=CARTESIAN_POINT('Ctrl Pts',(1.83858684135808,-2.21597977160931,2.17511176619573));
#15359=CARTESIAN_POINT('Ctrl Pts',(1.73114043431015,-2.22539275899379,2.2654447544356));
#15360=CARTESIAN_POINT('Ctrl Pts',(1.61713621323921,-2.2348057127633,2.34797828870751));
#15361=CARTESIAN_POINT('Ctrl Pts',(1.49781311768319,-2.24421867655057,2.42190950106786));
#15362=CARTESIAN_POINT('Ctrl Pts',(1.43041393440689,-2.24953555228628,2.46366925686782));
#15363=CARTESIAN_POINT('Ctrl Pts',(1.36131707299677,-2.25485243121816,2.50268375528082));
#15364=CARTESIAN_POINT('Ctrl Pts',(1.29074180256227,-2.26016932120947,2.53880214744044));
#15365=CARTESIAN_POINT('Ctrl Pts',(1.17763832214355,-2.26869013536035,2.59668525345238));
#15366=CARTESIAN_POINT('Ctrl Pts',(1.06062583874571,-2.27721098490573,2.64718152713231));
#15367=CARTESIAN_POINT('Ctrl Pts',(0.940746669490456,-2.28573185613866,
2.68956035801277));
#15368=CARTESIAN_POINT('Ctrl Pts',(0.840248387944155,-2.29287515652609,
2.72508779538063));
#15369=CARTESIAN_POINT('Ctrl Pts',(0.737736391549633,-2.30001847215547,
2.75491074422656));
#15370=CARTESIAN_POINT('Ctrl Pts',(0.633838265760999,-2.307161794951,2.77862358958537));
#15371=CARTESIAN_POINT('Ctrl Pts',(0.513799258434475,-2.31541485409794,
2.80602029569679));
#15372=CARTESIAN_POINT('Ctrl Pts',(0.391910586283146,-2.32366792281057,
2.82525992132688));
#15373=CARTESIAN_POINT('Ctrl Pts',(0.269315413872178,-2.33192098863433,
2.83649454098679));
#15374=CARTESIAN_POINT('Ctrl Pts',(0.133629132011341,-2.3410553435486,2.84892882970954));
#15375=CARTESIAN_POINT('Ctrl Pts',(-0.0029017556927971,-2.35018960945232,
2.8515644826885));
#15376=CARTESIAN_POINT('Ctrl Pts',(-0.138944627445231,-2.35932384692222,
2.84464052964891));
#15377=CARTESIAN_POINT('Ctrl Pts',(-0.277065228126552,-2.36859758798529,
2.83761082981533));
#15378=CARTESIAN_POINT('Ctrl Pts',(-0.414684058841455,-2.37787129973941,
2.82072724303376));
#15379=CARTESIAN_POINT('Ctrl Pts',(-0.550411283063103,-2.38714504557935,
2.79418713351009));
#15380=CARTESIAN_POINT('Ctrl Pts',(-0.631039269717429,-2.39265406162315,
2.77842113218832));
#15381=CARTESIAN_POINT('Ctrl Pts',(-0.710999729177977,-2.39816308969545,
2.75924645530946));
#15382=CARTESIAN_POINT('Ctrl Pts',(-0.789999251472441,-2.40367214308581,
2.73669598970977));
#15383=CARTESIAN_POINT('Ctrl Pts',(-0.908818344442536,-2.41195802517665,
2.70277900147002));
#15384=CARTESIAN_POINT('Ctrl Pts',(-1.02554898172219,-2.42024391903388,
2.66119535121063));
#15385=CARTESIAN_POINT('Ctrl Pts',(-1.13901931890348,-2.42852982142298,
2.61208499993025));
#15386=CARTESIAN_POINT('Ctrl Pts',(-1.21304893126723,-2.43393565837726,
2.58004472968301));
#15387=CARTESIAN_POINT('Ctrl Pts',(-1.28569081934136,-2.43934149896308,
2.54480182943131));
#15388=CARTESIAN_POINT('Ctrl Pts',(-1.35662275119696,-2.44474734228225,
2.50640673292635));
#15389=CARTESIAN_POINT('Ctrl Pts',(-1.46519412681361,-2.45302175170798,
2.44763759559389));
#15390=CARTESIAN_POINT('Ctrl Pts',(-1.56975749516473,-2.46129616753761,
2.38148148479742));
#15391=CARTESIAN_POINT('Ctrl Pts',(-1.66953923951437,-2.46957058655012,
2.30881919414378));
#15392=CARTESIAN_POINT('Ctrl Pts',(-1.69306756156468,-2.47152167686804,
2.29168558131155));
#15393=CARTESIAN_POINT('Ctrl Pts',(-1.71633016792867,-2.47347276736293,
2.2741903971365));
#15394=CARTESIAN_POINT('Ctrl Pts',(-1.73931720410331,-2.47542385799256,
2.25634549413614));
#15395=CARTESIAN_POINT('Ctrl Pts',(-1.8460242040886,-2.48448092068674,2.17350853987499));
#15396=CARTESIAN_POINT('Ctrl Pts',(-1.9468210578866,-2.4935378834916,2.08311981244695));
#15397=CARTESIAN_POINT('Ctrl Pts',(-2.04088398830876,-2.50259482028277,
1.98619769337065));
#15398=CARTESIAN_POINT('Ctrl Pts',(-2.13553289721494,-2.51170817855758,
1.88867178408551));
#15399=CARTESIAN_POINT('Ctrl Pts',(-2.22336458635848,-2.52082151049358,
1.78452990498833));
#15400=CARTESIAN_POINT('Ctrl Pts',(-2.30350597793839,-2.5299348913556,1.67477021328633));
#15401=CARTESIAN_POINT('Ctrl Pts',(-2.35404114510278,-2.53568156253532,
1.60555848313385));
#15402=CARTESIAN_POINT('Ctrl Pts',(-2.40151773977062,-2.54142825316924,
1.53411223130499));
#15403=CARTESIAN_POINT('Ctrl Pts',(-2.44570763150553,-2.54717498212873,
1.46067629080571));
#15404=CARTESIAN_POINT('Ctrl Pts',(-2.50880633543785,-2.55538073088615,
1.35581718195448));
#15405=CARTESIAN_POINT('Ctrl Pts',(-2.56522751641537,-2.56358647960479,
1.24685081219773));
#15406=CARTESIAN_POINT('Ctrl Pts',(-2.61420861752981,-2.57179222757394,
1.1346374093582));
#15407=CARTESIAN_POINT('Ctrl Pts',(-2.63518312611563,-2.57530606305979,
1.08658579500589));
#15408=CARTESIAN_POINT('Ctrl Pts',(-2.65479386158097,-2.57881989840821,
1.03793917153882));
#15409=CARTESIAN_POINT('Ctrl Pts',(-2.67298346364342,-2.58233373356339,
0.988766606983592));
#15410=CARTESIAN_POINT('Ctrl Pts',(-2.71546996183929,-2.59054120014066,
0.873911423891086));
#15411=CARTESIAN_POINT('Ctrl Pts',(-2.75019953557524,-2.59874866566371,
0.756186135019429));
#15412=CARTESIAN_POINT('Ctrl Pts',(-2.77716835857481,-2.60695612942142,
0.636738152390488));
#15413=CARTESIAN_POINT('Ctrl Pts',(-2.7902797066403,-2.61094632632634,0.578666501432876));
#15414=CARTESIAN_POINT('Ctrl Pts',(-2.80155751730202,-2.614936522814,0.520187858339262));
#15415=CARTESIAN_POINT('Ctrl Pts',(-2.81100576722147,-2.61892671880269,
0.461434456263184));
#15416=CARTESIAN_POINT('Ctrl Pts',(-2.83257209637234,-2.62803463622678,
0.327325471137989));
#15417=CARTESIAN_POINT('Ctrl Pts',(-2.84462417066588,-2.63714246177211,
0.191708380271717));
#15418=CARTESIAN_POINT('Ctrl Pts',(-2.84720452032045,-2.64625026874975,
0.0559117117292025));
#15419=CARTESIAN_POINT('Ctrl Pts',(-2.84977909096886,-2.65533767768847,
-0.0795808236956612));
#15420=CARTESIAN_POINT('Ctrl Pts',(-2.84292428703749,-2.66442506814257,
-0.215253398492207));
#15421=CARTESIAN_POINT('Ctrl Pts',(-2.8266315877823,-2.67351251293159,-0.349789492086304));
#15422=CARTESIAN_POINT('Ctrl Pts',(-2.81637317564084,-2.67923426305405,
-0.434497782245832));
#15423=CARTESIAN_POINT('Ctrl Pts',(-2.80237222267494,-2.6849560347169,-0.518755526343385));
#15424=CARTESIAN_POINT('Ctrl Pts',(-2.78461630087962,-2.69067784609661,
-0.602231317561455));
#15425=CARTESIAN_POINT('Ctrl Pts',(-2.75885578422968,-2.69897912265177,
-0.723339054705511));
#15426=CARTESIAN_POINT('Ctrl Pts',(-2.72518225862423,-2.70728039666944,
-0.842816999871552));
#15427=CARTESIAN_POINT('Ctrl Pts',(-2.68360003639548,-2.71558166376684,
-0.959480990643439));
#15428=CARTESIAN_POINT('Ctrl Pts',(-2.67635637108904,-2.71702775291864,
-0.979803976216825));
#15429=CARTESIAN_POINT('Ctrl Pts',(-2.66887283467555,-2.71847384186044,
-1.00004159014573));
#15430=CARTESIAN_POINT('Ctrl Pts',(-2.6611496096252,-2.71991993056907,-1.02018760778401));
#15431=CARTESIAN_POINT('Ctrl Pts',(-2.61673255514137,-2.72823653413051,
-1.13604940868169));
#15432=CARTESIAN_POINT('Ctrl Pts',(-2.56438391160144,-2.73655312997981,
-1.24887965301854));
#15433=CARTESIAN_POINT('Ctrl Pts',(-2.50488242176999,-2.74486971370987,
-1.35778164951388));
#15434=CARTESIAN_POINT('Ctrl Pts',(-2.46300472313212,-2.75072300222636,
-1.43442788145216));
#15435=CARTESIAN_POINT('Ctrl Pts',(-2.41758499103118,-2.7565762847396,-1.50912864719515));
#15436=CARTESIAN_POINT('Ctrl Pts',(-2.3689070842741,-2.76242955971315,-1.58158059804684));
#15437=CARTESIAN_POINT('Ctrl Pts',(-2.29156242541089,-2.77172986833818,
-1.69669999811805));
#15438=CARTESIAN_POINT('Ctrl Pts',(-2.20593010819929,-2.78103011048508,
-1.80624681857931));
#15439=CARTESIAN_POINT('Ctrl Pts',(-2.11296872096421,-2.79033034681067,
-1.9091751950852));
#15440=CARTESIAN_POINT('Ctrl Pts',(-2.02106806477434,-2.79952446327627,
-2.01092911273627));
#15441=CARTESIAN_POINT('Ctrl Pts',(-1.92200373022194,-2.80871857405262,
-2.10621564516073));
#15442=CARTESIAN_POINT('Ctrl Pts',(-1.81666548897215,-2.81791273774381,
-2.19399031980656));
#15443=CARTESIAN_POINT('Ctrl Pts',(-1.75453793015004,-2.82333537380425,
-2.24575904308739));
#15444=CARTESIAN_POINT('Ctrl Pts',(-1.69022734883333,-2.8287580282713,-2.29491403170352));
#15445=CARTESIAN_POINT('Ctrl Pts',(-1.62391216664702,-2.83418071316825,
-2.3412334732007));
#15446=CARTESIAN_POINT('Ctrl Pts',(-1.52883304313051,-2.84195546564739,
-2.40764378459746));
#15447=CARTESIAN_POINT('Ctrl Pts',(-1.42964894747358,-2.84973022034248,
-2.46820934176147));
#15448=CARTESIAN_POINT('Ctrl Pts',(-1.32700138290461,-2.85750496714164,
-2.52221476672808));
#15449=CARTESIAN_POINT('Ctrl Pts',(-1.21336288402553,-2.86611219088953,
-2.58200279433791));
#15450=CARTESIAN_POINT('Ctrl Pts',(-1.09547996868788,-2.87471940496007,
-2.63374940496428));
#15451=CARTESIAN_POINT('Ctrl Pts',(-0.974642740719075,-2.88332659563305,
-2.67727993579873));
#15452=CARTESIAN_POINT('Ctrl Pts',(-0.868854144173173,-2.89086187790328,
-2.71538933172979));
#15453=CARTESIAN_POINT('Ctrl Pts',(-0.760802169834941,-2.89839714224074,
-2.74720229870293));
#15454=CARTESIAN_POINT('Ctrl Pts',(-0.651358559006033,-2.90593237943932,
-2.77263384914226));
#15455=CARTESIAN_POINT('Ctrl Pts',(-0.511049236294445,-2.91559273347731,
-2.80523770413774));
#15456=CARTESIAN_POINT('Ctrl Pts',(-0.368294800260247,-2.92525306083563,
-2.82739851538043));
#15457=CARTESIAN_POINT('Ctrl Pts',(-0.22468566984122,-2.93491339754972,
-2.83892488199066));
#15458=CARTESIAN_POINT('Ctrl Pts',(-0.0841848176923486,-2.94436464578452,
-2.85020177174127));
#15459=CARTESIAN_POINT('Ctrl Pts',(0.0571353952658782,-2.95381590297447,
-2.85129956142687));
#15460=CARTESIAN_POINT('Ctrl Pts',(0.197785017350908,-2.96326720286551,
-2.84199026349249));
#15461=CARTESIAN_POINT('Ctrl Pts',(0.269297302826939,-2.9680726480982,-2.83725701813004));
#15462=CARTESIAN_POINT('Ctrl Pts',(0.340636105777945,-2.97287810436972,
-2.82983260933662));
#15463=CARTESIAN_POINT('Ctrl Pts',(0.411603962273926,-2.97768357611561,
-2.81968208523217));
#15464=CARTESIAN_POINT('Ctrl Pts',(0.497282125125452,-2.98348513207562,
-2.80742754775295));
#15465=CARTESIAN_POINT('Ctrl Pts',(0.582386767266939,-2.98928669479688,
-2.79120315094139));
#15466=CARTESIAN_POINT('Ctrl Pts',(0.666528411393449,-2.99508825648647,
-2.77096370899068));
#15467=CARTESIAN_POINT('Ctrl Pts',(0.799366076867762,-3.00424740614358,
-2.73901091977262));
#15468=CARTESIAN_POINT('Ctrl Pts',(0.929802222571363,-3.01340655322936,
-2.69704856763171));
#15469=CARTESIAN_POINT('Ctrl Pts',(1.0565547050704,-3.02256566707968,-2.64593552148088));
#15470=CARTESIAN_POINT('Ctrl Pts',(1.18050383232203,-3.031522210934,-2.59595293071296));
#15471=CARTESIAN_POINT('Ctrl Pts',(1.30092953946802,-3.04047872300668,-2.53722077815605));
#15472=CARTESIAN_POINT('Ctrl Pts',(1.41665920877042,-3.04943517462354,-2.47058258696873));
#15473=CARTESIAN_POINT('Ctrl Pts',(1.54981361231564,-3.05974014637462,-2.39391107607299));
#15474=CARTESIAN_POINT('Ctrl Pts',(1.67693960457707,-3.07004514415773,-2.30667609351077));
#15475=CARTESIAN_POINT('Ctrl Pts',(1.79640033527703,-3.08035016642422,-2.20997267653908));
#15476=CARTESIAN_POINT('Ctrl Pts',(1.91175602400711,-3.09030107609944,-2.11659228951182));
#15477=CARTESIAN_POINT('Ctrl Pts',(2.0199650594349,-3.10025200860431,-2.01438211680193));
#15478=CARTESIAN_POINT('Ctrl Pts',(2.1195166720553,-3.11020296254449,-1.90429782257829));
#15479=CARTESIAN_POINT('Ctrl Pts',(2.15614367154787,-3.11386411453715,-1.86379564202554));
#15480=CARTESIAN_POINT('Ctrl Pts',(2.19159832758418,-3.1175252694314,-1.8222273436528));
#15481=CARTESIAN_POINT('Ctrl Pts',(2.2258037334462,-3.12118642715779,-1.77963979455017));
#15482=CARTESIAN_POINT('Ctrl Pts',(2.2615666211292,-3.1250142891363,-1.73511309776443));
#15483=CARTESIAN_POINT('Ctrl Pts',(2.29594976379294,-3.12884215682671,-1.68948953326672));
#15484=CARTESIAN_POINT('Ctrl Pts',(2.32886296023783,-3.13267002702334,-1.64283210107154));
#15485=CARTESIAN_POINT('Ctrl Pts',(2.41642064644769,-3.14285316004386,-1.51871116330901));
#15486=CARTESIAN_POINT('Ctrl Pts',(2.49357204651819,-3.15303631080089,-1.38727219520211));
#15487=CARTESIAN_POINT('Ctrl Pts',(2.55979938239103,-3.16321941894212,-1.25052854618166));
#15488=CARTESIAN_POINT('Ctrl Pts',(2.62422603598284,-3.17312565436676,-1.1175028764909));
#15489=CARTESIAN_POINT('Ctrl Pts',(2.67831448479832,-3.18303184946147,-0.979458378356245));
#15490=CARTESIAN_POINT('Ctrl Pts',(2.72163477731378,-3.19293794866419,-0.838256249921217));
#15491=CARTESIAN_POINT('Ctrl Pts',(2.77393013709443,-3.20489638642506,-0.667799965359726));
#15492=CARTESIAN_POINT('Ctrl Pts',(2.81063217923236,-3.21685492550503,-0.492454187357721));
#15493=CARTESIAN_POINT('Ctrl Pts',(2.83090292012302,-3.22881349999406,-0.315238782193383));
#15494=CARTESIAN_POINT('Ctrl Pts',(2.84943804737397,-3.23974816198248,-0.153196846811367));
#15495=CARTESIAN_POINT('Ctrl Pts',(2.85423479389205,-3.25068285357602,0.0104093356369592));
#15496=CARTESIAN_POINT('Ctrl Pts',(2.84460655496912,-3.26161752438638,0.17325672336415));
#15497=CARTESIAN_POINT('Ctrl Pts',(2.84370497481946,-3.26264143771307,0.188505615022862));
#15498=CARTESIAN_POINT('Ctrl Pts',(2.84267687832759,-3.26366535085753,0.203747835727151));
#15499=CARTESIAN_POINT('Ctrl Pts',(2.84152168048413,-3.26468926377839,0.218981466195257));
#15500=CARTESIAN_POINT('Ctrl Pts',(2.83942996306458,-3.26654326351079,0.246565009908956));
#15501=CARTESIAN_POINT('Ctrl Pts',(2.83692202091477,-3.26839726499412,0.274113823713482));
#15502=CARTESIAN_POINT('Ctrl Pts',(2.8339950153857,-3.27025126780648,0.301616068458823));
#15503=CARTESIAN_POINT('Ctrl Pts',(2.81452741727389,-3.28258229393223,0.484534290702154));
#15504=CARTESIAN_POINT('Ctrl Pts',(2.77651913214918,-3.2949133788493,0.66538988922194));
#15505=CARTESIAN_POINT('Ctrl Pts',(2.72163883591144,-3.30724439842938,0.840980151964874));
#15506=CARTESIAN_POINT('Ctrl Pts',(2.67832497503693,-3.31697656285171,0.97956344565591));
#15507=CARTESIAN_POINT('Ctrl Pts',(2.62450239319057,-3.32670868657539,1.11486715825269));
#15508=CARTESIAN_POINT('Ctrl Pts',(2.56100487279523,-3.33644070857623,1.24533559631229));
#15509=CARTESIAN_POINT('Ctrl Pts',(2.47221764009378,-3.35004878802035,1.42776683926587));
#15510=CARTESIAN_POINT('Ctrl Pts',(2.36434093956612,-3.36365705283171,1.60110913754079));
#15511=CARTESIAN_POINT('Ctrl Pts',(2.23940451281916,-3.37726534765327,1.76109550492112));
#15512=CARTESIAN_POINT('Ctrl Pts',(2.14585736922928,-3.38745466667601,1.88088657043688));
#15513=CARTESIAN_POINT('Ctrl Pts',(2.04274602578603,-3.39764400252361,1.99318890306528));
#15514=CARTESIAN_POINT('Ctrl Pts',(1.93092652160215,-3.40783328997986,2.09619244540513));
#15515=CARTESIAN_POINT('Ctrl Pts',(1.92961400303739,-3.40795289012516,2.09740148369003));
#15516=CARTESIAN_POINT('Ctrl Pts',(1.92830028473655,-3.4080724902638,2.09860924062003));
#15517=CARTESIAN_POINT('Ctrl Pts',(1.92698536963071,-3.40819209039566,2.09981571492913));
#15518=CARTESIAN_POINT('Ctrl Pts',(1.78095071869536,-3.42147489734707,2.23380691619397));
#15519=CARTESIAN_POINT('Ctrl Pts',(1.62042629665332,-3.43475778445623,2.35173263647907));
#15520=CARTESIAN_POINT('Ctrl Pts',(1.44955001995471,-3.44804061145149,2.45204164123285));
#15521=CARTESIAN_POINT('Ctrl Pts',(1.31274498852354,-3.45867495812436,2.53234990176673));
#15522=CARTESIAN_POINT('Ctrl Pts',(1.1693033470129,-3.46930926626579,2.60136638804764));
#15523=CARTESIAN_POINT('Ctrl Pts',(1.02132469790409,-3.47994346389266,2.65829384092901));
#15524=CARTESIAN_POINT('Ctrl Pts',(0.85476358086714,-3.49191305441258,2.72236997758179));
#15525=CARTESIAN_POINT('Ctrl Pts',(0.682161769008386,-3.50388279843517,
2.7712376313902));
#15526=CARTESIAN_POINT('Ctrl Pts',(0.506544247507313,-3.51585258313136,
2.80358587734168));
#15527=CARTESIAN_POINT('Ctrl Pts',(0.361966225971356,-3.52570676951775,
2.83021673603875));
#15528=CARTESIAN_POINT('Ctrl Pts',(0.215345706367376,-3.5355609834706,2.8456519610467));
#15529=CARTESIAN_POINT('Ctrl Pts',(0.0683885252654139,-3.54541516203575,
2.84917935721609));
#15530=CARTESIAN_POINT('Ctrl Pts',(0.0371714470076327,-3.54750841573814,
2.84992865712399));
#15531=CARTESIAN_POINT('Ctrl Pts',(0.00593921664234942,-3.54960166784371,
2.85014070352172));
#15532=CARTESIAN_POINT('Ctrl Pts',(-0.0252914674637119,-3.55169491774903,
2.84982099350694));
#15533=CARTESIAN_POINT('Ctrl Pts',(-0.185879903078349,-3.56245842605082,
2.84817704197036));
#15534=CARTESIAN_POINT('Ctrl Pts',(-0.34620802968348,-3.57322195383387,
2.83247981270469));
#15535=CARTESIAN_POINT('Ctrl Pts',(-0.504125026400352,-3.58398545793961,
2.8035682722057));
#15536=CARTESIAN_POINT('Ctrl Pts',(-0.670268236132065,-3.59530965455724,
2.77315067158857));
#15537=CARTESIAN_POINT('Ctrl Pts',(-0.833743800644653,-3.60663382496655,
2.72810615902489));
#15538=CARTESIAN_POINT('Ctrl Pts',(-0.992059497535025,-3.61795791890694,
2.66935668768567));
#15539=CARTESIAN_POINT('Ctrl Pts',(-1.0176358187225,-3.61978735635039,2.65986555460108));
#15540=CARTESIAN_POINT('Ctrl Pts',(-1.04307747231,-3.62161679179806,2.65001662193548));
#15541=CARTESIAN_POINT('Ctrl Pts',(-1.06837394293086,-3.62344622503802,
2.63981365250559));
#15542=CARTESIAN_POINT('Ctrl Pts',(-1.20691714936607,-3.63346562856756,
2.58393423275716));
#15543=CARTESIAN_POINT('Ctrl Pts',(-1.34129998177926,-3.64348512800569,
2.51735235049409));
#15544=CARTESIAN_POINT('Ctrl Pts',(-1.46963398238972,-3.65350466767422,
2.4406713441377));
#15545=CARTESIAN_POINT('Ctrl Pts',(-1.59554739801365,-3.66333522276206,
2.36543666449018));
#15546=CARTESIAN_POINT('Ctrl Pts',(-1.71563678789023,-3.67316581657696,
2.28048082016419));
#15547=CARTESIAN_POINT('Ctrl Pts',(-1.82813144995633,-3.68299639653218,
2.18642068265436));
#15548=CARTESIAN_POINT('Ctrl Pts',(-1.87467292357269,-3.687063519978,2.14750597036611));
#15549=CARTESIAN_POINT('Ctrl Pts',(-1.91991470040694,-3.69113064105153,
2.10703343267552));
#15550=CARTESIAN_POINT('Ctrl Pts',(-1.96379020164121,-3.69519775602884,
2.0651174806424));
#15551=CARTESIAN_POINT('Ctrl Pts',(-2.06986645150067,-3.70503067627827,
1.96377876368458));
#15552=CARTESIAN_POINT('Ctrl Pts',(-2.16785687873356,-3.7148635706403,1.85410545128513));
#15553=CARTESIAN_POINT('Ctrl Pts',(-2.25697365342708,-3.72469644251745,
1.73763937962582));
#15554=CARTESIAN_POINT('Ctrl Pts',(-2.34933317921239,-3.73488710961468,
1.61693537989596));
#15555=CARTESIAN_POINT('Ctrl Pts',(-2.4321623802172,-3.74507775256094,1.48893434178596));
#15556=CARTESIAN_POINT('Ctrl Pts',(-2.50455081037485,-3.75526837514386,
1.35530862510515));
#15557=CARTESIAN_POINT('Ctrl Pts',(-2.53220835593805,-3.7591619201177,1.30425406653183));
#15558=CARTESIAN_POINT('Ctrl Pts',(-2.55834136549607,-3.76305546211892,
1.25237805780557));
#15559=CARTESIAN_POINT('Ctrl Pts',(-2.58289742121862,-3.76694900135878,
1.19977273255586));
#15560=CARTESIAN_POINT('Ctrl Pts',(-2.6401218230586,-3.77602234182351,1.07718349000714));
#15561=CARTESIAN_POINT('Ctrl Pts',(-2.68884667112697,-3.78509574169171,
0.950484867996509));
#15562=CARTESIAN_POINT('Ctrl Pts',(-2.72829656318992,-3.79416917286518,
0.8209674215693));
#15563=CARTESIAN_POINT('Ctrl Pts',(-2.76657077212904,-3.80297219823148,
0.695309845677688));
#15564=CARTESIAN_POINT('Ctrl Pts',(-2.79611424068812,-3.81177525306492,
0.567000077065634));
#15565=CARTESIAN_POINT('Ctrl Pts',(-2.81626037388312,-3.82057831170534,
0.437238500388076));
#15566=CARTESIAN_POINT('Ctrl Pts',(-2.83008489722928,-3.82661907836333,
0.348194517165623));
#15567=CARTESIAN_POINT('Ctrl Pts',(-2.83948525764255,-3.83265984681399,
0.258467350941794));
#15568=CARTESIAN_POINT('Ctrl Pts',(-2.84454876096055,-3.83870060876577,
0.168492053738068));
#15569=CARTESIAN_POINT('Ctrl Pts',(-2.85240049093481,-3.84806772649144,
0.0289717071264769));
#15570=CARTESIAN_POINT('Ctrl Pts',(-2.84982609907032,-3.85743478090333,
-0.111064582497238));
#15571=CARTESIAN_POINT('Ctrl Pts',(-2.83719044067114,-3.86680180880028,
-0.250186399393045));
#15572=CARTESIAN_POINT('Ctrl Pts',(-2.82423457679865,-3.87640621044592,
-0.392833760096772));
#15573=CARTESIAN_POINT('Ctrl Pts',(-2.80070099369802,-3.88601058421576,
-0.534520981583524));
#15574=CARTESIAN_POINT('Ctrl Pts',(-2.76692914184924,-3.8956149697777,-0.673711919111808));
#15575=CARTESIAN_POINT('Ctrl Pts',(-2.74953893645332,-3.90056057472622,
-0.745385779452855));
#15576=CARTESIAN_POINT('Ctrl Pts',(-2.72943314510381,-3.90550618280147,
-0.81639771099666));
#15577=CARTESIAN_POINT('Ctrl Pts',(-2.70665285141107,-3.91045179941958,
-0.886536819547011));
#15578=CARTESIAN_POINT('Ctrl Pts',(-2.66722359737821,-3.91901191618605,
-1.00793704229967));
#15579=CARTESIAN_POINT('Ctrl Pts',(-2.61973805017892,-3.92757206551366,
-1.12684088972418));
#15580=CARTESIAN_POINT('Ctrl Pts',(-2.56442927732012,-3.93613223517365,
-1.24198315809337));
#15581=CARTESIAN_POINT('Ctrl Pts',(-2.51698367917274,-3.94347541689273,
-1.34075580323537));
#15582=CARTESIAN_POINT('Ctrl Pts',(-2.46378211843104,-3.95081861357388,
-1.43675993538346));
#15583=CARTESIAN_POINT('Ctrl Pts',(-2.40500101984259,-3.95816181749765,
-1.52920570699362));
#15584=CARTESIAN_POINT('Ctrl Pts',(-2.34085127496968,-3.96617569729187,
-1.63009481600624));
#15585=CARTESIAN_POINT('Ctrl Pts',(-2.27005625443048,-3.97418958571212,
-1.72674501095433));
#15586=CARTESIAN_POINT('Ctrl Pts',(-2.19345610618758,-3.98220347272476,
-1.81851953916284));
#15587=CARTESIAN_POINT('Ctrl Pts',(-2.10614697227237,-3.99133773095294,
-1.92312448781064));
#15588=CARTESIAN_POINT('Ctrl Pts',(-2.01131854196274,-4.00047190003977,
-2.02138198284188));
#15589=CARTESIAN_POINT('Ctrl Pts',(-1.91008620673602,-4.00960604015026,
-2.11252412289686));
#15590=CARTESIAN_POINT('Ctrl Pts',(-1.80722638330456,-4.01888702766141,
-2.20513153348582));
#15591=CARTESIAN_POINT('Ctrl Pts',(-1.6977541622283,-4.02816798525704,-2.29039382549714));
#15592=CARTESIAN_POINT('Ctrl Pts',(-1.58279871002626,-4.03744897605077,
-2.36747157972989));
#15593=CARTESIAN_POINT('Ctrl Pts',(-1.5146519473948,-4.04295084189958,-2.41316405730487));
#15594=CARTESIAN_POINT('Ctrl Pts',(-1.44457753941025,-4.04845271941498,
-2.45597958821667));
#15595=CARTESIAN_POINT('Ctrl Pts',(-1.37280618311532,-4.05395462174532,
-2.49573591232744));
#15596=CARTESIAN_POINT('Ctrl Pts',(-1.2646045336739,-4.0622492247449,-2.55567207720687));
#15597=CARTESIAN_POINT('Ctrl Pts',(-1.15246138914533,-4.07054384096858,
-2.60869580600677));
#15598=CARTESIAN_POINT('Ctrl Pts',(-1.03730936249408,-4.07883846677113,
-2.6540787781793));
#15599=CARTESIAN_POINT('Ctrl Pts',(-0.959063735452324,-4.08447465239349,
-2.68491643877395));
#15600=CARTESIAN_POINT('Ctrl Pts',(-0.879429643629576,-4.09011084243859,
-2.71222696854328));
#15601=CARTESIAN_POINT('Ctrl Pts',(-0.798706481232868,-4.09574703576282,
-2.73579384397682));
#15602=CARTESIAN_POINT('Ctrl Pts',(-0.680102865998873,-4.10402809022803,
-2.77041979944237));
#15603=CARTESIAN_POINT('Ctrl Pts',(-0.559148320148908,-4.11230915177202,
-2.79696178855869));
#15604=CARTESIAN_POINT('Ctrl Pts',(-0.437015001412886,-4.12059021676748,
-2.8155024676079));
#15605=CARTESIAN_POINT('Ctrl Pts',(-0.411863282802995,-4.12229559101516,
-2.81932067174014));
#15606=CARTESIAN_POINT('Ctrl Pts',(-0.386661587666493,-4.12400096540922,
-2.82279971732075));
#15607=CARTESIAN_POINT('Ctrl Pts',(-0.361420159933744,-4.12570633991797,
-2.82594059869468));
#15608=CARTESIAN_POINT('Ctrl Pts',(-0.227420491876474,-4.13475969539792,
-2.84261465794239));
#15609=CARTESIAN_POINT('Ctrl Pts',(-0.0922757684614264,-4.14381295104456,
-2.84976621078605));
#15610=CARTESIAN_POINT('Ctrl Pts',(0.0427129671981117,-4.15286617971873,
-2.8475412505536));
#15611=CARTESIAN_POINT('Ctrl Pts',(0.178702659926457,-4.16198653912936,
-2.84529979198401));
#15612=CARTESIAN_POINT('Ctrl Pts',(0.314535306910664,-4.17110687116603,
-2.83354221057195));
#15613=CARTESIAN_POINT('Ctrl Pts',(0.448884946130907,-4.18022725032238,
-2.8123658974596));
#15614=CARTESIAN_POINT('Ctrl Pts',(0.533489004344512,-4.18597063075535,
-2.7990305283607));
#15615=CARTESIAN_POINT('Ctrl Pts',(0.617504980397791,-4.19171402987412,
-2.78195903079779));
#15616=CARTESIAN_POINT('Ctrl Pts',(0.700599140013145,-4.19745746628173,
-2.76116539599247));
#15617=CARTESIAN_POINT('Ctrl Pts',(0.819351038141763,-4.20566555188416,
-2.73144870334458));
#15618=CARTESIAN_POINT('Ctrl Pts',(0.93627704500667,-4.21387363880933,-2.69410983378928));
#15619=CARTESIAN_POINT('Ctrl Pts',(1.05022883861694,-4.22208172614931,-2.64922295283315));
#15620=CARTESIAN_POINT('Ctrl Pts',(1.10229703136876,-4.22583226188203,-2.6287127116548));
#15621=CARTESIAN_POINT('Ctrl Pts',(1.15374432733471,-4.22958279770134,-2.60662725371738));
#15622=CARTESIAN_POINT('Ctrl Pts',(1.20446204849237,-4.23333333352066,-2.58297719187402));
#15623=CARTESIAN_POINT('Ctrl Pts',(1.31545832066639,-4.24154142105096,-2.53121877999393));
#15624=CARTESIAN_POINT('Ctrl Pts',(1.42295823404889,-4.24974950858126,-2.4719636913944));
#15625=CARTESIAN_POINT('Ctrl Pts',(1.52615212050412,-4.25795759520368,-2.40602519583505));
#15626=CARTESIAN_POINT('Ctrl Pts',(1.57330468230345,-4.26170813048258,-2.37589580451528));
#15627=CARTESIAN_POINT('Ctrl Pts',(1.61955860008734,-4.26545866557193,-2.34437162040238));
#15628=CARTESIAN_POINT('Ctrl Pts',(1.66483896157514,-4.2692092003851,-2.31153298290008));
#15629=CARTESIAN_POINT('Ctrl Pts',(1.77466818054188,-4.27830626356444,-2.23188163316914));
#15630=CARTESIAN_POINT('Ctrl Pts',(1.87883199843095,-4.2874032331951,-2.1444586779963));
#15631=CARTESIAN_POINT('Ctrl Pts',(1.97643042794329,-4.29650018319877,-2.05023587971271));
#15632=CARTESIAN_POINT('Ctrl Pts',(2.07391017921323,-4.3055860714462,-1.95612765495402));
#15633=CARTESIAN_POINT('Ctrl Pts',(2.16484137488291,-4.31467194011433,-1.85523520039081));
#15634=CARTESIAN_POINT('Ctrl Pts',(2.24829369710724,-4.32375786285549,-1.74848840006571));
#15635=CARTESIAN_POINT('Ctrl Pts',(2.30096046759489,-4.32949198977877,-1.68112048167632));
#15636=CARTESIAN_POINT('Ctrl Pts',(2.35064778296174,-4.33522613823866,-1.61142013221164));
#15637=CARTESIAN_POINT('Ctrl Pts',(2.39711249291075,-4.34096032674836,-1.53961569740268));
#15638=CARTESIAN_POINT('Ctrl Pts',(2.46421481110792,-4.3492413930114,-1.43591884794842));
#15639=CARTESIAN_POINT('Ctrl Pts',(2.52460350404338,-4.35752245657002,-1.32781167233767));
#15640=CARTESIAN_POINT('Ctrl Pts',(2.5774530717427,-4.36580351379685,-1.2161327212669));
#15641=CARTESIAN_POINT('Ctrl Pts',(2.58833673124962,-4.36750888644488,-1.19313393943277));
#15642=CARTESIAN_POINT('Ctrl Pts',(2.59890079988213,-4.36921425882437,-1.16998378268028));
#15643=CARTESIAN_POINT('Ctrl Pts',(2.60913830161044,-4.37091963090365,-1.14668972393339));
#15644=CARTESIAN_POINT('Ctrl Pts',(2.65893175317248,-4.37921426804059,-1.03339141965186));
#15645=CARTESIAN_POINT('Ctrl Pts',(2.70099558254949,-4.38750889807554,-0.916687593696909));
#15646=CARTESIAN_POINT('Ctrl Pts',(2.73525327248987,-4.39580351736332,-0.79775517172945));
#15647=CARTESIAN_POINT('Ctrl Pts',(2.75853132072395,-4.40143969855944,-0.716940771810146));
#15648=CARTESIAN_POINT('Ctrl Pts',(2.77820618530874,-4.40707587479338,-0.63509785969229));
#15649=CARTESIAN_POINT('Ctrl Pts',(2.79426743213858,-4.41271204492151,-0.552597573438769));
#15650=CARTESIAN_POINT('Ctrl Pts',(2.82068044144347,-4.42198082807486,-0.416924368764449));
#15651=CARTESIAN_POINT('Ctrl Pts',(2.83734960329111,-4.43124954080225,-0.279360307421618));
#15652=CARTESIAN_POINT('Ctrl Pts',(2.84422306735829,-4.44051824596736,-0.141307961682125));
#15653=CARTESIAN_POINT('Ctrl Pts',(2.8510260385497,-4.44969189314202,-0.00467145324992427));
#15654=CARTESIAN_POINT('Ctrl Pts',(2.84823318955168,-4.45886553290869,0.132444642262169));
#15655=CARTESIAN_POINT('Ctrl Pts',(2.83574436772078,-4.46803922621668,0.268682484355037));
#15656=CARTESIAN_POINT('Ctrl Pts',(2.82829134876046,-4.47351385873898,0.349985847793197));
#15657=CARTESIAN_POINT('Ctrl Pts',(2.81738424752888,-4.47898851032953,0.430976379224427));
#15658=CARTESIAN_POINT('Ctrl Pts',(2.80299319512765,-4.48446319394224,0.511363033623647));
#15659=CARTESIAN_POINT('Ctrl Pts',(2.78192745396434,-4.49247708095487,0.629033681144406));
#15660=CARTESIAN_POINT('Ctrl Pts',(2.7533952712281,-4.50049096937513,0.745391361015317));
#15661=CARTESIAN_POINT('Ctrl Pts',(2.71734439106664,-4.50850484916934,0.859383185828289));
#15662=CARTESIAN_POINT('Ctrl Pts',(2.67883587937714,-4.51706504471385,0.981145969390209));
#15663=CARTESIAN_POINT('Ctrl Pts',(2.63174833745007,-4.52562523041615,1.10020817320856));
#15664=CARTESIAN_POINT('Ctrl Pts',(2.57686399773131,-4.53418539404755,1.21555311043328));
#15665=CARTESIAN_POINT('Ctrl Pts',(2.52978249162659,-4.54152857059544,1.31449961127346));
#15666=CARTESIAN_POINT('Ctrl Pts',(2.4769646669258,-4.54887173090188,1.4107105849836));
#15667=CARTESIAN_POINT('Ctrl Pts',(2.41892952084411,-4.55621486724742,1.50356149313978));
#15668=CARTESIAN_POINT('Ctrl Pts',(2.34301936580719,-4.56581971286395,1.62501077533051));
#15669=CARTESIAN_POINT('Ctrl Pts',(2.25810592177126,-4.57542452625917,1.74085044412127));
#15670=CARTESIAN_POINT('Ctrl Pts',(2.16516849635887,-4.58502934710639,1.84985007122675));
#15671=CARTESIAN_POINT('Ctrl Pts',(2.07411849119096,-4.59443910839358,1.95663607877125));
#15672=CARTESIAN_POINT('Ctrl Pts',(1.97536620097115,-4.60384887683315,2.05685793011607));
#15673=CARTESIAN_POINT('Ctrl Pts',(1.86979798952804,-4.61325868973011,2.14932401144856));
#15674=CARTESIAN_POINT('Ctrl Pts',(1.81479773992408,-4.61816113196139,2.19749814913326));
#15675=CARTESIAN_POINT('Ctrl Pts',(1.75794693188286,-4.62306358625989,2.24356645717859));
#15676=CARTESIAN_POINT('Ctrl Pts',(1.699368297219,-4.62796605790107,2.28735537598812));
#15677=CARTESIAN_POINT('Ctrl Pts',(1.62718846358363,-4.63400681985281,2.34131151362912));
#15678=CARTESIAN_POINT('Ctrl Pts',(1.55241103130075,-4.64004758830341,2.39178593047225));
#15679=CARTESIAN_POINT('Ctrl Pts',(1.47531315044321,-4.64608835496136,2.43843210031673));
#15680=CARTESIAN_POINT('Ctrl Pts',(1.35950914751608,-4.65516182043095,2.5084964539556));
#15681=CARTESIAN_POINT('Ctrl Pts',(1.23846929110902,-4.66423528185609,2.56992132487734));
#15682=CARTESIAN_POINT('Ctrl Pts',(1.11366996284203,-4.67330871113862,2.62242170807228));
#15683=CARTESIAN_POINT('Ctrl Pts',(0.992589896059362,-4.68211173467034,
2.67335747825334));
#15684=CARTESIAN_POINT('Ctrl Pts',(0.867972296334286,-4.69091472794669,
2.71589279995554));
#15685=CARTESIAN_POINT('Ctrl Pts',(0.741175224670663,-4.69971766530755,
2.74981326359758));
#15686=CARTESIAN_POINT('Ctrl Pts',(0.594188688536139,-4.70992226430581,
2.78913476676327));
#15687=CARTESIAN_POINT('Ctrl Pts',(0.444077504545696,-4.72012688227234,
2.81694165833229));
#15688=CARTESIAN_POINT('Ctrl Pts',(0.292716472016533,-4.73033152301031,
2.83287479822956));
#15689=CARTESIAN_POINT('Ctrl Pts',(0.14629116648403,-4.74020340094969,2.8482883748851));
#15690=CARTESIAN_POINT('Ctrl Pts',(-0.00130505071413023,-4.75007530019963,
2.8525899300837));
#15691=CARTESIAN_POINT('Ctrl Pts',(-0.148370980131912,-4.75994722420332,
2.84540659185951));
#15692=CARTESIAN_POINT('Ctrl Pts',(-0.205585286096275,-4.76378778253413,
2.84261199685963));
#15693=CARTESIAN_POINT('Ctrl Pts',(-0.262719192545857,-4.76762834461144,
2.83807863098206));
#15694=CARTESIAN_POINT('Ctrl Pts',(-0.319671760795388,-4.77146891063799,
2.83178250052298));
#15695=CARTESIAN_POINT('Ctrl Pts',(-0.37998387149061,-4.77553602561533,
2.82511497122851));
#15696=CARTESIAN_POINT('Ctrl Pts',(-0.440068487676707,-4.77960314668888,
2.81647300524789));
#15697=CARTESIAN_POINT('Ctrl Pts',(-0.499795169357878,-4.78367027013473,
2.8058340629029));
#15698=CARTESIAN_POINT('Ctrl Pts',(-0.646934880785383,-4.79368983514851,
2.77962448851381));
#15699=CARTESIAN_POINT('Ctrl Pts',(-0.791900799561659,-4.80370941455995,
2.74129173439158));
#15700=CARTESIAN_POINT('Ctrl Pts',(-0.932987708459681,-4.81372895269081,
2.69185259721203));
#15701=CARTESIAN_POINT('Ctrl Pts',(-1.07141349208279,-4.82355950627043,
2.6433459614144));
#15702=CARTESIAN_POINT('Ctrl Pts',(-1.20610416138044,-4.833390020112,2.584148780273));
#15703=CARTESIAN_POINT('Ctrl Pts',(-1.33547704634397,-4.84322044162881,
2.51526142986738));
#15704=CARTESIAN_POINT('Ctrl Pts',(-1.48479827299402,-4.85456664141242,
2.43575215969737));
#15705=CARTESIAN_POINT('Ctrl Pts',(-1.62728010749542,-4.86591292611561,
2.34321424573768));
#15706=CARTESIAN_POINT('Ctrl Pts',(-1.7606072822343,-4.87725924518256,2.23897728299655));
#15707=CARTESIAN_POINT('Ctrl Pts',(-1.88728409303887,-4.88803960947504,
2.13993966344253));
#15708=CARTESIAN_POINT('Ctrl Pts',(-2.00569749096051,-4.89882000478868,
2.03034012677808));
#15709=CARTESIAN_POINT('Ctrl Pts',(-2.11382090529319,-4.90960038776174,
1.91129521590937));
#15710=CARTESIAN_POINT('Ctrl Pts',(-2.13177852458187,-4.91139084188688,
1.89152370572511));
#15711=CARTESIAN_POINT('Ctrl Pts',(-2.14945219484852,-4.91318129567162,
1.87149161408109));
#15712=CARTESIAN_POINT('Ctrl Pts',(-2.16683249404356,-4.9149717489173,1.85120401255983));
#15713=CARTESIAN_POINT('Ctrl Pts',(-2.18715210290924,-4.91706499882263,
1.82748542618174));
#15714=CARTESIAN_POINT('Ctrl Pts',(-2.20706535664628,-4.9191582509282,1.80342384886703));
#15715=CARTESIAN_POINT('Ctrl Pts',(-2.22655731073033,-4.9212515046306,1.77902853884047));
#15716=CARTESIAN_POINT('Ctrl Pts',(-2.33801743056546,-4.93322127982647,
1.63952974014388));
#15717=CARTESIAN_POINT('Ctrl Pts',(-2.43569777707777,-4.94519110723601,
1.48911776930381));
#15718=CARTESIAN_POINT('Ctrl Pts',(-2.5186153379613,-4.95716087402997,1.33095551518211));
#15719=CARTESIAN_POINT('Ctrl Pts',(-2.58687764345666,-4.96701504567819,
1.20074763166928));
#15720=CARTESIAN_POINT('Ctrl Pts',(-2.64513519268278,-4.97686917624427,
1.0652876964692));
#15721=CARTESIAN_POINT('Ctrl Pts',(-2.69286608630087,-4.98672320277401,
0.926338234405749));
#15722=CARTESIAN_POINT('Ctrl Pts',(-2.75720448791769,-5.00000584360378,
0.739042635747796));
#15723=CARTESIAN_POINT('Ctrl Pts',(-2.80254615611727,-5.01328865684996,
0.545045070540891));
#15724=CARTESIAN_POINT('Ctrl Pts',(-2.82744790125318,-5.02657150224111,
0.348481808485192));
#15725=CARTESIAN_POINT('Ctrl Pts',(-2.84738445471526,-5.03720586364123,
0.191111553458274));
#15726=CARTESIAN_POINT('Ctrl Pts',(-2.85421898098582,-5.04784024564545,
0.0320971413027112));
#15727=CARTESIAN_POINT('Ctrl Pts',(-2.84719447964139,-5.05847457627068,
-0.126420910195643));
#15728=CARTESIAN_POINT('Ctrl Pts',(-2.84711547783896,-5.05859417640254,
-0.128203700342931));
#15729=CARTESIAN_POINT('Ctrl Pts',(-2.8470347242005,-5.05871377654117,-0.129986398137237));
#15730=CARTESIAN_POINT('Ctrl Pts',(-2.84695221781174,-5.05883337668647,
-0.131769000519424));
#15731=CARTESIAN_POINT('Ctrl Pts',(-2.83756453871079,-5.07244162934965,
-0.334595707407065));
#15732=CARTESIAN_POINT('Ctrl Pts',(-2.80548826042884,-5.08604996832765,
-0.536183502277633));
#15733=CARTESIAN_POINT('Ctrl Pts',(-2.75271150410846,-5.09965823826323,
-0.732204056437572));
#15734=CARTESIAN_POINT('Ctrl Pts',(-2.71319448789317,-5.10984753865225,
-0.878976006010336));
#15735=CARTESIAN_POINT('Ctrl Pts',(-2.66207125303721,-5.12003680033345,
-1.02262775397972));
#15736=CARTESIAN_POINT('Ctrl Pts',(-2.60016461395293,-5.1302259580906,-1.16135726039429));
#15737=CARTESIAN_POINT('Ctrl Pts',(-2.52524568289888,-5.14255679721866,
-1.32924662541192));
#15738=CARTESIAN_POINT('Ctrl Pts',(-2.43439483816887,-5.15488779965095,
-1.49022775634066));
#15739=CARTESIAN_POINT('Ctrl Pts',(-2.32895182834645,-5.16721884125924,
-1.64096625492276));
#15740=CARTESIAN_POINT('Ctrl Pts',(-2.24573172623983,-5.17695102306484,
-1.75993548071144));
#15741=CARTESIAN_POINT('Ctrl Pts',(-2.15342339325781,-5.18668322927331,
-1.87252384289964));
#15742=CARTESIAN_POINT('Ctrl Pts',(-2.05270819500149,-5.19641539886041,
-1.9770910616754));
#15743=CARTESIAN_POINT('Ctrl Pts',(-2.0335216961287,-5.19826940167276,-1.99701138015669));
#15744=CARTESIAN_POINT('Ctrl Pts',(-2.01403015453902,-5.20012340315607,
-2.01664061147923));
#15745=CARTESIAN_POINT('Ctrl Pts',(-1.99424446419597,-5.20197740288845,
-2.03597332011536));
#15746=CARTESIAN_POINT('Ctrl Pts',(-1.87755085247301,-5.21291206936477,
-2.14999530044671));
#15747=CARTESIAN_POINT('Ctrl Pts',(-1.75079332881031,-5.22384676134255,
-2.25354437627423));
#15748=CARTESIAN_POINT('Ctrl Pts',(-1.61619727332964,-5.23478142843354,
-2.34565521913265));
#15749=CARTESIAN_POINT('Ctrl Pts',(-1.4742672465223,-5.24631191190731,-2.44278506702792));
#15750=CARTESIAN_POINT('Ctrl Pts',(-1.32362032921175,-5.25784236770832,
-2.52719705812083));
#15751=CARTESIAN_POINT('Ctrl Pts',(-1.16681718870844,-5.26937273675464,
-2.59773035429892));
#15752=CARTESIAN_POINT('Ctrl Pts',(-1.14707129845689,-5.27082473191888,
-2.60661246419125));
#15753=CARTESIAN_POINT('Ctrl Pts',(-1.12722773442568,-5.27227672570737,
-2.61527444208103));
#15754=CARTESIAN_POINT('Ctrl Pts',(-1.10729157078743,-5.27372871800215,
-2.62371392855201));
#15755=CARTESIAN_POINT('Ctrl Pts',(-0.967477248542152,-5.2839116861139,
-2.68290089663921));
#15756=CARTESIAN_POINT('Ctrl Pts',(-0.822904805739579,-5.29409475555286,
-2.73122652109907));
#15757=CARTESIAN_POINT('Ctrl Pts',(-0.675423581781764,-5.30427786596671,
-2.76774962167252));
#15758=CARTESIAN_POINT('Ctrl Pts',(-0.531952285489216,-5.31418410360266,
-2.80327968064053));
#15759=CARTESIAN_POINT('Ctrl Pts',(-0.385729529005817,-5.3240903800156,
-2.82763991308817));
#15760=CARTESIAN_POINT('Ctrl Pts',(-0.238481853495246,-5.33399663964339,
-2.84000464883967));
#15761=CARTESIAN_POINT('Ctrl Pts',(-0.181583991961912,-5.33782450984006,
-2.84478249691263));
#15762=CARTESIAN_POINT('Ctrl Pts',(-0.124533255816757,-5.34165237753051,
-2.84776974350696));
#15763=CARTESIAN_POINT('Ctrl Pts',(-0.0674358860842899,-5.34548023950904,
-2.84899499112165));
#15764=CARTESIAN_POINT('Ctrl Pts',(0.0804325551778038,-5.3553934804654,
-2.85216808746204));
#15765=CARTESIAN_POINT('Ctrl Pts',(0.228462621505615,-5.36530670065781,
-2.84352538719917));
#15766=CARTESIAN_POINT('Ctrl Pts',(0.374965744204218,-5.37521989870767,
-2.82362224019619));
#15767=CARTESIAN_POINT('Ctrl Pts',(0.527029781898301,-5.38550937850958,
-2.80296361640482));
#15768=CARTESIAN_POINT('Ctrl Pts',(0.677450029835101,-5.39579883445611,
-2.77017343020061));
#15769=CARTESIAN_POINT('Ctrl Pts',(0.824346177097707,-5.40608826500567,
-2.7258178741885));
#15770=CARTESIAN_POINT('Ctrl Pts',(0.877374657186616,-5.40980267735202,
-2.70980582919854));
#15771=CARTESIAN_POINT('Ctrl Pts',(0.929943866829867,-5.41351708638873,
-2.69228613387777));
#15772=CARTESIAN_POINT('Ctrl Pts',(0.98196507546841,-5.4172314920433,-2.67328379028232));
#15773=CARTESIAN_POINT('Ctrl Pts',(1.11023950482274,-5.42639051157012,-2.62642761671593));
#15774=CARTESIAN_POINT('Ctrl Pts',(1.23533711721485,-5.43554959431835,-2.57049493875236));
#15775=CARTESIAN_POINT('Ctrl Pts',(1.35576092762186,-5.44470870962387,-2.50586711172746));
#15776=CARTESIAN_POINT('Ctrl Pts',(1.47352135254951,-5.45366525490087,-2.44266864336079));
#15777=CARTESIAN_POINT('Ctrl Pts',(1.58681131404656,-5.46262183131094,-2.37115588388267));
#15778=CARTESIAN_POINT('Ctrl Pts',(1.69424514700893,-5.4715784101799,-2.29173152475888));
#15779=CARTESIAN_POINT('Ctrl Pts',(1.76383466535031,-5.47737997186946,-2.24028494835374));
#15780=CARTESIAN_POINT('Ctrl Pts',(1.83096748386614,-5.48318153459071,-2.18551985140271));
#15781=CARTESIAN_POINT('Ctrl Pts',(1.89542786570679,-5.48898309055072,-2.1277636357077));
#15782=CARTESIAN_POINT('Ctrl Pts',(1.99996535344416,-5.49839166164059,-2.03409851121464));
#15783=CARTESIAN_POINT('Ctrl Pts',(2.09741321270494,-5.50780017341223,-1.93262981881011));
#15784=CARTESIAN_POINT('Ctrl Pts',(2.18701354397179,-5.51720865915534,-1.82464990341988));
#15785=CARTESIAN_POINT('Ctrl Pts',(2.27899284570153,-5.52686694877045,-1.71380302285589));
#15786=CARTESIAN_POINT('Ctrl Pts',(2.36270322802092,-5.53652521095654,-1.59609363458982));
#15787=CARTESIAN_POINT('Ctrl Pts',(2.43729095147334,-5.54618348172593,-1.47287733500589));
#15788=CARTESIAN_POINT('Ctrl Pts',(2.47474798900839,-5.55103374654147,-1.41099962450852));
#15789=CARTESIAN_POINT('Ctrl Pts',(2.50990375352354,-5.55588401352164,-1.34773254351142));
#15790=CARTESIAN_POINT('Ctrl Pts',(2.54264596413126,-5.56073428722735,-1.28324507982158));
#15791=CARTESIAN_POINT('Ctrl Pts',(2.60074923441848,-5.56934142641736,-1.16880770789828));
#15792=CARTESIAN_POINT('Ctrl Pts',(2.65130641309992,-5.5779486010165,-1.05040875527548));
#15793=CARTESIAN_POINT('Ctrl Pts',(2.69358203153906,-5.58655579730455,-0.929126797966435));
#15794=CARTESIAN_POINT('Ctrl Pts',(2.73059279732476,-5.59409108449017,-0.822948857069878));
#15795=CARTESIAN_POINT('Ctrl Pts',(2.76125653093975,-5.60162638829895,-0.714562292579616));
#15796=CARTESIAN_POINT('Ctrl Pts',(2.78510865337264,-5.6091616995248,-0.604706365635819));
#15797=CARTESIAN_POINT('Ctrl Pts',(2.8097186803481,-5.6169364463239,-0.49135975117377));
#15798=CARTESIAN_POINT('Ctrl Pts',(2.82707707960445,-5.62471120101895,-0.376449536131305));
#15799=CARTESIAN_POINT('Ctrl Pts',(2.83731951212943,-5.63248595349808,-0.26092697658365));
#15800=CARTESIAN_POINT('Ctrl Pts',(2.84937910293163,-5.64164006149519,-0.12490901472063));
#15801=CARTESIAN_POINT('Ctrl Pts',(2.85157945535316,-5.65079408277546,0.0119261659157435));
#15802=CARTESIAN_POINT('Ctrl Pts',(2.84417579217258,-5.65994807517877,0.148238094356482));
#15803=CARTESIAN_POINT('Ctrl Pts',(2.83664510333784,-5.6692591238723,0.286888745056287));
#15804=CARTESIAN_POINT('Ctrl Pts',(2.81917796946369,-5.6785701426895,0.424999299784865));
#15805=CARTESIAN_POINT('Ctrl Pts',(2.79198999722367,-5.68788119249867,0.561164284972185));
#15806=CARTESIAN_POINT('Ctrl Pts',(2.77607045508886,-5.69333314928484,0.640893813891735));
#15807=CARTESIAN_POINT('Ctrl Pts',(2.75681711012934,-5.69878511669668,0.71995629975189));
#15808=CARTESIAN_POINT('Ctrl Pts',(2.73426515074854,-5.70423710695368,0.798067696028705));
#15809=CARTESIAN_POINT('Ctrl Pts',(2.69986398426108,-5.71255367144159,0.917220231846649));
#15810=CARTESIAN_POINT('Ctrl Pts',(2.65775494410319,-5.7208702511505,1.03425194984188));
#15811=CARTESIAN_POINT('Ctrl Pts',(2.60808881511018,-5.7291868416733,1.14798084834381));
#15812=CARTESIAN_POINT('Ctrl Pts',(2.5731333343602,-5.73504013497034,1.22802429853621));
#15813=CARTESIAN_POINT('Ctrl Pts',(2.53443556790553,-5.74089343362401,1.30643163648447));
#15814=CARTESIAN_POINT('Ctrl Pts',(2.49206304447104,-5.74674673609787,1.38279491692253));
#15815=CARTESIAN_POINT('Ctrl Pts',(2.43196952830668,-5.75504800065133,1.49109476917145));
#15816=CARTESIAN_POINT('Ctrl Pts',(2.36448332309234,-5.76334927288853,1.59528160281069));
#15817=CARTESIAN_POINT('Ctrl Pts',(2.29050189237751,-5.7716505484267,1.69458502869615));
#15818=CARTESIAN_POINT('Ctrl Pts',(2.27761425207795,-5.77309663904876,1.7118837862487));
#15819=CARTESIAN_POINT('Ctrl Pts',(2.26452960469196,-5.77454272977099,1.72903443523847));
#15820=CARTESIAN_POINT('Ctrl Pts',(2.25125281022662,-5.77598882057022,1.74603301441406));
#15821=CARTESIAN_POINT('Ctrl Pts',(2.16812732437095,-5.78504273795906,1.85246044736981));
#15822=CARTESIAN_POINT('Ctrl Pts',(2.07746093396082,-5.79409655590333,1.9529454960784));
#15823=CARTESIAN_POINT('Ctrl Pts',(1.98028264461572,-5.80315034641737,2.04667701103836));
#15824=CARTESIAN_POINT('Ctrl Pts',(1.88228616404374,-5.81228036519205,2.14119769715721));
#15825=CARTESIAN_POINT('Ctrl Pts',(1.77766674968735,-5.82141035607266,2.22885151585887));
#15826=CARTESIAN_POINT('Ctrl Pts',(1.66743971161223,-5.83054039290774,2.30877304976365));
#15827=CARTESIAN_POINT('Ctrl Pts',(1.59822319673337,-5.83627355367733,2.35895937552604));
#15828=CARTESIAN_POINT('Ctrl Pts',(1.5267947663949,-5.84200673256746,2.40609603228708));
#15829=CARTESIAN_POINT('Ctrl Pts',(1.45340037684324,-5.84773994786366,2.44995969872409));
#15830=CARTESIAN_POINT('Ctrl Pts',(1.34833164615637,-5.8559474097365,2.51275332346791));
#15831=CARTESIAN_POINT('Ctrl Pts',(1.23917579451082,-5.86415487372048,2.56886748694508));
#15832=CARTESIAN_POINT('Ctrl Pts',(1.12680042373391,-5.87236233910441,2.61754633616288));
#15833=CARTESIAN_POINT('Ctrl Pts',(1.07216724228544,-5.87635253680033,2.64121237956396));
#15834=CARTESIAN_POINT('Ctrl Pts',(1.01677359388372,-5.88034273482714,2.66312162629128));
#15835=CARTESIAN_POINT('Ctrl Pts',(0.960721486505664,-5.88433293310313,
2.68319105271398));
#15836=CARTESIAN_POINT('Ctrl Pts',(0.845451670024785,-5.8925386803,2.72446334752742));
#15837=CARTESIAN_POINT('Ctrl Pts',(0.727396622634277,-5.90074442855068,
2.75795152729709));
#15838=CARTESIAN_POINT('Ctrl Pts',(0.607702879355788,-5.90895017714448,
2.78366462868508));
#15839=CARTESIAN_POINT('Ctrl Pts',(0.556448060882608,-5.91246401289806,
2.79467539923937));
#15840=CARTESIAN_POINT('Ctrl Pts',(0.504892884501329,-5.91597784871455,
2.8042611070848));
#15841=CARTESIAN_POINT('Ctrl Pts',(0.453127606679704,-5.91949168453815,
2.81242536210152));
#15842=CARTESIAN_POINT('Ctrl Pts',(0.319234225988536,-5.92858038989074,
2.83354260035493));
#15843=CARTESIAN_POINT('Ctrl Pts',(0.183869595833746,-5.93766899938026,
2.8451657633036));
#15844=CARTESIAN_POINT('Ctrl Pts',(0.0483532896092884,-5.94675758765968,
2.8473542009551));
#15845=CARTESIAN_POINT('Ctrl Pts',(-0.0871603316276508,-5.9558459958667,
2.84954259524703));
#15846=CARTESIAN_POINT('Ctrl Pts',(-0.222826888457978,-5.96493438286443,
2.84229661416303));
#15847=CARTESIAN_POINT('Ctrl Pts',(-0.357330541496659,-5.97402282330132,
2.82562460597089));
#15848=CARTESIAN_POINT('Ctrl Pts',(-0.442278735615453,-5.97976279084144,
2.81509510021948));
#15849=CARTESIAN_POINT('Ctrl Pts',(-0.526763083009378,-5.98550277969727,
2.8008047422449));
#15850=CARTESIAN_POINT('Ctrl Pts',(-0.610449379425582,-5.99124280867417,
2.78274520582773));
#15851=CARTESIAN_POINT('Ctrl Pts',(-0.731085633271099,-5.99951722900809,
2.7567118537396));
#15852=CARTESIAN_POINT('Ctrl Pts',(-0.850088999337008,-6.00779164691864,
2.72283472405422));
#15853=CARTESIAN_POINT('Ctrl Pts',(-0.966285437540862,-6.01606605918477,
2.68112815680615));
#15854=CARTESIAN_POINT('Ctrl Pts',(-0.993684309326853,-6.01801714791252,
2.671293837387));
#15855=CARTESIAN_POINT('Ctrl Pts',(-1.0209271484257,-6.01996823632644,2.66102442127421));
#15856=CARTESIAN_POINT('Ctrl Pts',(-1.04799865446575,-6.0219193243843,2.6503205127232));
#15857=CARTESIAN_POINT('Ctrl Pts',(-1.16296636172232,-6.03020523652882,
2.60486298173203));
#15858=CARTESIAN_POINT('Ctrl Pts',(-1.27484199587427,-6.03849114225165,
2.5515654815248));
#15859=CARTESIAN_POINT('Ctrl Pts',(-1.38274512718447,-6.04677703831838,
2.4912081959808));
#15860=CARTESIAN_POINT('Ctrl Pts',(-1.45314261769349,-6.05218287114856,
2.4518302707562));
#15861=CARTESIAN_POINT('Ctrl Pts',(-1.52184967133763,-6.05758869986867,
2.40944842689175));
#15862=CARTESIAN_POINT('Ctrl Pts',(-1.58862902491494,-6.06299452358051,
2.36428881032277));
#15863=CARTESIAN_POINT('Ctrl Pts',(-1.70302589983738,-6.07225501063062,
2.28692778881772));
#15864=CARTESIAN_POINT('Ctrl Pts',(-1.81186251619505,-6.08151542614159,
2.20135783068163));
#15865=CARTESIAN_POINT('Ctrl Pts',(-1.9141178692562,-6.09077583323541,2.10853699469762));
#15866=CARTESIAN_POINT('Ctrl Pts',(-2.01540941019701,-6.09994895597365,
2.01659104539743));
#15867=CARTESIAN_POINT('Ctrl Pts',(-2.11024405254985,-6.10912207045263,
1.91752935253497));
#15868=CARTESIAN_POINT('Ctrl Pts',(-2.19759562695022,-6.11829523802621,
1.81224624033903));
#15869=CARTESIAN_POINT('Ctrl Pts',(-2.24981189452375,-6.12377869468749,
1.74931101341112));
#15870=CARTESIAN_POINT('Ctrl Pts',(-2.29935352499215,-6.12926217032111,
1.68415204005637));
#15871=CARTESIAN_POINT('Ctrl Pts',(-2.34599349219481,-6.13474567803236,
1.6169559696464));
#15872=CARTESIAN_POINT('Ctrl Pts',(-2.41618993206687,-6.14299874385612,
1.51582114475093));
#15873=CARTESIAN_POINT('Ctrl Pts',(-2.47980005198525,-6.15125181256872,
1.41008201180028));
#15874=CARTESIAN_POINT('Ctrl Pts',(-2.5359725440974,-6.1595048717156,1.30051653404565));
#15875=CARTESIAN_POINT('Ctrl Pts',(-2.59396801765886,-6.16802576967752,
1.18739529748593));
#15876=CARTESIAN_POINT('Ctrl Pts',(-2.64403449050075,-6.17654665744279,
1.07019614130459));
#15877=CARTESIAN_POINT('Ctrl Pts',(-2.68601873281737,-6.18506752130453,
0.950178909542243));
#15878=CARTESIAN_POINT('Ctrl Pts',(-2.72121537483224,-6.19221081551329,
0.849564886068879));
#15879=CARTESIAN_POINT('Ctrl Pts',(-2.75073267587082,-6.19935409292271,
0.746971150019362));
#15880=CARTESIAN_POINT('Ctrl Pts',(-2.7745081152172,-6.20649734545702,0.643144978464038));
#15881=CARTESIAN_POINT('Ctrl Pts',(-2.80583618147833,-6.21590975990097,
0.506336857497832));
#15882=CARTESIAN_POINT('Ctrl Pts',(-2.82723626244033,-6.22532213968569,
0.367244546698496));
#15883=CARTESIAN_POINT('Ctrl Pts',(-2.83855637370735,-6.23473452843586,
0.227335517427473));
#15884=CARTESIAN_POINT('Ctrl Pts',(-2.8496594598203,-6.24396646621073,0.0901087743916822));
#15885=CARTESIAN_POINT('Ctrl Pts',(-2.8510653530964,-6.25319841261058,-0.0479049212921638));
#15886=CARTESIAN_POINT('Ctrl Pts',(-2.84258167957677,-6.26243040879888,
-0.185321199119131));
#15887=CARTESIAN_POINT('Ctrl Pts',(-2.83773638421417,-6.267703095002,-0.26380399930707));
#15888=CARTESIAN_POINT('Ctrl Pts',(-2.82966429723861,-6.2729757974457,-0.342091832328108));
#15889=CARTESIAN_POINT('Ctrl Pts',(-2.81832220863144,-6.27824852379865,
-0.419924497124111));
#15890=CARTESIAN_POINT('Ctrl Pts',(-2.80481332035976,-6.28452855507472,
-0.512626362629817));
#15891=CARTESIAN_POINT('Ctrl Pts',(-2.78666789891511,-6.2908085874816,-0.604654818892115));
#15892=CARTESIAN_POINT('Ctrl Pts',(-2.76383203365409,-6.29708861758833,
-0.695508798970515));
#15893=CARTESIAN_POINT('Ctrl Pts',(-2.73172566074844,-6.30591810515803,
-0.823246098653206));
#15894=CARTESIAN_POINT('Ctrl Pts',(-2.69034550062392,-6.31474758818097,
-0.948660552264399));
#15895=CARTESIAN_POINT('Ctrl Pts',(-2.64045788613141,-6.32357705712189,
-1.07060594415041));
#15896=CARTESIAN_POINT('Ctrl Pts',(-2.5906928614993,-6.33238482922731,-1.19225167711871));
#15897=CARTESIAN_POINT('Ctrl Pts',(-2.53246286639955,-6.34119258731979,
-1.31044437710593));
#15898=CARTESIAN_POINT('Ctrl Pts',(-2.46657308311698,-6.35000032193402,
-1.42407257589893));
#15899=CARTESIAN_POINT('',(-1.86074722859424,-6.34999975408592,-1.07430190765501));
#15900=CARTESIAN_POINT('Ctrl Pts',(-1.86074679171387,-6.34999975408563,
-1.07430266108979));
#15901=CARTESIAN_POINT('Ctrl Pts',(-1.8607430428313,-6.37442981441701,-1.07430049667143));
#15902=CARTESIAN_POINT('Ctrl Pts',(-1.86369055307458,-6.398701888929,-1.07600224250384));
#15903=CARTESIAN_POINT('Ctrl Pts',(-1.87454995456356,-6.4464134230453,-1.08227192087675));
#15904=CARTESIAN_POINT('Ctrl Pts',(-1.88253671298855,-6.46974575644526,
-1.08688307800337));
#15905=CARTESIAN_POINT('Ctrl Pts',(-1.91354213791911,-6.53898582858574,
-1.10478406843336));
#15906=CARTESIAN_POINT('Ctrl Pts',(-1.94373429399608,-6.58153621615069,
-1.12221551787182));
#15907=CARTESIAN_POINT('Ctrl Pts',(-2.00822303235105,-6.64385578994547,
-1.15944810832076));
#15908=CARTESIAN_POINT('Ctrl Pts',(-2.04167479775446,-6.66700783322522,
-1.17876149408129));
#15909=CARTESIAN_POINT('Ctrl Pts',(-2.10551567089605,-6.69360737099446,
-1.21562003937489));
#15910=CARTESIAN_POINT('Ctrl Pts',(-2.13510937709143,-6.70025495629181,
-1.23270597361311));
#15911=CARTESIAN_POINT('Ctrl Pts',(-2.19496906237396,-6.69982796752831,
-1.26726597902458));
#15912=CARTESIAN_POINT('Ctrl Pts',(-2.22452519635254,-6.69282040482862,
-1.28433022093333));
#15913=CARTESIAN_POINT('Ctrl Pts',(-2.288485768463,-6.66533843223848,-1.32125787445883));
#15914=CARTESIAN_POINT('Ctrl Pts',(-2.32200562531788,-6.64162093032346,
-1.34061057283719));
#15915=CARTESIAN_POINT('Ctrl Pts',(-2.38620384795508,-6.57824524282073,
-1.37767543395828));
#15916=CARTESIAN_POINT('Ctrl Pts',(-2.41606512644336,-6.53526148665362,
-1.39491585113183));
#15917=CARTESIAN_POINT('Ctrl Pts',(-2.44604492211185,-6.46620259780363,
-1.41222469423128));
#15918=CARTESIAN_POINT('Ctrl Pts',(-2.45357470056292,-6.44352512622915,
-1.41657201384694));
#15919=CARTESIAN_POINT('Ctrl Pts',(-2.46380600196008,-6.39721118892435,
-1.42247905846275));
#15920=CARTESIAN_POINT('Ctrl Pts',(-2.46657490953438,-6.37367868071213,
-1.42407768799611));
#15921=CARTESIAN_POINT('Ctrl Pts',(-2.46657132033207,-6.35000032196148,
-1.42407561576919));
#15922=CARTESIAN_POINT('Ctrl Pts',(2.01902767720344,-2.11666691256093,0.73486875714661));
#15923=CARTESIAN_POINT('Ctrl Pts',(1.98328697402221,-2.126004011307,0.833645723886708));
#15924=CARTESIAN_POINT('Ctrl Pts',(1.94040529944881,-2.13534109246068,0.929939958542491));
#15925=CARTESIAN_POINT('Ctrl Pts',(1.89068523013276,-2.1446781618249,1.02255013903026));
#15926=CARTESIAN_POINT('Ctrl Pts',(1.84649040156668,-2.15297763094347,1.10486883058545));
#15927=CARTESIAN_POINT('Ctrl Pts',(1.79689349372479,-2.16127709074722,1.18427617526517));
#15928=CARTESIAN_POINT('Ctrl Pts',(1.74213944561929,-2.16957654531166,1.25994053526106));
#15929=CARTESIAN_POINT('Ctrl Pts',(1.6892295996948,-2.17759646123489,1.33305640098927));
#15930=CARTESIAN_POINT('Ctrl Pts',(1.63150474578687,-2.18561637226582,1.40267685173721));
#15931=CARTESIAN_POINT('Ctrl Pts',(1.56962782965123,-2.1936362820818,1.46836171795241));
#15932=CARTESIAN_POINT('Ctrl Pts',(1.49433665037739,-2.20339482380342,1.54828637074126));
#15933=CARTESIAN_POINT('Ctrl Pts',(1.4129141324678,-2.2131534514039,1.62237850708974));
#15934=CARTESIAN_POINT('Ctrl Pts',(1.32642445619322,-2.22291210493305,1.68999096418341));
#15935=CARTESIAN_POINT('Ctrl Pts',(1.23875871499644,-2.23280345418495,1.75852279850818));
#15936=CARTESIAN_POINT('Ctrl Pts',(1.1458860079854,-2.24269483007546,1.82039837823104));
#15937=CARTESIAN_POINT('Ctrl Pts',(1.04887678686688,-2.25258617017529,1.87490705154322));
#15938=CARTESIAN_POINT('Ctrl Pts',(0.989966237882138,-2.25859285973281,
1.90800839832475));
#15939=CARTESIAN_POINT('Ctrl Pts',(0.929529589478074,-2.26459953609166,
1.93839225646822));
#15940=CARTESIAN_POINT('Ctrl Pts',(0.867802501469699,-2.27060618527117,
1.96589098130968));
#15941=CARTESIAN_POINT('Ctrl Pts',(0.776313466021059,-2.27950896292428,
2.0066483196677));
#15942=CARTESIAN_POINT('Ctrl Pts',(0.681931515948534,-2.28841172914792,
2.04108740306593));
#15943=CARTESIAN_POINT('Ctrl Pts',(0.585569263820482,-2.29731449308824,
2.06858465183689));
#15944=CARTESIAN_POINT('Ctrl Pts',(0.550019481933898,-2.30059888411561,
2.07872888544187));
#15945=CARTESIAN_POINT('Ctrl Pts',(0.514200436844675,-2.30388327483221,
2.08792876916703));
#15946=CARTESIAN_POINT('Ctrl Pts',(0.478158691722409,-2.30716766569729,
2.09615463779207));
#15947=CARTESIAN_POINT('Ctrl Pts',(0.380459348914482,-2.31607075371241,
2.11845272452356));
#15948=CARTESIAN_POINT('Ctrl Pts',(0.281123326237266,-2.32497384281853,
2.13358987550845));
#15949=CARTESIAN_POINT('Ctrl Pts',(0.181242420447869,-2.33387694216285,
2.14170712218003));
#15950=CARTESIAN_POINT('Ctrl Pts',(0.130015470738463,-2.33844316649537,
2.14587029815183));
#15951=CARTESIAN_POINT('Ctrl Pts',(0.078645281922746,-2.34300939352099,
2.14818777343025));
#15952=CARTESIAN_POINT('Ctrl Pts',(0.0272788198494572,-2.34757562447378,
2.14868386556989));
#15953=CARTESIAN_POINT('Ctrl Pts',(-0.0870156521548496,-2.35773585227095,
2.14978771011898));
#15954=CARTESIAN_POINT('Ctrl Pts',(-0.201396983616965,-2.3678961366145,
2.14188078703598));
#15955=CARTESIAN_POINT('Ctrl Pts',(-0.314478908535946,-2.37805642767878,
2.12517596726398));
#15956=CARTESIAN_POINT('Ctrl Pts',(-0.426117761075774,-2.38808706021975,
2.10868432271012));
#15957=CARTESIAN_POINT('Ctrl Pts',(-0.536491503978643,-2.398117699311,2.08361760213658));
#15958=CARTESIAN_POINT('Ctrl Pts',(-0.64425804797752,-2.4081482970102,2.05013182659052));
#15959=CARTESIAN_POINT('Ctrl Pts',(-0.702980846087058,-2.41361404492927,
2.03188517634113));
#15960=CARTESIAN_POINT('Ctrl Pts',(-0.760929242478707,-2.41907978055806,
2.01113787810776));
#15961=CARTESIAN_POINT('Ctrl Pts',(-0.817882895186075,-2.42454549613965,
1.98790940623174));
#15962=CARTESIAN_POINT('Ctrl Pts',(-0.888083410572842,-2.4312824837172,
1.95927821894472));
#15963=CARTESIAN_POINT('Ctrl Pts',(-0.956747742671155,-2.43801946488298,
1.92688588256022));
#15964=CARTESIAN_POINT('Ctrl Pts',(-1.02341716322646,-2.44475644852306,
1.89079806175955));
#15965=CARTESIAN_POINT('Ctrl Pts',(-1.12079483922406,-2.45459651919776,
1.83808801730262));
#15966=CARTESIAN_POINT('Ctrl Pts',(-1.2139148019473,-2.46443659515107,1.77749245331374));
#15967=CARTESIAN_POINT('Ctrl Pts',(-1.3018249097566,-2.47427670407209,1.71009504716673));
#15968=CARTESIAN_POINT('Ctrl Pts',(-1.38293909340318,-2.48335611964798,
1.64790782301531));
#15969=CARTESIAN_POINT('Ctrl Pts',(-1.45961750775132,-2.49243556329139,
1.57993091908226));
#15970=CARTESIAN_POINT('Ctrl Pts',(-1.53114165351361,-2.50151505675352,
1.50704173381545));
#15971=CARTESIAN_POINT('Ctrl Pts',(-1.63219781099869,-2.51434343395977,
1.40405691789381));
#15972=CARTESIAN_POINT('Ctrl Pts',(-1.72318285274175,-2.52717174276055,
1.29105843264262));
#15973=CARTESIAN_POINT('Ctrl Pts',(-1.80215132297835,-2.54000002688318,
1.17022486064862));
#15974=CARTESIAN_POINT('Ctrl Pts',(-1.87537003053102,-2.5518942725329,1.05818928564172));
#15975=CARTESIAN_POINT('Ctrl Pts',(-1.93825866804043,-2.56378849696735,
0.939416864259108));
#15976=CARTESIAN_POINT('Ctrl Pts',(-1.98921976954583,-2.57568273504094,
0.815636020431718));
#15977=CARTESIAN_POINT('Ctrl Pts',(-1.99322167356137,-2.5766167729189,0.805915683913724));
#15978=CARTESIAN_POINT('Ctrl Pts',(-1.99714999655,-2.57755081088096,0.796164462336127));
#15979=CARTESIAN_POINT('Ctrl Pts',(-2.00100395068832,-2.57848484894402,
0.786383193490234));
#15980=CARTESIAN_POINT('Ctrl Pts',(-2.00629831746431,-2.57976798307355,
0.772946182320367));
#15981=CARTESIAN_POINT('Ctrl Pts',(-2.01145137689601,-2.58105111671826,
0.759454900076632));
#15982=CARTESIAN_POINT('Ctrl Pts',(-2.01646120941697,-2.58233424995876,
0.745911650883031));
#15983=CARTESIAN_POINT('Ctrl Pts',(-2.07587033556421,-2.59755029245722,
0.585308956796785));
#15984=CARTESIAN_POINT('Ctrl Pts',(-2.11513693986626,-2.61276627811604,
0.417402205530998));
#15985=CARTESIAN_POINT('Ctrl Pts',(-2.13438726309228,-2.62798234140889,
0.247239058661555));
#15986=CARTESIAN_POINT('Ctrl Pts',(-2.14597254926331,-2.6371397173955,0.144830972880328));
#15987=CARTESIAN_POINT('Ctrl Pts',(-2.15030844243079,-2.64629712150046,
0.0416048035328496));
#15988=CARTESIAN_POINT('Ctrl Pts',(-2.14742535580896,-2.65545458303564,
-0.0613479590683571));
#15989=CARTESIAN_POINT('Ctrl Pts',(-2.14388349299061,-2.66670449563844,
-0.187825103092371));
#15990=CARTESIAN_POINT('Ctrl Pts',(-2.12943572662261,-2.67795431606019,
-0.314140136072367));
#15991=CARTESIAN_POINT('Ctrl Pts',(-2.10404000415043,-2.68920409851113,
-0.438193946100994));
#15992=CARTESIAN_POINT('Ctrl Pts',(-2.08093266461339,-2.69944017441315,
-0.551069392441806));
#15993=CARTESIAN_POINT('Ctrl Pts',(-2.04876210810997,-2.70967621887905,
-0.662071553421715));
#15994=CARTESIAN_POINT('Ctrl Pts',(-2.00753391608164,-2.71991227274539,
-0.769615212908264));
#15995=CARTESIAN_POINT('Ctrl Pts',(-1.99073561147467,-2.72408292254497,
-0.813433558116374));
#15996=CARTESIAN_POINT('Ctrl Pts',(-1.97243403118461,-2.72825357390515,
-0.856677792790132));
#15997=CARTESIAN_POINT('Ctrl Pts',(-1.9526992126251,-2.73242422958818,-0.899267183121456));
#15998=CARTESIAN_POINT('Ctrl Pts',(-1.90326331720604,-2.74287175904245,
-1.00595398340959));
#15999=CARTESIAN_POINT('Ctrl Pts',(-1.84489228968031,-2.75331932322472,
-1.10841690245437));
#16000=CARTESIAN_POINT('Ctrl Pts',(-1.77867028859895,-2.76376690339706,
-1.20553228931488));
#16001=CARTESIAN_POINT('Ctrl Pts',(-1.71025876617817,-2.77455991559136,
-1.30585863640679));
#16002=CARTESIAN_POINT('Ctrl Pts',(-1.63346781980748,-2.78535294485061,
-1.40047918676907));
#16003=CARTESIAN_POINT('Ctrl Pts',(-1.54944166015184,-2.79614597051608,
-1.48813545871277));
#16004=CARTESIAN_POINT('Ctrl Pts',(-1.51506181712427,-2.80056200630413,
-1.52400058550372));
#16005=CARTESIAN_POINT('Ctrl Pts',(-1.47947021694904,-2.80497804149054,
-1.55869950244843));
#16006=CARTESIAN_POINT('Ctrl Pts',(-1.44274333212728,-2.80939407466028,
-1.5921443698884));
#16007=CARTESIAN_POINT('Ctrl Pts',(-1.36675766648564,-2.8185305756602,-1.66133974344259));
#16008=CARTESIAN_POINT('Ctrl Pts',(-1.28581733678521,-2.82766704559732,
-1.72524726017498));
#16009=CARTESIAN_POINT('Ctrl Pts',(-1.20068636638464,-2.83680349751591,
-1.78296493675049));
#16010=CARTESIAN_POINT('Ctrl Pts',(-1.13642101631696,-2.84370060297778,
-1.82653599758493));
#16011=CARTESIAN_POINT('Ctrl Pts',(-1.06976858867396,-2.85059769817135,
-1.86658003345463));
#16012=CARTESIAN_POINT('Ctrl Pts',(-1.00107121872319,-2.85749478870825,
-1.90272342059117));
#16013=CARTESIAN_POINT('Ctrl Pts',(-0.910271969975343,-2.86661086752968,
-1.95049515335986));
#16014=CARTESIAN_POINT('Ctrl Pts',(-0.815900262721384,-2.8757269382161,
-1.99145060003429));
#16015=CARTESIAN_POINT('Ctrl Pts',(-0.719119978740421,-2.88484301372475,
-2.0254427242301));
#16016=CARTESIAN_POINT('Ctrl Pts',(-0.713739094553147,-2.88534985814116,
-2.02733265135217));
#16017=CARTESIAN_POINT('Ctrl Pts',(-0.708350768133567,-2.88585670257248,
-2.02920106606425));
#16018=CARTESIAN_POINT('Ctrl Pts',(-0.702955200467601,-2.88636354702093,
-2.03104794768616));
#16019=CARTESIAN_POINT('Ctrl Pts',(-0.598216337224688,-2.89620242119662,
-2.06689964923064));
#16020=CARTESIAN_POINT('Ctrl Pts',(-0.490737426444422,-2.90604137804317,
-2.09464568934945));
#16021=CARTESIAN_POINT('Ctrl Pts',(-0.38178492289613,-2.91588035490109,
-2.11417112339656));
#16022=CARTESIAN_POINT('Ctrl Pts',(-0.272214869587739,-2.92577509970926,
-2.13380722885295));
#16023=CARTESIAN_POINT('Ctrl Pts',(-0.161153117653703,-2.93566986475628,
-2.14512948741539));
#16024=CARTESIAN_POINT('Ctrl Pts',(-0.0498742561368832,-2.94556458631102,
-2.14797114567485));
#16025=CARTESIAN_POINT('Ctrl Pts',(0.0167371607961003,-2.95148755689082,
-2.14967215951093));
#16026=CARTESIAN_POINT('Ctrl Pts',(0.0834265370338267,-2.95741051188645,
-2.1483334293431));
#16027=CARTESIAN_POINT('Ctrl Pts',(0.149919701399027,-2.9633334376282,-2.14391022910733));
#16028=CARTESIAN_POINT('Ctrl Pts',(0.251021357348566,-2.97233913928601,
-2.13718483300531));
#16029=CARTESIAN_POINT('Ctrl Pts',(0.351700451929421,-2.98134483501702,
-2.12332085454694));
#16030=CARTESIAN_POINT('Ctrl Pts',(0.45082962216509,-2.99035053533562,-2.10217188848715));
#16031=CARTESIAN_POINT('Ctrl Pts',(0.468209302747445,-2.99192944691721,
-2.09846397613509));
#16032=CARTESIAN_POINT('Ctrl Pts',(0.485541342774309,-2.99350835863981,
-2.09453226464521));
#16033=CARTESIAN_POINT('Ctrl Pts',(0.502819678785445,-2.99508727056008,
-2.09037613140608));
#16034=CARTESIAN_POINT('Ctrl Pts',(0.601517176268586,-3.00410634827552,
-2.06663542225191));
#16035=CARTESIAN_POINT('Ctrl Pts',(0.698460834250939,-3.01312543244114,
-2.0355679225887));
#16036=CARTESIAN_POINT('Ctrl Pts',(0.792702219519714,-3.02214453361833,
-1.99780436319945));
#16037=CARTESIAN_POINT('Ctrl Pts',(0.855948223313822,-3.02819731081006,
-1.97246099400342));
#16038=CARTESIAN_POINT('Ctrl Pts',(0.917977434715979,-3.03425009566351,
-1.94410294380237));
#16039=CARTESIAN_POINT('Ctrl Pts',(0.978509859770852,-3.04030289137092,
-1.91293217178945));
#16040=CARTESIAN_POINT('Ctrl Pts',(1.08348604361805,-3.05079973491213,-1.85887538006963));
#16041=CARTESIAN_POINT('Ctrl Pts',(1.18409430990973,-3.06129660945067,-1.79629832428746));
#16042=CARTESIAN_POINT('Ctrl Pts',(1.2790534874194,-3.07179348120978,-1.72608240750692));
#16043=CARTESIAN_POINT('Ctrl Pts',(1.37191500981002,-3.08205847631034,-1.65741756542116));
#16044=CARTESIAN_POINT('Ctrl Pts',(1.45937529059133,-3.09232346875291,-1.58144670908853));
#16045=CARTESIAN_POINT('Ctrl Pts',(1.54020412886531,-3.1025884269501,-1.49895764141283));
#16046=CARTESIAN_POINT('Ctrl Pts',(1.57874687027005,-3.10748321002225,-1.45962322968509));
#16047=CARTESIAN_POINT('Ctrl Pts',(1.61578118376996,-3.11237798530769,-1.41880624933984));
#16048=CARTESIAN_POINT('Ctrl Pts',(1.65117000973465,-3.11727274938154,-1.37658999295121));
#16049=CARTESIAN_POINT('Ctrl Pts',(1.68828215808527,-3.12240587277567,-1.33231794020028));
#16050=CARTESIAN_POINT('Ctrl Pts',(1.72356791055107,-3.1275389907195,-1.28652619838855));
#16051=CARTESIAN_POINT('Ctrl Pts',(1.75686153146657,-3.13267210796456,-1.23932947979743));
#16052=CARTESIAN_POINT('Ctrl Pts',(1.82542896556432,-3.14324364295352,-1.14212894099627));
#16053=CARTESIAN_POINT('Ctrl Pts',(1.88554372347303,-3.15381517497873,-1.03896801995445));
#16054=CARTESIAN_POINT('Ctrl Pts',(1.93676088325265,-3.16438674554565,-0.931553000126708));
#16055=CARTESIAN_POINT('Ctrl Pts',(1.98497550482512,-3.17433857177936,-0.830435043674648));
#16056=CARTESIAN_POINT('Ctrl Pts',(2.02530530011653,-3.18429043216828,-0.725548422436352));
#16057=CARTESIAN_POINT('Ctrl Pts',(2.05742048141989,-3.19424236133786,-0.618324980965681));
#16058=CARTESIAN_POINT('Ctrl Pts',(2.10378205582973,-3.20860899686635,-0.46353689139319));
#16059=CARTESIAN_POINT('Ctrl Pts',(2.13314836674837,-3.22297550741097,-0.303496650724494));
#16060=CARTESIAN_POINT('Ctrl Pts',(2.14439073836144,-3.23734199227713,-0.14222435195816));
#16061=CARTESIAN_POINT('Ctrl Pts',(2.15297465656259,-3.24831127306355,-0.0190876804117314));
#16062=CARTESIAN_POINT('Ctrl Pts',(2.15099200706442,-3.2592805388799,0.104766880514908));
#16063=CARTESIAN_POINT('Ctrl Pts',(2.13792606424054,-3.27024983392955,0.227534928837607));
#16064=CARTESIAN_POINT('Ctrl Pts',(2.13754399199661,-3.2705705963292,0.231124892787152));
#16065=CARTESIAN_POINT('Ctrl Pts',(2.13715244165655,-3.27089135875384,0.234713926564423));
#16066=CARTESIAN_POINT('Ctrl Pts',(2.13675143309155,-3.27121212120459,0.238301988353448));
#16067=CARTESIAN_POINT('Ctrl Pts',(2.12006352161317,-3.28456060263571,0.387618643257629));
#16068=CARTESIAN_POINT('Ctrl Pts',(2.0870328714325,-3.29790904708474,0.534960049969257));
#16069=CARTESIAN_POINT('Ctrl Pts',(2.03925161079542,-3.31125752348132,0.67736934110968));
#16070=CARTESIAN_POINT('Ctrl Pts',(1.99519448295209,-3.32356560249129,0.8086790692792));
#16071=CARTESIAN_POINT('Ctrl Pts',(1.9385955017089,-3.33587370866286,0.935796635592113));
#16072=CARTESIAN_POINT('Ctrl Pts',(1.87066540489768,-3.34818189603184,1.05641555578819));
#16073=CARTESIAN_POINT('Ctrl Pts',(1.81420327390761,-3.35841221396306,1.1566715776649));
#16074=CARTESIAN_POINT('Ctrl Pts',(1.74981010065795,-3.36864246265313,1.25260873732792));
#16075=CARTESIAN_POINT('Ctrl Pts',(1.67816911246331,-3.37887267710189,1.34277188237266));
#16076=CARTESIAN_POINT('Ctrl Pts',(1.61058024014888,-3.38852425611483,1.42783527208108));
#16077=CARTESIAN_POINT('Ctrl Pts',(1.53654116992183,-3.39817580465036,1.50775846422047));
#16078=CARTESIAN_POINT('Ctrl Pts',(1.45666386721952,-3.40782735209894,1.58133816061886));
#16079=CARTESIAN_POINT('Ctrl Pts',(1.4088717163615,-3.41360206151039,1.62536233058195));
#16080=CARTESIAN_POINT('Ctrl Pts',(1.35899025659116,-3.41937677053273,1.66711606163006));
#16081=CARTESIAN_POINT('Ctrl Pts',(1.30728661284953,-3.42515148546112,1.70648898569144));
#16082=CARTESIAN_POINT('Ctrl Pts',(1.21683432243152,-3.43525398799254,1.7753694533738));
#16083=CARTESIAN_POINT('Ctrl Pts',(1.12087575786482,-3.44535654774423,1.83691690101427));
#16084=CARTESIAN_POINT('Ctrl Pts',(1.02072745743775,-3.45545912633785,1.8906623281449));
#16085=CARTESIAN_POINT('Ctrl Pts',(0.918166962665796,-3.46580503789717,
1.94570227964423));
#16086=CARTESIAN_POINT('Ctrl Pts',(0.811211277586695,-3.47615096921703,
1.99256053397001));
#16087=CARTESIAN_POINT('Ctrl Pts',(0.701240761208127,-3.48649687907851,
2.03069136304103));
#16088=CARTESIAN_POINT('Ctrl Pts',(0.645881247179067,-3.4917050436028,2.04988654586285));
#16089=CARTESIAN_POINT('Ctrl Pts',(0.589757320139156,-3.49691320268921,
2.06686934936848));
#16090=CARTESIAN_POINT('Ctrl Pts',(0.533043472824269,-3.50212135107947,
2.08156541081787));
#16091=CARTESIAN_POINT('Ctrl Pts',(0.435417063012063,-3.51108658361408,
2.10686300189326));
#16092=CARTESIAN_POINT('Ctrl Pts',(0.335946159210999,-3.52005179614604,
2.12540431829036));
#16093=CARTESIAN_POINT('Ctrl Pts',(0.235664798255475,-3.52901699808759,
2.13674789347885));
#16094=CARTESIAN_POINT('Ctrl Pts',(0.174528790778321,-3.5344825865849,2.143663444793));
#16095=CARTESIAN_POINT('Ctrl Pts',(0.11309205425833,-3.53994817114611,2.14790472408161));
#16096=CARTESIAN_POINT('Ctrl Pts',(0.0515913436216816,-3.5454137539039,
2.14938091862104));
#16097=CARTESIAN_POINT('Ctrl Pts',(-0.0491838684249719,-3.55436967092784,
2.15179981453611));
#16098=CARTESIAN_POINT('Ctrl Pts',(-0.150130148628519,-3.56332558310961,
2.14679170622627));
#16099=CARTESIAN_POINT('Ctrl Pts',(-0.250189782466457,-3.5722814998323,
2.13472144525996));
#16100=CARTESIAN_POINT('Ctrl Pts',(-0.275548643893186,-3.57455126479554,
2.13166238874048));
#16101=CARTESIAN_POINT('Ctrl Pts',(-0.300850603572711,-3.57682103005044,
2.12814998377674));
#16102=CARTESIAN_POINT('Ctrl Pts',(-0.326078579897805,-3.57909079574975,
2.12419068029949));
#16103=CARTESIAN_POINT('Ctrl Pts',(-0.436100150534687,-3.58898945682339,
2.10692378653116));
#16104=CARTESIAN_POINT('Ctrl Pts',(-0.544767060932894,-3.59888819610816,
2.08115384518473));
#16105=CARTESIAN_POINT('Ctrl Pts',(-0.65087082904308,-3.60878695149005,
2.04733995937731));
#16106=CARTESIAN_POINT('Ctrl Pts',(-0.756777976652686,-3.61866736352493,
2.01358873395672));
#16107=CARTESIAN_POINT('Ctrl Pts',(-0.860132761081111,-3.62854779159731,
1.97182287975362));
#16108=CARTESIAN_POINT('Ctrl Pts',(-0.959720255848221,-3.63842817393778,
1.92244995048172));
#16109=CARTESIAN_POINT('Ctrl Pts',(-1.01896167856859,-3.64430569810123,
1.89307957038752));
#16110=CARTESIAN_POINT('Ctrl Pts',(-1.07686963551438,-3.65018320608162,
1.86101638968194));
#16111=CARTESIAN_POINT('Ctrl Pts',(-1.13318331580902,-3.65606068487622,
1.82633897465691));
#16112=CARTESIAN_POINT('Ctrl Pts',(-1.21923957158997,-3.66504240682813,
1.77334637176535));
#16113=CARTESIAN_POINT('Ctrl Pts',(-1.30156902058835,-3.67402412301627,
1.71424500772037));
#16114=CARTESIAN_POINT('Ctrl Pts',(-1.37911670791559,-3.68300584746048,
1.64940507645279));
#16115=CARTESIAN_POINT('Ctrl Pts',(-1.45890924686097,-3.69224757499889,
1.58268815788047));
#16116=CARTESIAN_POINT('Ctrl Pts',(-1.53363805546767,-3.70148931127831,
1.50989612163114));
#16117=CARTESIAN_POINT('Ctrl Pts',(-1.60269510276803,-3.71073107157176,
1.43208165791051));
#16118=CARTESIAN_POINT('Ctrl Pts',(-1.65823669784161,-3.71816408714443,
1.36949659811146));
#16119=CARTESIAN_POINT('Ctrl Pts',(-1.71010990385534,-3.72559711825116,
1.30366373156248));
#16120=CARTESIAN_POINT('Ctrl Pts',(-1.75801902860842,-3.7330301728381,1.23514382748167));
#16121=CARTESIAN_POINT('Ctrl Pts',(-1.8292633322244,-3.7440836579626,1.13324981720219));
#16122=CARTESIAN_POINT('Ctrl Pts',(-1.89185880350952,-3.75513714094056,
1.0252604177841));
#16123=CARTESIAN_POINT('Ctrl Pts',(-1.94489966990501,-3.76619061134567,
0.912769160216455));
#16124=CARTESIAN_POINT('Ctrl Pts',(-1.99619038500844,-3.7768793583436,0.803989695708698));
#16125=CARTESIAN_POINT('Ctrl Pts',(-2.03854705782826,-3.7875680935847,0.690999271567748));
#16126=CARTESIAN_POINT('Ctrl Pts',(-2.07110465120936,-3.79825680764115,
0.575226138231553));
#16127=CARTESIAN_POINT('Ctrl Pts',(-2.08302783918947,-3.80217121081797,
0.532827892892737));
#16128=CARTESIAN_POINT('Ctrl Pts',(-2.09363632692981,-3.80608561115359,
0.490056409623361));
#16129=CARTESIAN_POINT('Ctrl Pts',(-2.10288583604143,-3.81000000818494,
0.446981897454489));
#16130=CARTESIAN_POINT('Ctrl Pts',(-2.11122461550155,-3.8135289839576,0.408148608790789));
#16131=CARTESIAN_POINT('Ctrl Pts',(-2.1184553833498,-3.81705795633114,0.369084721521393));
#16132=CARTESIAN_POINT('Ctrl Pts',(-2.12454729965618,-3.82058692703921,
0.329846588021416));
#16133=CARTESIAN_POINT('Ctrl Pts',(-2.14500360606005,-3.83243700876457,
0.198087180763822));
#16134=CARTESIAN_POINT('Ctrl Pts',(-2.15261465112136,-3.84428707171052,
0.0643636641716998));
#16135=CARTESIAN_POINT('Ctrl Pts',(-2.14789672175115,-3.85613718151895,
-0.0689357913238956));
#16136=CARTESIAN_POINT('Ctrl Pts',(-2.14380492206176,-3.86641462991389,
-0.184544701036669));
#16137=CARTESIAN_POINT('Ctrl Pts',(-2.13044038557123,-3.87669211355817,
-0.299833970567715));
#16138=CARTESIAN_POINT('Ctrl Pts',(-2.10816907223884,-3.88696967527413,
-0.413258423524959));
#16139=CARTESIAN_POINT('Ctrl Pts',(-2.07723123887715,-3.90124658328524,
-0.57082016101039));
#16140=CARTESIAN_POINT('Ctrl Pts',(-2.02902853462656,-3.91552334561718,
-0.725184703687629));
#16141=CARTESIAN_POINT('Ctrl Pts',(-1.96432556990801,-3.92980007738602,
-0.872244774834655));
#16142=CARTESIAN_POINT('Ctrl Pts',(-1.92147496314573,-3.93925507873779,
-0.969637735212349));
#16143=CARTESIAN_POINT('Ctrl Pts',(-1.87138840711967,-3.94871006668468,
-1.06382611877347));
#16144=CARTESIAN_POINT('Ctrl Pts',(-1.81429901500113,-3.95816507466421,
-1.15361132284044));
#16145=CARTESIAN_POINT('Ctrl Pts',(-1.80267723264998,-3.96008984633874,
-1.17188904592168));
#16146=CARTESIAN_POINT('Ctrl Pts',(-1.7907652699902,-3.96201461884347,-1.18998428708905));
#16147=CARTESIAN_POINT('Ctrl Pts',(-1.77857117794315,-3.96393939246046,
-1.20789076769297));
#16148=CARTESIAN_POINT('Ctrl Pts',(-1.70631579042681,-3.97534452726184,
-1.31399458338486));
#16149=CARTESIAN_POINT('Ctrl Pts',(-1.62427072861909,-3.98674965866473,
-1.41330788790257));
#16150=CARTESIAN_POINT('Ctrl Pts',(-1.5341310047501,-3.9981548057651,-1.50464901891823));
#16151=CARTESIAN_POINT('Ctrl Pts',(-1.43944800007175,-4.01013480248477,
-1.60059398484525));
#16152=CARTESIAN_POINT('Ctrl Pts',(-1.33583295329178,-4.02211481652421,
-1.68774399261372));
#16153=CARTESIAN_POINT('Ctrl Pts',(-1.22519919519716,-4.03409487001487,
-1.76470626599637));
#16154=CARTESIAN_POINT('Ctrl Pts',(-1.20422281494436,-4.03636631194902,
-1.77929846587639));
#16155=CARTESIAN_POINT('Ctrl Pts',(-1.18299400113378,-4.0386377553014,-1.79352433457489));
#16156=CARTESIAN_POINT('Ctrl Pts',(-1.16152564269842,-4.04090920022285,
-1.80737423761186));
#16157=CARTESIAN_POINT('Ctrl Pts',(-1.07059808751356,-4.05052972775721,
-1.8660344200609));
#16158=CARTESIAN_POINT('Ctrl Pts',(-0.975233856793274,-4.06015020406865,
-1.91803505472432));
#16159=CARTESIAN_POINT('Ctrl Pts',(-0.876496392399245,-4.06977065219613,
-1.96253168699072));
#16160=CARTESIAN_POINT('Ctrl Pts',(-0.787640766643975,-4.07842826705043,
-2.00257500923217));
#16161=CARTESIAN_POINT('Ctrl Pts',(-0.696054456911158,-4.08708585907987,
-2.03654116909533));
#16162=CARTESIAN_POINT('Ctrl Pts',(-0.602532959552935,-4.09574344507526,
-2.06384447888001));
#16163=CARTESIAN_POINT('Ctrl Pts',(-0.522829227727489,-4.10312187604487,
-2.08711373506707));
#16164=CARTESIAN_POINT('Ctrl Pts',(-0.441720492063881,-4.11050030263179,
-2.10554402195451));
#16165=CARTESIAN_POINT('Ctrl Pts',(-0.359817555710095,-4.11787873522977,
-2.11917939160544));
#16166=CARTESIAN_POINT('Ctrl Pts',(-0.24975524404404,-4.12779397617666,
-2.13750279209648));
#16167=CARTESIAN_POINT('Ctrl Pts',(-0.138301660871375,-4.1377092906271,
-2.14716746504687));
#16168=CARTESIAN_POINT('Ctrl Pts',(-0.0267587316605952,-4.14762462594713,
-2.14832538881259));
#16169=CARTESIAN_POINT('Ctrl Pts',(0.0865866807360727,-4.1577001885924,
-2.1495020241016));
#16170=CARTESIAN_POINT('Ctrl Pts',(0.200025723302156,-4.16777577278721,
-2.14189478402756));
#16171=CARTESIAN_POINT('Ctrl Pts',(0.312200346981725,-4.17785132330444,
-2.12561083565466));
#16172=CARTESIAN_POINT('Ctrl Pts',(0.37527943382547,-4.18351710140315,-2.11645389302468));
#16173=CARTESIAN_POINT('Ctrl Pts',(0.437958720801109,-4.18918286885252,
-2.10455231092883));
#16174=CARTESIAN_POINT('Ctrl Pts',(0.499995277943403,-4.19484861583228,
-2.08991802219758));
#16175=CARTESIAN_POINT('Ctrl Pts',(0.597528552581938,-4.20375624839063,
-2.06691013511109));
#16176=CARTESIAN_POINT('Ctrl Pts',(0.69354183936608,-4.21266386910625,-2.03712587047305));
#16177=CARTESIAN_POINT('Ctrl Pts',(0.786932036352475,-4.22157148620242,
-2.00063394444371));
#16178=CARTESIAN_POINT('Ctrl Pts',(0.828036981668865,-4.22549210234257,
-1.98457231621795));
#16179=CARTESIAN_POINT('Ctrl Pts',(0.868633832481699,-4.22941271778155,
-1.96721191752031));
#16180=CARTESIAN_POINT('Ctrl Pts',(0.90862926159499,-4.23333333322053,-1.94856174266362));
#16181=CARTESIAN_POINT('Ctrl Pts',(0.999498644208469,-4.24224094872318,
-1.90618865372738));
#16182=CARTESIAN_POINT('Ctrl Pts',(1.08726144411594,-4.25114856422586,-1.85715487810709));
#16183=CARTESIAN_POINT('Ctrl Pts',(1.17114146098775,-4.26005618795191,-1.80224348783637));
#16184=CARTESIAN_POINT('Ctrl Pts',(1.20806057760194,-4.26397680708578,-1.77807467985973));
#16185=CARTESIAN_POINT('Ctrl Pts',(1.24422788683378,-4.26789742781272,-1.75276780321408));
#16186=CARTESIAN_POINT('Ctrl Pts',(1.27957931791511,-4.27181805083389,-1.72639201418339));
#16187=CARTESIAN_POINT('Ctrl Pts',(1.3702680503316,-4.28187581430195,-1.65872892953555));
#16188=CARTESIAN_POINT('Ctrl Pts',(1.4556635312844,-4.29193364227575,-1.5839813747478));
#16189=CARTESIAN_POINT('Ctrl Pts',(1.53483475315364,-4.3019914798193,-1.5031378542605));
#16190=CARTESIAN_POINT('Ctrl Pts',(1.61323645562851,-4.31195155834294,-1.42308010738455));
#16191=CARTESIAN_POINT('Ctrl Pts',(1.68553520674605,-4.32191164625115,-1.33704328383143));
#16192=CARTESIAN_POINT('Ctrl Pts',(1.75079126578976,-4.33187169019429,-1.24595250185277));
#16193=CARTESIAN_POINT('Ctrl Pts',(1.78773523357387,-4.33751045459343,-1.19438250261951));
#16194=CARTESIAN_POINT('Ctrl Pts',(1.8224212065658,-4.3431492049012,-1.14119209659256));
#16195=CARTESIAN_POINT('Ctrl Pts',(1.85467186346985,-4.34878793143707,-1.08654601653875));
#16196=CARTESIAN_POINT('Ctrl Pts',(1.89687275700405,-4.3561663640351,-1.01504008060466));
#16197=CARTESIAN_POINT('Ctrl Pts',(1.93489002847075,-4.36354479062205,-0.94106042430691));
#16198=CARTESIAN_POINT('Ctrl Pts',(1.96829731533633,-4.37092322159169,-0.865046633882483));
#16199=CARTESIAN_POINT('Ctrl Pts',(2.01185562744538,-4.38054363765073,-0.765935550087445));
#16200=CARTESIAN_POINT('Ctrl Pts',(2.04757471480282,-4.39016406116053,-0.663366408448736));
#16201=CARTESIAN_POINT('Ctrl Pts',(2.07537116398524,-4.39978451516008,-0.558692542423503));
#16202=CARTESIAN_POINT('Ctrl Pts',(2.10038569014399,-4.40844213529894,-0.464494641726159));
#16203=CARTESIAN_POINT('Ctrl Pts',(2.11898467097047,-4.41709978012996,-0.368593231105418));
#16204=CARTESIAN_POINT('Ctrl Pts',(2.13114328281877,-4.42575746644398,-0.271977501874224));
#16205=CARTESIAN_POINT('Ctrl Pts',(2.14799668867745,-4.43775813749655,-0.138055626796601));
#16206=CARTESIAN_POINT('Ctrl Pts',(2.15251713901127,-4.44975876475148,-0.00250973760409071));
#16207=CARTESIAN_POINT('Ctrl Pts',(2.14455054625308,-4.46175937045459,0.132288978275308));
#16208=CARTESIAN_POINT('Ctrl Pts',(2.13696358465177,-4.47318811263152,0.260664145969383));
#16209=CARTESIAN_POINT('Ctrl Pts',(2.11805102970323,-4.48461683526174,0.38836291944513));
#16210=CARTESIAN_POINT('Ctrl Pts',(2.08763593327636,-4.49604555756,0.513320113310582));
#16211=CARTESIAN_POINT('Ctrl Pts',(2.08170861414705,-4.49827279640717,0.537671874526404));
#16212=CARTESIAN_POINT('Ctrl Pts',(2.07534431290476,-4.50050003524172,0.561919428162025));
#16213=CARTESIAN_POINT('Ctrl Pts',(2.06854152661343,-4.50272727420588,0.586047348227131));
#16214=CARTESIAN_POINT('Ctrl Pts',(2.06266257793018,-4.50465204782288,0.606898628544018));
#16215=CARTESIAN_POINT('Ctrl Pts',(2.05645768099176,-4.50657682032761,0.627655118162937));
#16216=CARTESIAN_POINT('Ctrl Pts',(2.04992647049026,-4.50850159200216,0.648306613882153));
#16217=CARTESIAN_POINT('Ctrl Pts',(2.00148207209989,-4.52277833377783,0.80148637829951));
#16218=CARTESIAN_POINT('Ctrl Pts',(1.93508341248904,-4.53705502987922,0.94888612204242));
#16219=CARTESIAN_POINT('Ctrl Pts',(1.85337829407576,-4.55133179542225,1.0872462190929));
#16220=CARTESIAN_POINT('Ctrl Pts',(1.79926773028061,-4.560786819143,1.17887747798519));
#16221=CARTESIAN_POINT('Ctrl Pts',(1.73844424393401,-4.57024187332064,1.26654474140526));
#16222=CARTESIAN_POINT('Ctrl Pts',(1.67167927767296,-4.57969699139271,1.34931380870346));
#16223=CARTESIAN_POINT('Ctrl Pts',(1.58800174988501,-4.59154723186343,1.45304951496815));
#16224=CARTESIAN_POINT('Ctrl Pts',(1.4948126152933,-4.60339736854122,1.54930761273379));
#16225=CARTESIAN_POINT('Ctrl Pts',(1.39356918635948,-4.61524746706802,1.6361369566103));
#16226=CARTESIAN_POINT('Ctrl Pts',(1.30576205774412,-4.62552490567718,1.71144293395264));
#16227=CARTESIAN_POINT('Ctrl Pts',(1.21189793087447,-4.63580231558964,1.77965629821637));
#16228=CARTESIAN_POINT('Ctrl Pts',(1.11295553457626,-4.64607973962771,1.83951895292272));
#16229=CARTESIAN_POINT('Ctrl Pts',(1.07898157212933,-4.64960871033575,1.86007406032922));
#16230=CARTESIAN_POINT('Ctrl Pts',(1.04440905037871,-4.65313768270927,1.87964475352249));
#16231=CARTESIAN_POINT('Ctrl Pts',(1.00930096127305,-4.65666665848189,1.89821843465103));
#16232=CARTESIAN_POINT('Ctrl Pts',(0.903387473349617,-4.66731281275567,
1.95425120094545));
#16233=CARTESIAN_POINT('Ctrl Pts',(0.79273223753515,-4.67795899147102,2.00114538521535));
#16234=CARTESIAN_POINT('Ctrl Pts',(0.678977839651301,-4.68860518531224,
2.03866324799128));
#16235=CARTESIAN_POINT('Ctrl Pts',(0.560988748976523,-4.69964770106407,
2.07757777433349));
#16236=CARTESIAN_POINT('Ctrl Pts',(0.439664173613485,-4.71069023308892,
2.10640542715997));
#16237=CARTESIAN_POINT('Ctrl Pts',(0.316807093101287,-4.72173277099149,
2.12483465690906));
#16238=CARTESIAN_POINT('Ctrl Pts',(0.272660948818338,-4.72570067800559,
2.13145681846568));
#16239=CARTESIAN_POINT('Ctrl Pts',(0.228316755754743,-4.7296685857786,2.13673590012991));
#16240=CARTESIAN_POINT('Ctrl Pts',(0.183857783687548,-4.73363649382823,
2.14065585624885));
#16241=CARTESIAN_POINT('Ctrl Pts',(0.0803066645080147,-4.74287830262938,
2.14978597834517));
#16242=CARTESIAN_POINT('Ctrl Pts',(-0.0240018215168891,-4.75212007513271,
2.15155020610059));
#16243=CARTESIAN_POINT('Ctrl Pts',(-0.127875392181151,-4.7613618266112,
2.14569602543938));
#16244=CARTESIAN_POINT('Ctrl Pts',(-0.211419418846149,-4.76879483509461,
2.14098759169503));
#16245=CARTESIAN_POINT('Ctrl Pts',(-0.294681391670819,-4.77622782997754,
2.13135186522761));
#16246=CARTESIAN_POINT('Ctrl Pts',(-0.37703846110927,-4.78366081920613,
2.11668183700904));
#16247=CARTESIAN_POINT('Ctrl Pts',(-0.476555422722861,-4.79264254365043,
2.09895516648698));
#16248=CARTESIAN_POINT('Ctrl Pts',(-0.574750043958772,-4.80162425983865,
2.07387677410038));
#16249=CARTESIAN_POINT('Ctrl Pts',(-0.670660627882294,-4.81060598179061,
2.04201684610747));
#16250=CARTESIAN_POINT('Ctrl Pts',(-0.775749929386506,-4.82044726152873,
2.00710789819179));
#16251=CARTESIAN_POINT('Ctrl Pts',(-0.878098236304415,-4.83028862309304,
1.96406650285739));
#16252=CARTESIAN_POINT('Ctrl Pts',(-0.976634154300157,-4.8401300054433,
1.91358292833901));
#16253=CARTESIAN_POINT('Ctrl Pts',(-1.07602185190398,-4.85005646021153,
1.8626629558026));
#16254=CARTESIAN_POINT('Ctrl Pts',(-1.17153217597132,-4.85998293612661,
1.80417094133948));
#16255=CARTESIAN_POINT('Ctrl Pts',(-1.26204688891126,-4.86990937055149,
1.73876672548302));
#16256=CARTESIAN_POINT('Ctrl Pts',(-1.31574469854142,-4.8757982229683,1.69996570609074));
#16257=CARTESIAN_POINT('Ctrl Pts',(-1.36768388313526,-4.88168706078284,
1.65873109857275));
#16258=CARTESIAN_POINT('Ctrl Pts',(-1.41762519582607,-4.88757587091708,
1.61519413405892));
#16259=CARTESIAN_POINT('Ctrl Pts',(-1.49357778596525,-4.89653179054423,
1.54898151281495));
#16260=CARTESIAN_POINT('Ctrl Pts',(-1.56493859108713,-4.90548770325245,
1.4774108413));
#16261=CARTESIAN_POINT('Ctrl Pts',(-1.63074006771737,-4.91444361842479,
1.40104746702544));
#16262=CARTESIAN_POINT('Ctrl Pts',(-1.64741662811824,-4.91671338299491,
1.38169412590424));
#16263=CARTESIAN_POINT('Ctrl Pts',(-1.66373626609291,-4.9189831477233,1.36203315505184));
#16264=CARTESIAN_POINT('Ctrl Pts',(-1.679683585303,-4.9212529127627,1.34207416089156));
#16265=CARTESIAN_POINT('Ctrl Pts',(-1.7426728306755,-4.93021810528952,1.26323946999538));
#16266=CARTESIAN_POINT('Ctrl Pts',(-1.79984989259213,-4.93918330266859,
1.17975311248381));
#16267=CARTESIAN_POINT('Ctrl Pts',(-1.85085912733998,-4.94814851431222,
1.09267833389976));
#16268=CARTESIAN_POINT('Ctrl Pts',(-1.88195664065002,-4.95361410872455,
1.03959365032485));
#16269=CARTESIAN_POINT('Ctrl Pts',(-1.91076264313262,-4.95907970843854,
0.985175881641332));
#16270=CARTESIAN_POINT('Ctrl Pts',(-1.93720535570157,-4.96454531558686,
0.929669464527957));
#16271=CARTESIAN_POINT('Ctrl Pts',(-1.98722787292446,-4.97488477781101,
0.82466621651417));
#16272=CARTESIAN_POINT('Ctrl Pts',(-2.02885485523213,-4.98522428219098,
0.715652303906996));
#16273=CARTESIAN_POINT('Ctrl Pts',(-2.06164273452908,-4.99556378758447,
0.604041827372011));
#16274=CARTESIAN_POINT('Ctrl Pts',(-2.09383013986182,-5.00571393630334,
0.494475374016633));
#16275=CARTESIAN_POINT('Ctrl Pts',(-2.1174995142741,-5.01586408599892,0.382405247350599));
#16276=CARTESIAN_POINT('Ctrl Pts',(-2.13218356424474,-5.02601419774826,
0.269158197582545));
#16277=CARTESIAN_POINT('Ctrl Pts',(-2.13965861246377,-5.03118120377906,
0.211508764396793));
#16278=CARTESIAN_POINT('Ctrl Pts',(-2.14480439931278,-5.03634819997643,
0.153554287072376));
#16279=CARTESIAN_POINT('Ctrl Pts',(-2.14755404178161,-5.04151518120572,
0.0954703307314682));
#16280=CARTESIAN_POINT('Ctrl Pts',(-2.1506270936678,-5.04728989613413,0.0305546140104575));
#16281=CARTESIAN_POINT('Ctrl Pts',(-2.15070506431235,-5.0530646051565,-0.0344955820371225));
#16282=CARTESIAN_POINT('Ctrl Pts',(-2.147700795961,-5.05883931456796,-0.0994046846055585));
#16283=CARTESIAN_POINT('Ctrl Pts',(-2.14237858720656,-5.06906949556035,
-0.214394343827251));
#16284=CARTESIAN_POINT('Ctrl Pts',(-2.12738017659775,-5.07929967777391,
-0.328940292500448));
#16285=CARTESIAN_POINT('Ctrl Pts',(-2.1033362720808,-5.08952989620844,-0.441563566451724));
#16286=CARTESIAN_POINT('Ctrl Pts',(-2.08065232489935,-5.09918147898111,
-0.547816708320187));
#16287=CARTESIAN_POINT('Ctrl Pts',(-2.04991806394045,-5.10883309399318,
-0.652357606947935));
#16288=CARTESIAN_POINT('Ctrl Pts',(-2.01170181027345,-5.11848477063517,
-0.753962008416238));
#16289=CARTESIAN_POINT('Ctrl Pts',(-1.95884744412238,-5.13183336455158,
-0.894484318231309));
#16290=CARTESIAN_POINT('Ctrl Pts',(-1.89157103852933,-5.14518186296322,
-1.0297108192664));
#16291=CARTESIAN_POINT('Ctrl Pts',(-1.81113280530604,-5.15853033479973,
-1.15656558152439));
#16292=CARTESIAN_POINT('Ctrl Pts',(-1.73696403125853,-5.17083840960258,
-1.27353312073731));
#16293=CARTESIAN_POINT('Ctrl Pts',(-1.65160455740265,-5.18314646181149,
-1.38338351355141));
#16294=CARTESIAN_POINT('Ctrl Pts',(-1.5560272601333,-5.19545454546225,-1.48366899616924));
#16295=CARTESIAN_POINT('Ctrl Pts',(-1.55353640867527,-5.19577530791299,
-1.48628254821282));
#16296=CARTESIAN_POINT('Ctrl Pts',(-1.55103873300124,-5.19609607033762,
-1.48888947961775));
#16297=CARTESIAN_POINT('Ctrl Pts',(-1.54853425237114,-5.19641683273726,
-1.49148974828301));
#16298=CARTESIAN_POINT('Ctrl Pts',(-1.43636203427787,-5.2107833362814,-1.60795217978105));
#16299=CARTESIAN_POINT('Ctrl Pts',(-1.31054382535276,-5.22514978968107,
-1.7110490773328));
#16300=CARTESIAN_POINT('Ctrl Pts',(-1.17492438881865,-5.23951629224171,
-1.7990638690772));
#16301=CARTESIAN_POINT('Ctrl Pts',(-1.07137451604925,-5.25048558654283,
-1.86626603950257));
#16302=CARTESIAN_POINT('Ctrl Pts',(-0.962109293889222,-5.26145490950394,
-1.9246757010747));
#16303=CARTESIAN_POINT('Ctrl Pts',(-0.84881997766153,-5.27242430532847,
-1.97352716347531));
#16304=CARTESIAN_POINT('Ctrl Pts',(-0.739638176970612,-5.28299598524052,
-2.02060742495879));
#16305=CARTESIAN_POINT('Ctrl Pts',(-0.626517694921249,-5.29356758753868,
-2.0588913811808));
#16306=CARTESIAN_POINT('Ctrl Pts',(-0.511028391401235,-5.3041391537284,
-2.08757984687915));
#16307=CARTESIAN_POINT('Ctrl Pts',(-0.402309495430654,-5.31409097584348,
-2.11458648924993));
#16308=CARTESIAN_POINT('Ctrl Pts',(-0.291492680525968,-5.3240427659596,
-2.1330895639489));
#16309=CARTESIAN_POINT('Ctrl Pts',(-0.179907363169104,-5.33399455870215,
-2.14245964744254));
#16310=CARTESIAN_POINT('Ctrl Pts',(-0.122351852152804,-5.33912767594726,
-2.14729272007715));
#16311=CARTESIAN_POINT('Ctrl Pts',(-0.064592098313675,-5.34426079389113,
-2.14969662974198));
#16312=CARTESIAN_POINT('Ctrl Pts',(-0.00682250918969845,-5.34939391728529,
-2.14972460168947));
#16313=CARTESIAN_POINT('Ctrl Pts',(0.108166914391305,-5.35961131556033,
-2.14978027939405));
#16314=CARTESIAN_POINT('Ctrl Pts',(0.223093636218288,-5.36982876268752,
-2.14042775114858));
#16315=CARTESIAN_POINT('Ctrl Pts',(0.336579295018667,-5.3800462275161,-2.12212138775708));
#16316=CARTESIAN_POINT('Ctrl Pts',(0.45318559989502,-5.39054465376185,-2.10331163317337));
#16317=CARTESIAN_POINT('Ctrl Pts',(0.56827187342757,-5.40104309869592,-2.0750486851374));
#16318=CARTESIAN_POINT('Ctrl Pts',(0.680345080826755,-5.41154152852646,
-2.03777130715719));
#16319=CARTESIAN_POINT('Ctrl Pts',(0.733088785761198,-5.41648228196884,
-2.02022789004132));
#16320=CARTESIAN_POINT('Ctrl Pts',(0.785165052028643,-5.42142303206607,
-2.00068719241862));
#16321=CARTESIAN_POINT('Ctrl Pts',(0.836417046445954,-5.42636377529591,
-1.97919113881164));
#16322=CARTESIAN_POINT('Ctrl Pts',(0.929975508341221,-5.43538290406268,
-1.93995095440218));
#16323=CARTESIAN_POINT('Ctrl Pts',(1.02088553759679,-5.44440200873009,-1.8941483086934));
#16324=CARTESIAN_POINT('Ctrl Pts',(1.10804186902105,-5.4534210998595,-1.84207162275567));
#16325=CARTESIAN_POINT('Ctrl Pts',(1.16653304731231,-5.45947387030836,-1.80712262166504));
#16326=CARTESIAN_POINT('Ctrl Pts',(1.22333370305523,-5.46552663465992,-1.76934898144453));
#16327=CARTESIAN_POINT('Ctrl Pts',(1.27811476006261,-5.47157939610642,-1.72885009767664));
#16328=CARTESIAN_POINT('Ctrl Pts',(1.35962167103746,-5.48058509835686,-1.66859315678911));
#16329=CARTESIAN_POINT('Ctrl Pts',(1.43665565945691,-5.48959079417627,-1.60230184066544));
#16330=CARTESIAN_POINT('Ctrl Pts',(1.50859729941936,-5.49859649407912,-1.53092790094143));
#16331=CARTESIAN_POINT('Ctrl Pts',(1.52121036497895,-5.50017540558772,-1.51841436661758));
#16332=CARTESIAN_POINT('Ctrl Pts',(1.53366699810796,-5.50175431722184,-1.50574468538882));
#16333=CARTESIAN_POINT('Ctrl Pts',(1.54596399104637,-5.50333322903814,-1.49292408572141));
#16334=CARTESIAN_POINT('Ctrl Pts',(1.62278259204332,-5.51319659949247,-1.41283454388587));
#16335=CARTESIAN_POINT('Ctrl Pts',(1.69340018429812,-5.52306005107312,-1.3268320665492));
#16336=CARTESIAN_POINT('Ctrl Pts',(1.75715433925784,-5.53292352065149,-1.2360112097772));
#16337=CARTESIAN_POINT('Ctrl Pts',(1.82098380056235,-5.54279864095037,-1.14508307549899));
#16338=CARTESIAN_POINT('Ctrl Pts',(1.87793435093592,-5.55267377928949,-1.04932402499391));
#16339=CARTESIAN_POINT('Ctrl Pts',(1.92730132974581,-5.56254887231616,-0.949800550051649));
#16340=CARTESIAN_POINT('Ctrl Pts',(1.95688676024052,-5.56846697557897,-0.890156534527914));
#16341=CARTESIAN_POINT('Ctrl Pts',(1.98374769198347,-5.57438506256756,-0.829159971897384));
#16342=CARTESIAN_POINT('Ctrl Pts',(2.0077238870586,-5.5803031196459,-0.767037530372227));
#16343=CARTESIAN_POINT('Ctrl Pts',(2.04465641671103,-5.58941919573078,-0.671345161065114));
#16344=CARTESIAN_POINT('Ctrl Pts',(2.07474324568416,-5.59853526627298,-0.572967749687063));
#16345=CARTESIAN_POINT('Ctrl Pts',(2.09734624033654,-5.60765134422977,-0.472890201266301));
#16346=CARTESIAN_POINT('Ctrl Pts',(2.09860294357747,-5.60815818878241,-0.467325992568302));
#16347=CARTESIAN_POINT('Ctrl Pts',(2.09983652484205,-5.60866503335797,-0.461756533546821));
#16348=CARTESIAN_POINT('Ctrl Pts',(2.10104687894532,-5.60917187795868,-0.456181995147292));
#16349=CARTESIAN_POINT('Ctrl Pts',(2.12286484469567,-5.61830831010622,-0.355694800907008));
#16350=CARTESIAN_POINT('Ctrl Pts',(2.13713093076308,-5.62744475042515,-0.253556656199974));
#16351=CARTESIAN_POINT('Ctrl Pts',(2.14400573572527,-5.63658121195977,-0.150935426994296));
#16352=CARTESIAN_POINT('Ctrl Pts',(2.14919552441782,-5.64347832468125,-0.0734666845532049));
#16353=CARTESIAN_POINT('Ctrl Pts',(2.15017435337808,-5.65037544949297,0.00427695486709702));
#16354=CARTESIAN_POINT('Ctrl Pts',(2.14703088504541,-5.65727259200655,0.0817948386269175));
#16355=CARTESIAN_POINT('Ctrl Pts',(2.1421091136896,-5.66807154235945,0.203165649297445));
#16356=CARTESIAN_POINT('Ctrl Pts',(2.1270823894308,-5.678870504772,0.324156550535808));
#16357=CARTESIAN_POINT('Ctrl Pts',(2.10220051973105,-5.68966945855141,0.443083840827794));
#16358=CARTESIAN_POINT('Ctrl Pts',(2.07802325244665,-5.70016260858665,0.558643359444972));
#16359=CARTESIAN_POINT('Ctrl Pts',(2.04454067222171,-5.71065575047077,0.672255788683429));
#16360=CARTESIAN_POINT('Ctrl Pts',(2.00193664484768,-5.72114886521972,0.782360480362788));
#16361=CARTESIAN_POINT('Ctrl Pts',(1.98421583250369,-5.72551339432251,0.828157666678365));
#16362=CARTESIAN_POINT('Ctrl Pts',(1.96491642180674,-5.7298779187307,0.873347683152784));
#16363=CARTESIAN_POINT('Ctrl Pts',(1.94404948782929,-5.73424243707816,0.917816577806229));
#16364=CARTESIAN_POINT('Ctrl Pts',(1.92410941887966,-5.73841309276118,0.960310258308687));
#16365=CARTESIAN_POINT('Ctrl Pts',(1.90274644225908,-5.74258374412136,1.00212694042875));
#16366=CARTESIAN_POINT('Ctrl Pts',(1.87997738447089,-5.74675439392095,1.04316107770339));
#16367=CARTESIAN_POINT('Ctrl Pts',(1.81856096074179,-5.75800415215426,1.15384505881766));
#16368=CARTESIAN_POINT('Ctrl Pts',(1.74691152655741,-5.76925389903309,1.25883281240855));
#16369=CARTESIAN_POINT('Ctrl Pts',(1.66663796485726,-5.78050368876758,1.35676769980135));
#16370=CARTESIAN_POINT('Ctrl Pts',(1.59359777283289,-5.79073977129635,1.44587777327455));
#16371=CARTESIAN_POINT('Ctrl Pts',(1.51341887038642,-5.80097588930537,1.52914854881905));
#16372=CARTESIAN_POINT('Ctrl Pts',(1.42733367458171,-5.8112120836312,1.60558955286148));
#16373=CARTESIAN_POINT('Ctrl Pts',(1.29936716837099,-5.82642828907195,1.71921987137455));
#16374=CARTESIAN_POINT('Ctrl Pts',(1.15800801595529,-5.84164433594918,1.81806817825947));
#16375=CARTESIAN_POINT('Ctrl Pts',(1.00701260070832,-5.8568603587367,1.89880465791413));
#16376=CARTESIAN_POINT('Ctrl Pts',(0.916140095555648,-5.86601771034833,
1.9473937236909));
#16377=CARTESIAN_POINT('Ctrl Pts',(0.821778444532971,-5.87517505323489,
1.98942241037955));
#16378=CARTESIAN_POINT('Ctrl Pts',(0.724754805610119,-5.88433241670825,
2.02416167134736));
#16379=CARTESIAN_POINT('Ctrl Pts',(0.711159816552476,-5.88561554994876,
2.02902934976029));
#16380=CARTESIAN_POINT('Ctrl Pts',(0.697512572004403,-5.88689868359346,
2.03375390628264));
#16381=CARTESIAN_POINT('Ctrl Pts',(0.683816070900821,-5.888181817723,2.03833533032528));
#16382=CARTESIAN_POINT('Ctrl Pts',(0.55685391361538,-5.9000760581528,2.08080365676094));
#16383=CARTESIAN_POINT('Ctrl Pts',(0.425875493423747,-5.91197028220641,
2.11090507367887));
#16384=CARTESIAN_POINT('Ctrl Pts',(0.293234341046548,-5.9238645247382,2.1287554216344));
#16385=CARTESIAN_POINT('Ctrl Pts',(0.152943045286072,-5.93644477352953,
2.14763529714494));
#16386=CARTESIAN_POINT('Ctrl Pts',(0.0107904063241632,-5.94902504299202,
2.15281057981495));
#16387=CARTESIAN_POINT('Ctrl Pts',(-0.13046881088098,-5.96160537436534,
2.14437022668701));
#16388=CARTESIAN_POINT('Ctrl Pts',(-0.143741864035601,-5.96278745232333,
2.14357715096475));
#16389=CARTESIAN_POINT('Ctrl Pts',(-0.157007040977092,-5.96396953082792,
2.14266382791756));
#16390=CARTESIAN_POINT('Ctrl Pts',(-0.170262062184394,-5.96515160991333,
2.14163030907934));
#16391=CARTESIAN_POINT('Ctrl Pts',(-0.280603216944505,-5.97499180324552,
2.1330268025069));
#16392=CARTESIAN_POINT('Ctrl Pts',(-0.390415974774632,-5.98483193806144,
2.11607611287816));
#16393=CARTESIAN_POINT('Ctrl Pts',(-0.498256555670661,-5.99467204205021,
2.09076297147814));
#16394=CARTESIAN_POINT('Ctrl Pts',(-0.597760479647373,-6.00375145307605,
2.06740667205402));
#16395=CARTESIAN_POINT('Ctrl Pts',(-0.695584319035439,-6.0128308378567,
2.036931429903));
#16396=CARTESIAN_POINT('Ctrl Pts',(-0.790595476208689,-6.02191021814334,
1.99936459740079));
#16397=CARTESIAN_POINT('Ctrl Pts',(-0.861094628275192,-6.02864720178338,
1.97148966232973));
#16398=CARTESIAN_POINT('Ctrl Pts',(-0.930045179462325,-6.03538418294912,
1.93971112476214));
#16399=CARTESIAN_POINT('Ctrl Pts',(-0.9971019628676,-6.04212117052666,1.90433818248478));
#16400=CARTESIAN_POINT('Ctrl Pts',(-1.09648359962445,-6.05210573611818,
1.85191364432608));
#16401=CARTESIAN_POINT('Ctrl Pts',(-1.19165717291185,-6.06209036860843,
1.79162701794501));
#16402=CARTESIAN_POINT('Ctrl Pts',(-1.28166486791139,-6.07207502071128,
1.72441933663095));
#16403=CARTESIAN_POINT('Ctrl Pts',(-1.37337957659669,-6.0822490337103,1.65593704838699));
#16404=CARTESIAN_POINT('Ctrl Pts',(-1.45973172270526,-6.09242306707288,
1.58026789185158));
#16405=CARTESIAN_POINT('Ctrl Pts',(-1.53968310678685,-6.10259707077108,
1.49836039146294));
#16406=CARTESIAN_POINT('Ctrl Pts',(-1.58288860032817,-6.10809507253954,
1.4540978184046));
#16407=CARTESIAN_POINT('Ctrl Pts',(-1.62422435978237,-6.11359306564514,
1.40801273570408));
#16408=CARTESIAN_POINT('Ctrl Pts',(-1.66352182264475,-6.1190910421929,1.36025057756247));
#16409=CARTESIAN_POINT('Ctrl Pts',(-1.72715791131522,-6.12799415444537,
1.28290724012521));
#16410=CARTESIAN_POINT('Ctrl Pts',(-1.78549671967051,-6.13689725176826,
1.20109991786849));
#16411=CARTESIAN_POINT('Ctrl Pts',(-1.83770840508035,-6.14580034330871,
1.11555659088419));
#16412=CARTESIAN_POINT('Ctrl Pts',(-1.86448675036628,-6.15036656363871,
1.0716831030067));
#16413=CARTESIAN_POINT('Ctrl Pts',(-1.88965392423985,-6.15493278244766,
1.0268275077978));
#16414=CARTESIAN_POINT('Ctrl Pts',(-1.91310209470199,-6.15949900096963,
0.981091420437047));
#16415=CARTESIAN_POINT('Ctrl Pts',(-1.95881902987313,-6.16840176447023,
0.891919698309309));
#16416=CARTESIAN_POINT('Ctrl Pts',(-1.99799829735294,-6.17730452687992,
0.799400097384168));
#16417=CARTESIAN_POINT('Ctrl Pts',(-2.03051224263836,-6.1862072973449,0.704628173813906));
#16418=CARTESIAN_POINT('Ctrl Pts',(-2.04250722654103,-6.18949169077914,
0.669665092967466));
#16419=CARTESIAN_POINT('Ctrl Pts',(-2.05359555039938,-6.1927760853097,0.634395617509192));
#16420=CARTESIAN_POINT('Ctrl Pts',(-2.06377255761049,-6.19606048139582,
0.598875080802976));
#16421=CARTESIAN_POINT('Ctrl Pts',(-2.09435351800118,-6.20592978624482,
0.492139170772034));
#16422=CARTESIAN_POINT('Ctrl Pts',(-2.11673115765934,-6.21579916446869,
0.383066308732467));
#16423=CARTESIAN_POINT('Ctrl Pts',(-2.13079348428194,-6.22566855405326,
0.272931722386978));
#16424=CARTESIAN_POINT('Ctrl Pts',(-2.14476120863747,-6.23547154874784,
0.163538050531035));
#16425=CARTESIAN_POINT('Ctrl Pts',(-2.15052521665063,-6.24527455465074,
0.0530955349082416));
#16426=CARTESIAN_POINT('Ctrl Pts',(-2.14792609857233,-6.25507751099098,
-0.0571533180216573));
#16427=CARTESIAN_POINT('Ctrl Pts',(-2.14633944053961,-6.26106182526724,
-0.12445585019977));
#16428=CARTESIAN_POINT('Ctrl Pts',(-2.14163519357573,-6.26704612107341,
-0.191686265490047));
#16429=CARTESIAN_POINT('Ctrl Pts',(-2.13376765524527,-6.2730303845844,-0.258559957831637));
#16430=CARTESIAN_POINT('Ctrl Pts',(-2.12322384350172,-6.28105029440031,
-0.348181843741631));
#16431=CARTESIAN_POINT('Ctrl Pts',(-2.10699630494181,-6.2890702054312,-0.437152810429182));
#16432=CARTESIAN_POINT('Ctrl Pts',(-2.0849960956876,-6.29709012135442,-0.524682076447492));
#16433=CARTESIAN_POINT('Ctrl Pts',(-2.05938271999409,-6.30642717434324,
-0.626586560573035));
#16434=CARTESIAN_POINT('Ctrl Pts',(-2.02594380632947,-6.31576423396336,
-0.726535670824349));
#16435=CARTESIAN_POINT('Ctrl Pts',(-1.98536504097984,-6.32510130601794,
-0.823502176291762));
#16436=CARTESIAN_POINT('Ctrl Pts',(-1.94929567093623,-6.33340077753115,
-0.909693087656475));
#16437=CARTESIAN_POINT('Ctrl Pts',(-1.90758625798322,-6.34170025886873,
-0.993527106597534));
#16438=CARTESIAN_POINT('Ctrl Pts',(-1.86074810235497,-6.34999975410607,
-1.07430040078544));
#16439=CARTESIAN_POINT('Ctrl Pts',(2.812123342995,-2.149914753478,-0.265823920622));
#16440=CARTESIAN_POINT('Ctrl Pts',(2.875955166892,-2.195775864589,0.4094462416164));
#16441=CARTESIAN_POINT('Ctrl Pts',(2.495432588024,-2.287498086811,1.80426843011));
#16442=CARTESIAN_POINT('Ctrl Pts',(0.6849378988389,-2.425081420145,3.00271269346));
#16443=CARTESIAN_POINT('Ctrl Pts',(-1.465969151843,-2.562664753478,2.708385870756));
#16444=CARTESIAN_POINT('Ctrl Pts',(-2.888423491095,-2.700248086811,1.068470223143));
#16445=CARTESIAN_POINT('Ctrl Pts',(-2.875636985226,-2.837831420145,-1.102416714848));
#16446=CARTESIAN_POINT('Ctrl Pts',(-1.433956868336,-2.975414753478,-2.725503141803));
#16447=CARTESIAN_POINT('Ctrl Pts',(0.7202502017102,-3.112998086811,-2.994301979619));
#16448=CARTESIAN_POINT('Ctrl Pts',(2.516567984095,-3.250581420145,-1.775243376929));
#16449=CARTESIAN_POINT('Ctrl Pts',(3.062413387288,-3.388164753478,0.32592613737));
#16450=CARTESIAN_POINT('Ctrl Pts',(2.086558092334,-3.525748086811,2.265144358043));
#16451=CARTESIAN_POINT('Ctrl Pts',(0.07390060109619,-3.663331420145,3.078821578666));
#16452=CARTESIAN_POINT('Ctrl Pts',(-1.975477796517,-3.800914753478,2.3626449362));
#16453=CARTESIAN_POINT('Ctrl Pts',(-3.043249345157,-3.938498086811,0.4724796727349));
#16454=CARTESIAN_POINT('Ctrl Pts',(-2.598842722989,-4.076081420145,-1.652458810098));
#16455=CARTESIAN_POINT('Ctrl Pts',(-0.8630817656259,-4.213664753478,-2.956297259047));
#16456=CARTESIAN_POINT('Ctrl Pts',(1.301540996194,-4.351248086811,-2.791163673665));
#16457=CARTESIAN_POINT('Ctrl Pts',(2.819433352591,-4.488831420145,-1.239112258151));
#16458=CARTESIAN_POINT('Ctrl Pts',(2.93636079082,-4.626414753478,0.928648977838));
#16459=CARTESIAN_POINT('Ctrl Pts',(1.594222544469,-4.763998086811,2.634968329346));
#16460=CARTESIAN_POINT('Ctrl Pts',(-0.5400783736277,-4.901581420145,3.031982679605));
#16461=CARTESIAN_POINT('Ctrl Pts',(-2.406016552425,-5.039164753478,1.922417218389));
#16462=CARTESIAN_POINT('Ctrl Pts',(-3.076414936985,-5.176748086811,-0.142389504376));
#16463=CARTESIAN_POINT('Ctrl Pts',(-2.218155287486,-5.314331420145,-2.136443475091));
#16464=CARTESIAN_POINT('Ctrl Pts',(-0.2577033950294,-5.451914753478,-3.068907366815));
#16465=CARTESIAN_POINT('Ctrl Pts',(1.830800486974,-5.589498086811,-2.476443876835));
#16466=CARTESIAN_POINT('Ctrl Pts',(3.009586244273,-5.727081420145,-0.653444959052));
#16467=CARTESIAN_POINT('Ctrl Pts',(2.69292402247,-5.864664753478,1.494245927945));
#16468=CARTESIAN_POINT('Ctrl Pts',(1.038147154526,-6.002248086811,2.899460185483));
#16469=CARTESIAN_POINT('Ctrl Pts',(-1.132437139127,-6.139831420145,2.863914402526));
#16470=CARTESIAN_POINT('Ctrl Pts',(-2.740480967886,-6.277414753478,1.405413643517));
#16471=CARTESIAN_POINT('Ctrl Pts',(-2.98618295317,-6.414998086811,-0.75185087581));
#16472=CARTESIAN_POINT('Ctrl Pts',(-2.162282365438,-6.506720309034,-1.939922503313));
#16473=CARTESIAN_POINT('Ctrl Pts',(-1.603965104547,-6.552581420145,-2.325079782801));
#16474=CARTESIAN_POINT('Ctrl Pts',(2.828248590073,-2.112003200128,-0.2673482052555));
#16475=CARTESIAN_POINT('Ctrl Pts',(2.89244643772,-2.157864311239,0.4117940838004));
#16476=CARTESIAN_POINT('Ctrl Pts',(2.50974187042,-2.249586533461,1.814614446512));
#16477=CARTESIAN_POINT('Ctrl Pts',(0.6888654622864,-2.387169866795,3.019930815918));
#16478=CARTESIAN_POINT('Ctrl Pts',(-1.474375296204,-2.524753200128,2.72391626755));
#16479=CARTESIAN_POINT('Ctrl Pts',(-2.904986257652,-2.662336533461,1.074597033472));
#16480=CARTESIAN_POINT('Ctrl Pts',(-2.892126431541,-2.799919866795,-1.10873818078));
#16481=CARTESIAN_POINT('Ctrl Pts',(-1.442179448209,-2.937503200128,-2.741131692266));
#16482=CARTESIAN_POINT('Ctrl Pts',(0.7243802525807,-3.075086533461,-3.011471873454));
#16483=CARTESIAN_POINT('Ctrl Pts',(2.53099846085,-3.212669866795,-1.785422958187));
#16484=CARTESIAN_POINT('Ctrl Pts',(3.079973844815,-3.350253200128,0.3277950594809));
#16485=CARTESIAN_POINT('Ctrl Pts',(2.098522811046,-3.487836533461,2.278133124177));
#16486=CARTESIAN_POINT('Ctrl Pts',(0.07432436111898,-3.625419866795,3.096476123865));
#16487=CARTESIAN_POINT('Ctrl Pts',(-1.986805559805,-3.763003200128,2.376192789088));
#16488=CARTESIAN_POINT('Ctrl Pts',(-3.060699912442,-3.900586533461,0.4751889605338));
#16489=CARTESIAN_POINT('Ctrl Pts',(-2.613744978657,-4.038169866795,-1.661934321428));
#16490=CARTESIAN_POINT('Ctrl Pts',(-0.8680308396962,-4.175753200128,-2.973249226626));
#16491=CARTESIAN_POINT('Ctrl Pts',(1.309004278414,-4.313336533461,-2.807168734035));
#16492=CARTESIAN_POINT('Ctrl Pts',(2.835600516647,-4.450919866795,-1.24621756218));
#16493=CARTESIAN_POINT('Ctrl Pts',(2.95319843892,-4.588503200128,0.9339740267032));
#16494=CARTESIAN_POINT('Ctrl Pts',(1.603364118038,-4.726086533461,2.650077736072));
#16495=CARTESIAN_POINT('Ctrl Pts',(-0.5431752851618,-4.863669866795,3.049368641699));
#16496=CARTESIAN_POINT('Ctrl Pts',(-2.419813106363,-5.001253200128,1.933440722287));
#16497=CARTESIAN_POINT('Ctrl Pts',(-3.094055682046,-5.138836533461,-0.1432059927228));
#16498=CARTESIAN_POINT('Ctrl Pts',(-2.230874609403,-5.276419866795,-2.148694246022));
#16499=CARTESIAN_POINT('Ctrl Pts',(-0.2591811150334,-5.414003200128,-3.086505062049));
#16500=CARTESIAN_POINT('Ctrl Pts',(1.841298643208,-5.551586533461,-2.49064427437));
#16501=CARTESIAN_POINT('Ctrl Pts',(3.026843780971,-5.689169866795,-0.6571919360268));
#16502=CARTESIAN_POINT('Ctrl Pts',(2.708365758102,-5.826753200128,1.502814216688));
#16503=CARTESIAN_POINT('Ctrl Pts',(1.044100086645,-5.964336533461,2.916086238533));
#16504=CARTESIAN_POINT('Ctrl Pts',(-1.13893074785,-6.101919866795,2.880336629334));
#16505=CARTESIAN_POINT('Ctrl Pts',(-2.756195404036,-6.239503200128,1.413472551141));
#16506=CARTESIAN_POINT('Ctrl Pts',(-3.003306290972,-6.377086533461,-0.7561621309221));
#16507=CARTESIAN_POINT('Ctrl Pts',(-2.174681301453,-6.468808755684,-1.951046385826));
#16508=CARTESIAN_POINT('Ctrl Pts',(-1.613162543799,-6.514669866795,-2.338412229995));
#16509=CARTESIAN_POINT('Ctrl Pts',(2.877175670666,-1.897001600064,-0.2719731760698));
#16510=CARTESIAN_POINT('Ctrl Pts',(2.942484104304,-1.942862711175,0.4189178855753));
#16511=CARTESIAN_POINT('Ctrl Pts',(2.553158967202,-2.034584933397,1.846006237029));
#16512=CARTESIAN_POINT('Ctrl Pts',(0.700782440203,-2.172168266731,3.072173889222));
#16513=CARTESIAN_POINT('Ctrl Pts',(-1.499881144309,-2.309751600064,2.771038458724));
#16514=CARTESIAN_POINT('Ctrl Pts',(-2.955240855938,-2.447334933397,1.093186946624));
#16515=CARTESIAN_POINT('Ctrl Pts',(-2.942158562201,-2.584918266731,-1.127918716224));
#16516=CARTESIAN_POINT('Ctrl Pts',(-1.467128326585,-2.722501600064,-2.788551700427));
#16517=CARTESIAN_POINT('Ctrl Pts',(0.7369116160266,-2.860084933397,-3.063568611899));
#16518=CARTESIAN_POINT('Ctrl Pts',(2.574783284471,-2.997668266731,-1.816309752677));
#16519=CARTESIAN_POINT('Ctrl Pts',(3.133255628127,-3.135251600064,0.3334657262495));
#16520=CARTESIAN_POINT('Ctrl Pts',(2.134826053647,-3.272834933397,2.317543522314));
#16521=CARTESIAN_POINT('Ctrl Pts',(0.07561012999347,-3.410418266731,3.150043387152));
#16522=CARTESIAN_POINT('Ctrl Pts',(-2.02117615795,-3.548001600064,2.41729956326));
#16523=CARTESIAN_POINT('Ctrl Pts',(-3.113648267764,-3.685584933397,0.4834094573636));
#16524=CARTESIAN_POINT('Ctrl Pts',(-2.658961269639,-3.823168266731,-1.690684833236));
#16525=CARTESIAN_POINT('Ctrl Pts',(-0.8830472760164,-3.960751600064,-3.024684735174));
#16526=CARTESIAN_POINT('Ctrl Pts',(1.331649302635,-4.098334933397,-2.855731145192));
#16527=CARTESIAN_POINT('Ctrl Pts',(2.884654781358,-4.235918266731,-1.267776412174));
#16528=CARTESIAN_POINT('Ctrl Pts',(3.004287080326,-4.373501600064,0.9501312423865));
#16529=CARTESIAN_POINT('Ctrl Pts',(1.631101398876,-4.511084933397,2.695922562946));
#16530=CARTESIAN_POINT('Ctrl Pts',(-0.5525719064653,-4.648668266731,3.102120972527));
#16531=CARTESIAN_POINT('Ctrl Pts',(-2.461674487038,-4.786251600064,1.966888139311));
#16532=CARTESIAN_POINT('Ctrl Pts',(-3.147581073076,-4.923834933397,-0.1456833743688));
#16533=CARTESIAN_POINT('Ctrl Pts',(-2.269467462304,-5.061418266731,-2.185865425709));
#16534=CARTESIAN_POINT('Ctrl Pts',(-0.263664799865,-5.199001600064,-3.139899831678));
#16535=CARTESIAN_POINT('Ctrl Pts',(1.873152055043,-5.336584933397,-2.53373099368));
#16536=CARTESIAN_POINT('Ctrl Pts',(3.079206444611,-5.474168266731,-0.6685609800817));
#16537=CARTESIAN_POINT('Ctrl Pts',(2.755218934369,-5.611751600064,1.528812041827));
#16538=CARTESIAN_POINT('Ctrl Pts',(1.062162420085,-5.749334933397,2.966532860131));
#16539=CARTESIAN_POINT('Ctrl Pts',(-1.15863359741,-5.886918266731,2.930164803169));
#16540=CARTESIAN_POINT('Ctrl Pts',(-2.803876005782,-6.024501600064,1.437924816642));
#16541=CARTESIAN_POINT('Ctrl Pts',(-3.055261769517,-6.162084933397,-0.7692433026587));
#16542=CARTESIAN_POINT('Ctrl Pts',(-2.212302042314,-6.25380715562,-1.984798370744));
#16543=CARTESIAN_POINT('Ctrl Pts',(-1.64106933179,-6.299668266731,-2.378865422135));
#16544=CARTESIAN_POINT('Ctrl Pts',(2.488904911508,-1.507,-0.2352707832963));
#16545=CARTESIAN_POINT('Ctrl Pts',(2.545400065037,-1.552861111111,0.3623855135288));
#16546=CARTESIAN_POINT('Ctrl Pts',(2.208613800721,-1.644583333333,1.596890324375));
#16547=CARTESIAN_POINT('Ctrl Pts',(0.6062128479337,-1.782166666667,2.657588398181));
#16548=CARTESIAN_POINT('Ctrl Pts',(-1.297474319976,-1.91975,2.397090765159));
#16549=CARTESIAN_POINT('Ctrl Pts',(-2.556435311206,-2.057333333333,0.9456629250653));
#16550=CARTESIAN_POINT('Ctrl Pts',(-2.545118454378,-2.194916666667,-0.9757076918219));
#16551=CARTESIAN_POINT('Ctrl Pts',(-1.269141448358,-2.3325,-2.412240619837));
#16552=CARTESIAN_POINT('Ctrl Pts',(0.6374664429341,-2.470083333333,-2.650144390777));
#16553=CARTESIAN_POINT('Ctrl Pts',(2.22731994717,-2.607666666667,-1.571201338294));
#16554=CARTESIAN_POINT('Ctrl Pts',(2.710427243412,-2.74525,0.2884650014053));
#16555=CARTESIAN_POINT('Ctrl Pts',(1.846734318071,-2.882833333333,2.004794324563));
#16556=CARTESIAN_POINT('Ctrl Pts',(0.06540665063282,-3.020416666667,2.724949518265));
#16557=CARTESIAN_POINT('Ctrl Pts',(-1.748421313941,-3.158,2.091088429853));
#16558=CARTESIAN_POINT('Ctrl Pts',(-2.693465868406,-3.295583333333,0.4181740395515));
#16559=CARTESIAN_POINT('Ctrl Pts',(-2.300138233124,-3.433166666667,-1.46252932282));
#16560=CARTESIAN_POINT('Ctrl Pts',(-0.7638813037308,-3.57075,-2.616507837839));
#16561=CARTESIAN_POINT('Ctrl Pts',(1.151945125744,-3.708333333333,-2.470354294206));
#16562=CARTESIAN_POINT('Ctrl Pts',(2.495374726863,-3.845916666667,-1.096691790885));
#16563=CARTESIAN_POINT('Ctrl Pts',(2.598862817463,-3.9835,0.8219123843785));
#16564=CARTESIAN_POINT('Ctrl Pts',(1.41098658807,-4.121083333333,2.332111652539));
#16565=CARTESIAN_POINT('Ctrl Pts',(-0.4780031146462,-4.258666666667,2.683494165244));
#16566=CARTESIAN_POINT('Ctrl Pts',(-2.129475020865,-4.39625,1.701459386102));
#16567=CARTESIAN_POINT('Ctrl Pts',(-2.722819489967,-4.533833333333,-0.1260236104762));
#16568=CARTESIAN_POINT('Ctrl Pts',(-1.963206060383,-4.671416666667,-1.890885999562));
#16569=CARTESIAN_POINT('Ctrl Pts',(-0.2280836106277,-4.809,-2.716174821156));
#16570=CARTESIAN_POINT('Ctrl Pts',(1.620372852909,-4.946583333333,-2.191807604556));
#16571=CARTESIAN_POINT('Ctrl Pts',(2.663671920236,-5.084166666667,-0.5783396279667));
#16572=CARTESIAN_POINT('Ctrl Pts',(2.383406063087,-5.22175,1.322501034076));
#16573=CARTESIAN_POINT('Ctrl Pts',(0.9188251141986,-5.359333333333,2.566203475515));
#16574=CARTESIAN_POINT('Ctrl Pts',(-1.002277643535,-5.496916666667,2.534743236046));
#16575=CARTESIAN_POINT('Ctrl Pts',(-2.425496932009,-5.6345,1.243878910491));
#16576=CARTESIAN_POINT('Ctrl Pts',(-2.642958544944,-5.772083333333,-0.6654350145011));
#16577=CARTESIAN_POINT('Ctrl Pts',(-1.913755032407,-5.863805555556,-1.71695265731));
#16578=CARTESIAN_POINT('Ctrl Pts',(-1.419609362633,-5.909666666667,-2.057840921336));
#16579=CARTESIAN_POINT('Ctrl Pts',(2.10063415235,-1.897001600064,-0.1985683905227));
#16580=CARTESIAN_POINT('Ctrl Pts',(2.14831602577,-1.942862711175,0.3058531414823));
#16581=CARTESIAN_POINT('Ctrl Pts',(1.864068634239,-2.034584933397,1.347774411722));
#16582=CARTESIAN_POINT('Ctrl Pts',(0.5116432556643,-2.172168266731,2.24300290714));
#16583=CARTESIAN_POINT('Ctrl Pts',(-1.095067495643,-2.309751600064,2.023143071595));
#16584=CARTESIAN_POINT('Ctrl Pts',(-2.157629766474,-2.447334933397,0.7981389035067));
#16585=CARTESIAN_POINT('Ctrl Pts',(-2.148078346554,-2.584918266731,-0.8234966674198));
#16586=CARTESIAN_POINT('Ctrl Pts',(-1.071154570131,-2.722501600064,-2.035929539246));
#16587=CARTESIAN_POINT('Ctrl Pts',(0.5380212698415,-2.860084933397,-2.236720169656));
#16588=CARTESIAN_POINT('Ctrl Pts',(1.87985660987,-2.997668266731,-1.326092923911));
#16589=CARTESIAN_POINT('Ctrl Pts',(2.287598858697,-3.135251600064,0.2434642765611));
#16590=CARTESIAN_POINT('Ctrl Pts',(1.558642582494,-3.272834933397,1.692045126811));
#16591=CARTESIAN_POINT('Ctrl Pts',(0.05520317127216,-3.410418266731,2.299855649378));
#16592=CARTESIAN_POINT('Ctrl Pts',(-1.475666469932,-3.548001600064,1.764877296446));
#16593=CARTESIAN_POINT('Ctrl Pts',(-2.273283469047,-3.685584933397,0.3529386217393));
#16594=CARTESIAN_POINT('Ctrl Pts',(-1.941315196609,-3.823168266731,-1.234373812404));
#16595=CARTESIAN_POINT('Ctrl Pts',(-0.6447153314452,-3.960751600064,-2.208330940504));
#16596=CARTESIAN_POINT('Ctrl Pts',(0.972240948854,-4.098334933397,-2.08497744322));
#16597=CARTESIAN_POINT('Ctrl Pts',(2.106094672369,-4.235918266731,-0.9256071695965));
#16598=CARTESIAN_POINT('Ctrl Pts',(2.1934385546,-4.373501600064,0.6936935263705));
#16599=CARTESIAN_POINT('Ctrl Pts',(1.190871777263,-4.511084933397,1.968300742132));
#16600=CARTESIAN_POINT('Ctrl Pts',(-0.4034343228272,-4.648668266731,2.264867357961));
#16601=CARTESIAN_POINT('Ctrl Pts',(-1.797275554691,-4.786251600064,1.436030632892));
#16602=CARTESIAN_POINT('Ctrl Pts',(-2.298057906858,-4.923834933397,-0.1063638465836));
#16603=CARTESIAN_POINT('Ctrl Pts',(-1.656944658461,-5.061418266731,-1.595906573415));
#16604=CARTESIAN_POINT('Ctrl Pts',(-0.1925024213904,-5.199001600064,-2.292449810634));
#16605=CARTESIAN_POINT('Ctrl Pts',(1.367593650775,-5.336584933397,-1.849884215432));
#16606=CARTESIAN_POINT('Ctrl Pts',(2.248137395861,-5.474168266731,-0.4881182758517));
#16607=CARTESIAN_POINT('Ctrl Pts',(2.011593191805,-5.611751600064,1.116190026326));
#16608=CARTESIAN_POINT('Ctrl Pts',(0.775487808312,-5.749334933397,2.165874090898));
#16609=CARTESIAN_POINT('Ctrl Pts',(-0.8459216896603,-5.886918266731,2.139321668922));
#16610=CARTESIAN_POINT('Ctrl Pts',(-2.047117858235,-6.024501600064,1.04983300434));
#16611=CARTESIAN_POINT('Ctrl Pts',(-2.230655320372,-6.162084933397,-0.5616267263435));
#16612=CARTESIAN_POINT('Ctrl Pts',(-1.615208022499,-6.25380715562,-1.449106943876));
#16613=CARTESIAN_POINT('Ctrl Pts',(-1.198149393476,-6.299668266731,-1.736816420537));
#16614=CARTESIAN_POINT('Ctrl Pts',(2.149561232942,-2.112003200128,-0.2031933613371));
#16615=CARTESIAN_POINT('Ctrl Pts',(2.198353692354,-2.157864311239,0.3129769432571));
#16616=CARTESIAN_POINT('Ctrl Pts',(1.907485731021,-2.249586533461,1.379166202239));
#16617=CARTESIAN_POINT('Ctrl Pts',(0.5235602335809,-2.387169866795,2.295245980444));
#16618=CARTESIAN_POINT('Ctrl Pts',(-1.120573343748,-2.524753200128,2.070265262769));
#16619=CARTESIAN_POINT('Ctrl Pts',(-2.20788436476,-2.662336533461,0.8167288166584));
#16620=CARTESIAN_POINT('Ctrl Pts',(-2.198110477214,-2.799919866795,-0.842677202864));
#16621=CARTESIAN_POINT('Ctrl Pts',(-1.096103448508,-2.937503200128,-2.083349547407));
#16622=CARTESIAN_POINT('Ctrl Pts',(0.5505526332874,-3.075086533461,-2.2888169081));
#16623=CARTESIAN_POINT('Ctrl Pts',(1.923641433491,-3.212669866795,-1.3569797184));
#16624=CARTESIAN_POINT('Ctrl Pts',(2.340880642008,-3.350253200128,0.2491349433296));
#16625=CARTESIAN_POINT('Ctrl Pts',(1.594945825095,-3.487836533461,1.731455524949));
#16626=CARTESIAN_POINT('Ctrl Pts',(0.05648894014665,-3.625419866795,2.353422912665));
#16627=CARTESIAN_POINT('Ctrl Pts',(-1.510037068078,-3.763003200128,1.805984070618));
#16628=CARTESIAN_POINT('Ctrl Pts',(-2.326231824369,-3.900586533461,0.3611591185692));
#16629=CARTESIAN_POINT('Ctrl Pts',(-1.986531487591,-4.038169866795,-1.263124324211));
#16630=CARTESIAN_POINT('Ctrl Pts',(-0.6597317677653,-4.175753200128,-2.259766449053));
#16631=CARTESIAN_POINT('Ctrl Pts',(0.9948859730751,-4.313336533461,-2.133539854377));
#16632=CARTESIAN_POINT('Ctrl Pts',(2.15514893708,-4.450919866795,-0.9471660195909));
#16633=CARTESIAN_POINT('Ctrl Pts',(2.244527196006,-4.588503200128,0.7098507420537));
#16634=CARTESIAN_POINT('Ctrl Pts',(1.218609058101,-4.726086533461,2.014145569006));
#16635=CARTESIAN_POINT('Ctrl Pts',(-0.4128309441306,-4.863669866795,2.317619688789));
#16636=CARTESIAN_POINT('Ctrl Pts',(-1.839136935367,-5.001253200128,1.469478049916));
#16637=CARTESIAN_POINT('Ctrl Pts',(-2.351583297887,-5.138836533461,-0.1088412282295));
#16638=CARTESIAN_POINT('Ctrl Pts',(-1.695537511362,-5.276419866795,-1.633077753103));
#16639=CARTESIAN_POINT('Ctrl Pts',(-0.196986106222,-5.414003200128,-2.345844580263));
#16640=CARTESIAN_POINT('Ctrl Pts',(1.39944706261,-5.551586533461,-1.892970934742));
#16641=CARTESIAN_POINT('Ctrl Pts',(2.300500059501,-5.689169866795,-0.4994873199066));
#16642=CARTESIAN_POINT('Ctrl Pts',(2.058446368072,-5.826753200128,1.142187851465));
#16643=CARTESIAN_POINT('Ctrl Pts',(0.7935501417522,-5.964336533461,2.216320712496));
#16644=CARTESIAN_POINT('Ctrl Pts',(-0.8656245392205,-6.101919866795,2.189149842758));
#16645=CARTESIAN_POINT('Ctrl Pts',(-2.094798459981,-6.239503200128,1.07428526984));
#16646=CARTESIAN_POINT('Ctrl Pts',(-2.282610798917,-6.377086533461,-0.5747078980801));
#16647=CARTESIAN_POINT('Ctrl Pts',(-1.652828763361,-6.468808755684,-1.482858928795));
#16648=CARTESIAN_POINT('Ctrl Pts',(-1.226056181467,-6.514669866795,-1.777269612677));
#16649=CARTESIAN_POINT('Ctrl Pts',(2.16568648002,-2.149914753478,-0.2047176459706));
#16650=CARTESIAN_POINT('Ctrl Pts',(2.214844963183,-2.195775864589,0.3153247854411));
#16651=CARTESIAN_POINT('Ctrl Pts',(1.921795013418,-2.287498086811,1.389512218641));
#16652=CARTESIAN_POINT('Ctrl Pts',(0.5274877970284,-2.425081420145,2.312464102902));
#16653=CARTESIAN_POINT('Ctrl Pts',(-1.128979488109,-2.562664753478,2.085795659563));
#16654=CARTESIAN_POINT('Ctrl Pts',(-2.224447131318,-2.700248086811,0.8228556269872));
#16655=CARTESIAN_POINT('Ctrl Pts',(-2.214599923529,-2.837831420145,-0.8489986687962));
#16656=CARTESIAN_POINT('Ctrl Pts',(-1.104326028381,-2.975414753478,-2.09897809787));
#16657=CARTESIAN_POINT('Ctrl Pts',(0.5546826841579,-3.112998086811,-2.305986801935));
#16658=CARTESIAN_POINT('Ctrl Pts',(1.938071910246,-3.250581420145,-1.367159299658));
#16659=CARTESIAN_POINT('Ctrl Pts',(2.358441099535,-3.388164753478,0.2510038654405));
#16660=CARTESIAN_POINT('Ctrl Pts',(1.606910543807,-3.525748086811,1.744444291083));
#16661=CARTESIAN_POINT('Ctrl Pts',(0.05691270016944,-3.663331420145,2.371077457865));
#16662=CARTESIAN_POINT('Ctrl Pts',(-1.521364831366,-3.800914753478,1.819531923506));
#16663=CARTESIAN_POINT('Ctrl Pts',(-2.343682391654,-3.938498086811,0.3638684063681));
#16664=CARTESIAN_POINT('Ctrl Pts',(-2.001433743259,-4.076081420145,-1.272599835542));
#16665=CARTESIAN_POINT('Ctrl Pts',(-0.6646808418357,-4.213664753478,-2.276718416632));
#16666=CARTESIAN_POINT('Ctrl Pts',(1.002349255295,-4.351248086811,-2.149544914748));
#16667=CARTESIAN_POINT('Ctrl Pts',(2.171316101136,-4.488831420145,-0.9542713236204));
#16668=CARTESIAN_POINT('Ctrl Pts',(2.261364844106,-4.626414753478,0.715175790919));
#16669=CARTESIAN_POINT('Ctrl Pts',(1.227750631671,-4.763998086811,2.029254975732));
#16670=CARTESIAN_POINT('Ctrl Pts',(-0.4159278556647,-4.901581420145,2.335005650883));
#16671=CARTESIAN_POINT('Ctrl Pts',(-1.852933489305,-5.039164753478,1.480501553815));
#16672=CARTESIAN_POINT('Ctrl Pts',(-2.369224042948,-5.176748086811,-0.1096577165763));
#16673=CARTESIAN_POINT('Ctrl Pts',(-1.708256833279,-5.314331420145,-1.645328524034));
#16674=CARTESIAN_POINT('Ctrl Pts',(-0.198463826226,-5.451914753478,-2.363442275497));
#16675=CARTESIAN_POINT('Ctrl Pts',(1.409945218843,-5.589498086811,-1.907171332278));
#16676=CARTESIAN_POINT('Ctrl Pts',(2.317757596199,-5.727081420145,-0.5032342968815));
#16677=CARTESIAN_POINT('Ctrl Pts',(2.073888103704,-5.864664753478,1.150756140208));
#16678=CARTESIAN_POINT('Ctrl Pts',(0.7995030738709,-6.002248086811,2.232946765546));
#16679=CARTESIAN_POINT('Ctrl Pts',(-0.872118147943,-6.139831420145,2.205572069566));
#16680=CARTESIAN_POINT('Ctrl Pts',(-2.110512896131,-6.277414753478,1.082344177464));
#16681=CARTESIAN_POINT('Ctrl Pts',(-2.299734136718,-6.414998086811,-0.5790191531922));
#16682=CARTESIAN_POINT('Ctrl Pts',(-1.665227699375,-6.506720309034,-1.493982811308));
#16683=CARTESIAN_POINT('Ctrl Pts',(-1.235253620718,-6.552581420145,-1.790602059871));
#16684=CARTESIAN_POINT('Ctrl Pts',(-2.46657132033207,-6.35000032196148,
-1.42407561576919));
#16685=CARTESIAN_POINT('Ctrl Pts',(-2.46656773371528,-6.32633902069027,
-1.42407354503503));
#16686=CARTESIAN_POINT('Ctrl Pts',(-2.46379616437334,-6.30282232723362,
-1.42247337872942));
#16687=CARTESIAN_POINT('Ctrl Pts',(-2.45356483291024,-6.25653765529766,
-1.41656631675503));
#16688=CARTESIAN_POINT('Ctrl Pts',(-2.44603863170313,-6.2338753697584,-1.41222106246213));
#16689=CARTESIAN_POINT('Ctrl Pts',(-2.41606465188457,-6.16483033080454,
-1.39491557714521));
#16690=CARTESIAN_POINT('Ctrl Pts',(-2.38620330258456,-6.12184666366958,
-1.37767511908847));
#16691=CARTESIAN_POINT('Ctrl Pts',(-2.32200501666487,-6.0584711962758,-1.34061022143123));
#16692=CARTESIAN_POINT('Ctrl Pts',(-2.28848517345059,-6.0347538130208,-1.32125753092827));
#16693=CARTESIAN_POINT('Ctrl Pts',(-2.2245246425145,-6.00727203284357,-1.2843299011748));
#16694=CARTESIAN_POINT('Ctrl Pts',(-2.19496853427892,-6.00026455306915,
-1.26726567412879));
#16695=CARTESIAN_POINT('Ctrl Pts',(-2.13510893685025,-5.999837714383,-1.23270571943976));
#16696=CARTESIAN_POINT('Ctrl Pts',(-2.10551526912305,-6.00648534402824,
-1.21561980741115));
#16697=CARTESIAN_POINT('Ctrl Pts',(-2.04167439680108,-6.03308499838888,
-1.17876126259076));
#16698=CARTESIAN_POINT('Ctrl Pts',(-2.00822262138601,-6.0562371212313,-1.15944787105));
#16699=CARTESIAN_POINT('Ctrl Pts',(-1.94373392235482,-6.11855684463581,
-1.12221530330465));
#16700=CARTESIAN_POINT('Ctrl Pts',(-1.91354181190603,-6.16110729445364,
-1.10478388020964));
#16701=CARTESIAN_POINT('Ctrl Pts',(-1.88254279196225,-6.23033336303122,
-1.08688658770048));
#16702=CARTESIAN_POINT('Ctrl Pts',(-1.87455993512035,-6.25365009437143,
-1.08227768315391));
#16703=CARTESIAN_POINT('Ctrl Pts',(-1.863700740893,-6.30133148665094,-1.07600812444357));
#16704=CARTESIAN_POINT('Ctrl Pts',(-1.86075053790222,-6.32558725065952,
-1.07430482395264));
#16705=CARTESIAN_POINT('Ctrl Pts',(-1.86074679171387,-6.34999975408563,
-1.07430266108979));
#16706=CARTESIAN_POINT('Origin',(-2.165063509461,-6.35,-1.25));
#17083=UNCERTAINTY_MEASURE_WITH_UNIT(LENGTH_MEASURE(0.01),#17114,
'DISTANCE_ACCURACY_VALUE',
'Maximum model space distance between geometric entities at asserted c
onnectivities');
#17090=UNCERTAINTY_MEASURE_WITH_UNIT(LENGTH_MEASURE(0.01),#17114,
'DISTANCE_ACCURACY_VALUE',
'Maximum model space distance between geometric entities at asserted c
onnectivities');
#17106=(
GEOMETRIC_REPRESENTATION_CONTEXT(3)
GLOBAL_UNCERTAINTY_ASSIGNED_CONTEXT((#17083))
GLOBAL_UNIT_ASSIGNED_CONTEXT((#17114,#17116,#17117))
REPRESENTATION_CONTEXT('','3D')
);
#17113=(
GEOMETRIC_REPRESENTATION_CONTEXT(3)
GLOBAL_UNCERTAINTY_ASSIGNED_CONTEXT((#17090))
GLOBAL_UNIT_ASSIGNED_CONTEXT((#17114,#17116,#17117))
REPRESENTATION_CONTEXT('','3D')
);
#17114=(
LENGTH_UNIT()
NAMED_UNIT(*)
SI_UNIT(.MILLI.,.METRE.)
);
#17116=(
NAMED_UNIT(*)
PLANE_ANGLE_UNIT()
SI_UNIT($,.RADIAN.)
);
#17117=(
NAMED_UNIT(*)
SI_UNIT($,.STERADIAN.)
SOLID_ANGLE_UNIT()
);
#17133=SHAPE_DEFINITION_REPRESENTATION(#17164,#17199);
#17164=PRODUCT_DEFINITION_SHAPE('',$,#17222);
#17199=SHAPE_REPRESENTATION('',(#6815),#17106);
#17206=PRODUCT_DEFINITION_CONTEXT('part definition',#17274,'design');
#17222=PRODUCT_DEFINITION('PRESSURESPRING','PRESSURESPRING',#17244,#17206);
#17244=PRODUCT_DEFINITION_FORMATION('',$,#17291);
#17274=APPLICATION_CONTEXT(
'Core Data for Automotive Mechanical Design Process');
#17275=PRODUCT_CONTEXT('part definition',#17274,'mechanical');
#17291=PRODUCT('PRESSURESPRING','PRESSURESPRING','NOT SPECIFIED',(#17275));
#17298=PRESENTATION_STYLE_ASSIGNMENT((#17299));
#17299=SURFACE_STYLE_USAGE(.BOTH.,#17300);
#17300=SURFACE_SIDE_STYLE('',(#17301));
#17301=SURFACE_STYLE_FILL_AREA(#17302);
#17302=FILL_AREA_STYLE('Steel - Satin',(#17303));
#17303=FILL_AREA_STYLE_COLOUR('Steel - Satin',#17304);
#17304=COLOUR_RGB('Steel - Satin', 0.09019608, 0.27058824, 0.51372549);
ENDSEC;
END-ISO-10303-21;
